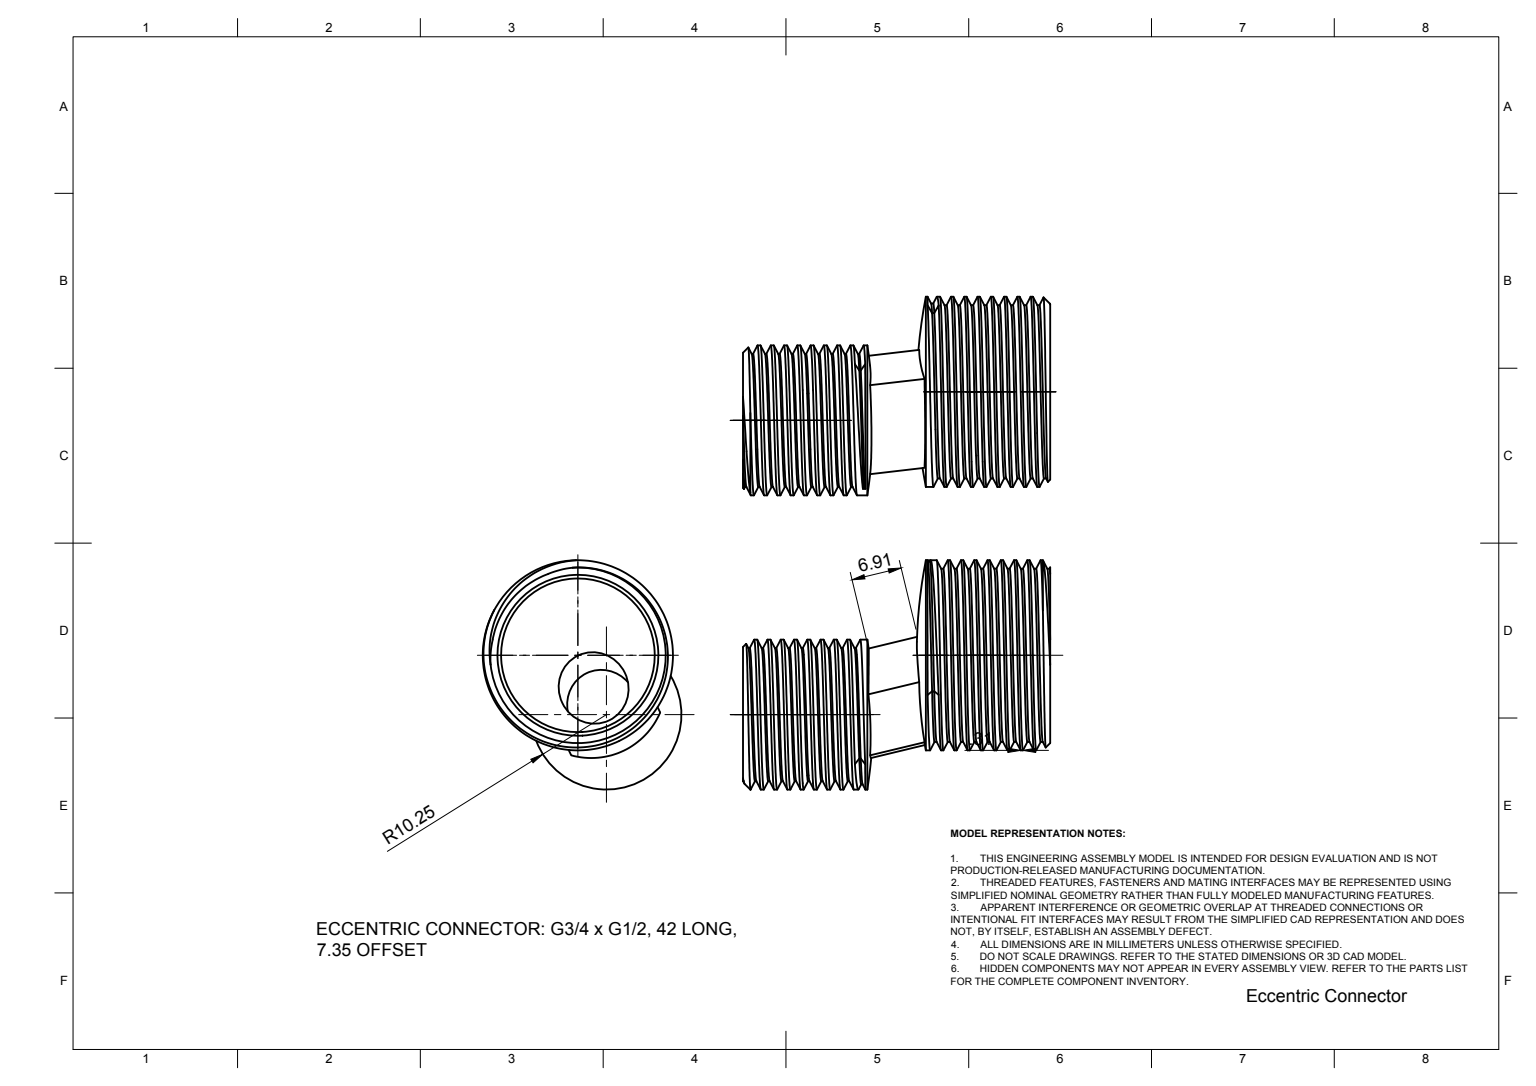
ISO-10303-21;
HEADER;
/* Generated by software containing ST-Developer
 * from STEP Tools, Inc. (www.steptools.com) 
 */

FILE_DESCRIPTION(
/* description */ ('STEP AP214'),
/* implementation_level */ '2;1');

FILE_NAME(
/* name */ 'Eccentric Connector.step',
/* time_stamp */ '2026-10-05T23:18:41-07:00',
/* author */ (''),
/* organization */ (''),
/* preprocessor_version */ 'ST-DEVELOPER v20.2',
/* originating_system */ 'Autodesk Translation Framework v15.15.0.0',
/* authorisation */ '');

FILE_SCHEMA (('AUTOMOTIVE_DESIGN { 1 0 10303 214 3 1 1 }'));
ENDSEC;

DATA;
#10=MECHANICAL_DESIGN_GEOMETRIC_PRESENTATION_REPRESENTATION('',(#112),#221662);
#73=MANIFOLD_SOLID_BREP('Body1',#79335);
#86=SHAPE_REPRESENTATION_RELATIONSHIP('SRR','None',#221721,#99);
#99=ADVANCED_BREP_SHAPE_REPRESENTATION('',(#73),#221661);
#112=STYLED_ITEM('',(#221783),#73);
#226=B_SPLINE_SURFACE_WITH_KNOTS('',3,3,((#217794,#217795,#217796,#217797,
#217798,#217799,#217800),(#217801,#217802,#217803,#217804,#217805,#217806,
#217807),(#217808,#217809,#217810,#217811,#217812,#217813,#217814),(#217815,
#217816,#217817,#217818,#217819,#217820,#217821)),.UNSPECIFIED.,.F.,.F.,
 .F.,(4,4),(4,1,1,1,4),(0.,1.),(0.,0.25,0.5,0.75,1.),.UNSPECIFIED.);
#227=B_SPLINE_SURFACE_WITH_KNOTS('',3,3,((#217858,#217859,#217860,#217861,
#217862,#217863,#217864,#217865,#217866,#217867,#217868,#217869,#217870,
#217871,#217872,#217873,#217874,#217875,#217876,#217877,#217878,#217879,
#217880,#217881,#217882,#217883,#217884,#217885,#217886,#217887,#217888,
#217889,#217890,#217891,#217892,#217893,#217894,#217895,#217896,#217897,
#217898,#217899,#217900,#217901,#217902,#217903,#217904,#217905,#217906,
#217907,#217908,#217909,#217910,#217911,#217912,#217913,#217914,#217915,
#217916,#217917,#217918,#217919,#217920,#217921,#217922,#217923,#217924),
(#217925,#217926,#217927,#217928,#217929,#217930,#217931,#217932,#217933,
#217934,#217935,#217936,#217937,#217938,#217939,#217940,#217941,#217942,
#217943,#217944,#217945,#217946,#217947,#217948,#217949,#217950,#217951,
#217952,#217953,#217954,#217955,#217956,#217957,#217958,#217959,#217960,
#217961,#217962,#217963,#217964,#217965,#217966,#217967,#217968,#217969,
#217970,#217971,#217972,#217973,#217974,#217975,#217976,#217977,#217978,
#217979,#217980,#217981,#217982,#217983,#217984,#217985,#217986,#217987,
#217988,#217989,#217990,#217991),(#217992,#217993,#217994,#217995,#217996,
#217997,#217998,#217999,#218000,#218001,#218002,#218003,#218004,#218005,
#218006,#218007,#218008,#218009,#218010,#218011,#218012,#218013,#218014,
#218015,#218016,#218017,#218018,#218019,#218020,#218021,#218022,#218023,
#218024,#218025,#218026,#218027,#218028,#218029,#218030,#218031,#218032,
#218033,#218034,#218035,#218036,#218037,#218038,#218039,#218040,#218041,
#218042,#218043,#218044,#218045,#218046,#218047,#218048,#218049,#218050,
#218051,#218052,#218053,#218054,#218055,#218056,#218057,#218058),(#218059,
#218060,#218061,#218062,#218063,#218064,#218065,#218066,#218067,#218068,
#218069,#218070,#218071,#218072,#218073,#218074,#218075,#218076,#218077,
#218078,#218079,#218080,#218081,#218082,#218083,#218084,#218085,#218086,
#218087,#218088,#218089,#218090,#218091,#218092,#218093,#218094,#218095,
#218096,#218097,#218098,#218099,#218100,#218101,#218102,#218103,#218104,
#218105,#218106,#218107,#218108,#218109,#218110,#218111,#218112,#218113,
#218114,#218115,#218116,#218117,#218118,#218119,#218120,#218121,#218122,
#218123,#218124,#218125)),.UNSPECIFIED.,.F.,.F.,.F.,(4,4),(4,1,1,1,1,1,
1,1,1,1,1,1,1,1,1,1,1,1,1,1,1,1,1,1,1,1,1,1,1,1,1,1,1,1,1,1,1,1,1,1,1,1,
1,1,1,1,1,1,1,1,1,1,1,1,1,1,1,1,1,1,1,1,1,1,4),(0.,1.),(0.,0.0156250000000022,
0.0312500000000006,0.0468750000000009,0.0625000000000012,0.0781250000000015,
0.0937500000000018,0.109375000000002,0.124999999999983,0.140624999999983,
0.156249999999984,0.171874999999984,0.187499999999984,0.203124999999984,
0.218749999999985,0.234374999999986,0.249999999999986,0.265624999999986,
0.281249999999986,0.296874999999986,0.312499999999987,0.328124999999987,
0.343749999999987,0.359374999999987,0.374999999999988,0.390624999999988,
0.406249999999988,0.421874999999989,0.437499999999989,0.45312499999999,
0.46874999999999,0.48437499999999,0.49999999999999,0.515624999999991,0.531249999999991,
0.546874999999991,0.562499999999992,0.578124999999992,0.593749999999992,
0.609374999999993,0.624999999999993,0.640624999999993,0.65625,0.671875,
0.6875,0.703125,0.71875,0.734375,0.75,0.765625,0.78125,0.796875,0.8125,
0.828125,0.84375,0.859375,0.875,0.890625,0.90625,0.921875,0.9375,0.953125,
0.96875,0.984375,1.),.UNSPECIFIED.);
#228=B_SPLINE_SURFACE_WITH_KNOTS('',3,3,((#218167,#218168,#218169,#218170,
#218171,#218172,#218173,#218174,#218175,#218176,#218177,#218178,#218179,
#218180,#218181,#218182,#218183,#218184,#218185,#218186,#218187,#218188,
#218189,#218190,#218191,#218192,#218193,#218194,#218195,#218196,#218197,
#218198,#218199,#218200,#218201,#218202,#218203,#218204,#218205,#218206,
#218207,#218208,#218209,#218210,#218211,#218212,#218213,#218214,#218215,
#218216,#218217,#218218,#218219,#218220,#218221,#218222,#218223,#218224,
#218225,#218226,#218227,#218228,#218229,#218230,#218231,#218232,#218233),
(#218234,#218235,#218236,#218237,#218238,#218239,#218240,#218241,#218242,
#218243,#218244,#218245,#218246,#218247,#218248,#218249,#218250,#218251,
#218252,#218253,#218254,#218255,#218256,#218257,#218258,#218259,#218260,
#218261,#218262,#218263,#218264,#218265,#218266,#218267,#218268,#218269,
#218270,#218271,#218272,#218273,#218274,#218275,#218276,#218277,#218278,
#218279,#218280,#218281,#218282,#218283,#218284,#218285,#218286,#218287,
#218288,#218289,#218290,#218291,#218292,#218293,#218294,#218295,#218296,
#218297,#218298,#218299,#218300),(#218301,#218302,#218303,#218304,#218305,
#218306,#218307,#218308,#218309,#218310,#218311,#218312,#218313,#218314,
#218315,#218316,#218317,#218318,#218319,#218320,#218321,#218322,#218323,
#218324,#218325,#218326,#218327,#218328,#218329,#218330,#218331,#218332,
#218333,#218334,#218335,#218336,#218337,#218338,#218339,#218340,#218341,
#218342,#218343,#218344,#218345,#218346,#218347,#218348,#218349,#218350,
#218351,#218352,#218353,#218354,#218355,#218356,#218357,#218358,#218359,
#218360,#218361,#218362,#218363,#218364,#218365,#218366,#218367),(#218368,
#218369,#218370,#218371,#218372,#218373,#218374,#218375,#218376,#218377,
#218378,#218379,#218380,#218381,#218382,#218383,#218384,#218385,#218386,
#218387,#218388,#218389,#218390,#218391,#218392,#218393,#218394,#218395,
#218396,#218397,#218398,#218399,#218400,#218401,#218402,#218403,#218404,
#218405,#218406,#218407,#218408,#218409,#218410,#218411,#218412,#218413,
#218414,#218415,#218416,#218417,#218418,#218419,#218420,#218421,#218422,
#218423,#218424,#218425,#218426,#218427,#218428,#218429,#218430,#218431,
#218432,#218433,#218434)),.UNSPECIFIED.,.F.,.F.,.F.,(4,4),(4,1,1,1,1,1,
1,1,1,1,1,1,1,1,1,1,1,1,1,1,1,1,1,1,1,1,1,1,1,1,1,1,1,1,1,1,1,1,1,1,1,1,
1,1,1,1,1,1,1,1,1,1,1,1,1,1,1,1,1,1,1,1,1,1,4),(0.,1.),(0.,0.0156250000000031,
0.03125,0.046875,0.0625,0.078125,0.09375,0.109375,0.124999999999992,0.140624999999992,
0.156249999999992,0.171874999999992,0.187499999999992,0.203124999999992,
0.218749999999993,0.234374999999993,0.249999999999993,0.265624999999993,
0.281249999999993,0.296874999999993,0.312499999999993,0.328124999999993,
0.343749999999994,0.359374999999994,0.374999999999994,0.390624999999994,
0.406249999999994,0.421874999999994,0.437499999999994,0.453125,0.46875,
0.484375,0.5,0.515625,0.53125,0.546875,0.5625,0.578125,0.59375,0.609375,
0.625,0.640625,0.65625,0.671875,0.6875,0.703125,0.71875,0.734375,0.75,0.765625,
0.78125,0.796875,0.8125,0.828125,0.84375,0.859375,0.875,0.890625,0.90625,
0.921875,0.9375,0.953125,0.96875,0.984375,1.),.UNSPECIFIED.);
#229=B_SPLINE_SURFACE_WITH_KNOTS('',3,3,((#218441,#218442,#218443,#218444,
#218445,#218446,#218447),(#218448,#218449,#218450,#218451,#218452,#218453,
#218454),(#218455,#218456,#218457,#218458,#218459,#218460,#218461),(#218462,
#218463,#218464,#218465,#218466,#218467,#218468)),.UNSPECIFIED.,.F.,.F.,
 .F.,(4,4),(4,1,1,1,4),(0.,1.),(0.,0.250000000000029,0.500000000000019,
0.75000000000001,1.),.UNSPECIFIED.);
#230=B_SPLINE_SURFACE_WITH_KNOTS('',3,3,((#218482,#218483,#218484,#218485,
#218486,#218487,#218488),(#218489,#218490,#218491,#218492,#218493,#218494,
#218495),(#218496,#218497,#218498,#218499,#218500,#218501,#218502),(#218503,
#218504,#218505,#218506,#218507,#218508,#218509)),.UNSPECIFIED.,.F.,.F.,
 .F.,(4,4),(4,1,1,1,4),(0.,1.),(0.,0.25,0.5,0.75,1.),.UNSPECIFIED.);
#231=B_SPLINE_SURFACE_WITH_KNOTS('',3,3,((#218516,#218517,#218518,#218519,
#218520,#218521,#218522,#218523,#218524,#218525,#218526,#218527,#218528,
#218529,#218530,#218531,#218532,#218533,#218534,#218535,#218536,#218537,
#218538,#218539,#218540,#218541,#218542,#218543,#218544,#218545,#218546,
#218547,#218548,#218549,#218550,#218551,#218552,#218553,#218554,#218555,
#218556,#218557,#218558,#218559,#218560,#218561,#218562,#218563,#218564,
#218565,#218566,#218567,#218568,#218569,#218570,#218571,#218572,#218573,
#218574,#218575,#218576,#218577,#218578,#218579,#218580,#218581,#218582),
(#218583,#218584,#218585,#218586,#218587,#218588,#218589,#218590,#218591,
#218592,#218593,#218594,#218595,#218596,#218597,#218598,#218599,#218600,
#218601,#218602,#218603,#218604,#218605,#218606,#218607,#218608,#218609,
#218610,#218611,#218612,#218613,#218614,#218615,#218616,#218617,#218618,
#218619,#218620,#218621,#218622,#218623,#218624,#218625,#218626,#218627,
#218628,#218629,#218630,#218631,#218632,#218633,#218634,#218635,#218636,
#218637,#218638,#218639,#218640,#218641,#218642,#218643,#218644,#218645,
#218646,#218647,#218648,#218649),(#218650,#218651,#218652,#218653,#218654,
#218655,#218656,#218657,#218658,#218659,#218660,#218661,#218662,#218663,
#218664,#218665,#218666,#218667,#218668,#218669,#218670,#218671,#218672,
#218673,#218674,#218675,#218676,#218677,#218678,#218679,#218680,#218681,
#218682,#218683,#218684,#218685,#218686,#218687,#218688,#218689,#218690,
#218691,#218692,#218693,#218694,#218695,#218696,#218697,#218698,#218699,
#218700,#218701,#218702,#218703,#218704,#218705,#218706,#218707,#218708,
#218709,#218710,#218711,#218712,#218713,#218714,#218715,#218716),(#218717,
#218718,#218719,#218720,#218721,#218722,#218723,#218724,#218725,#218726,
#218727,#218728,#218729,#218730,#218731,#218732,#218733,#218734,#218735,
#218736,#218737,#218738,#218739,#218740,#218741,#218742,#218743,#218744,
#218745,#218746,#218747,#218748,#218749,#218750,#218751,#218752,#218753,
#218754,#218755,#218756,#218757,#218758,#218759,#218760,#218761,#218762,
#218763,#218764,#218765,#218766,#218767,#218768,#218769,#218770,#218771,
#218772,#218773,#218774,#218775,#218776,#218777,#218778,#218779,#218780,
#218781,#218782,#218783)),.UNSPECIFIED.,.F.,.F.,.F.,(4,4),(4,1,1,1,1,1,
1,1,1,1,1,1,1,1,1,1,1,1,1,1,1,1,1,1,1,1,1,1,1,1,1,1,1,1,1,1,1,1,1,1,1,1,
1,1,1,1,1,1,1,1,1,1,1,1,1,1,1,1,1,1,1,1,1,1,4),(0.,1.),(0.,0.0156250000000031,
0.03125,0.046875,0.0625,0.078125,0.09375,0.109375,0.124999999999992,0.140624999999992,
0.156249999999992,0.171874999999992,0.187499999999992,0.203124999999992,
0.218749999999993,0.234374999999993,0.249999999999993,0.265624999999993,
0.281249999999993,0.296874999999993,0.312499999999993,0.328124999999993,
0.343749999999994,0.359374999999994,0.374999999999994,0.390624999999994,
0.406249999999994,0.421874999999994,0.437499999999994,0.453125,0.46875,
0.484375,0.5,0.515625,0.53125,0.546875,0.5625,0.578125,0.59375,0.609375,
0.625,0.640625,0.65625,0.671875,0.6875,0.703125,0.71875,0.734375,0.75,0.765625,
0.78125,0.796875,0.8125,0.828125,0.84375,0.859375,0.875,0.890625,0.90625,
0.921875,0.9375,0.953125,0.96875,0.984375,1.),.UNSPECIFIED.);
#232=B_SPLINE_SURFACE_WITH_KNOTS('',3,3,((#218785,#218786,#218787,#218788,
#218789,#218790,#218791,#218792,#218793,#218794,#218795,#218796,#218797,
#218798,#218799,#218800,#218801,#218802,#218803,#218804,#218805,#218806,
#218807,#218808,#218809,#218810,#218811,#218812,#218813,#218814,#218815,
#218816,#218817,#218818,#218819,#218820,#218821,#218822,#218823,#218824,
#218825,#218826,#218827,#218828,#218829,#218830,#218831,#218832,#218833,
#218834,#218835,#218836,#218837,#218838,#218839,#218840,#218841,#218842,
#218843,#218844,#218845,#218846,#218847,#218848,#218849,#218850,#218851),
(#218852,#218853,#218854,#218855,#218856,#218857,#218858,#218859,#218860,
#218861,#218862,#218863,#218864,#218865,#218866,#218867,#218868,#218869,
#218870,#218871,#218872,#218873,#218874,#218875,#218876,#218877,#218878,
#218879,#218880,#218881,#218882,#218883,#218884,#218885,#218886,#218887,
#218888,#218889,#218890,#218891,#218892,#218893,#218894,#218895,#218896,
#218897,#218898,#218899,#218900,#218901,#218902,#218903,#218904,#218905,
#218906,#218907,#218908,#218909,#218910,#218911,#218912,#218913,#218914,
#218915,#218916,#218917,#218918),(#218919,#218920,#218921,#218922,#218923,
#218924,#218925,#218926,#218927,#218928,#218929,#218930,#218931,#218932,
#218933,#218934,#218935,#218936,#218937,#218938,#218939,#218940,#218941,
#218942,#218943,#218944,#218945,#218946,#218947,#218948,#218949,#218950,
#218951,#218952,#218953,#218954,#218955,#218956,#218957,#218958,#218959,
#218960,#218961,#218962,#218963,#218964,#218965,#218966,#218967,#218968,
#218969,#218970,#218971,#218972,#218973,#218974,#218975,#218976,#218977,
#218978,#218979,#218980,#218981,#218982,#218983,#218984,#218985),(#218986,
#218987,#218988,#218989,#218990,#218991,#218992,#218993,#218994,#218995,
#218996,#218997,#218998,#218999,#219000,#219001,#219002,#219003,#219004,
#219005,#219006,#219007,#219008,#219009,#219010,#219011,#219012,#219013,
#219014,#219015,#219016,#219017,#219018,#219019,#219020,#219021,#219022,
#219023,#219024,#219025,#219026,#219027,#219028,#219029,#219030,#219031,
#219032,#219033,#219034,#219035,#219036,#219037,#219038,#219039,#219040,
#219041,#219042,#219043,#219044,#219045,#219046,#219047,#219048,#219049,
#219050,#219051,#219052)),.UNSPECIFIED.,.F.,.F.,.F.,(4,4),(4,1,1,1,1,1,
1,1,1,1,1,1,1,1,1,1,1,1,1,1,1,1,1,1,1,1,1,1,1,1,1,1,1,1,1,1,1,1,1,1,1,1,
1,1,1,1,1,1,1,1,1,1,1,1,1,1,1,1,1,1,1,1,1,1,4),(0.,1.),(0.,0.0156250000000022,
0.0312500000000006,0.0468750000000009,0.0625000000000012,0.0781250000000015,
0.0937500000000018,0.109375000000002,0.124999999999983,0.140624999999983,
0.156249999999984,0.171874999999984,0.187499999999984,0.203124999999984,
0.218749999999985,0.234374999999986,0.249999999999986,0.265624999999986,
0.281249999999986,0.296874999999986,0.312499999999987,0.328124999999987,
0.343749999999987,0.359374999999987,0.374999999999988,0.390624999999988,
0.406249999999988,0.421874999999989,0.437499999999989,0.45312499999999,
0.46874999999999,0.48437499999999,0.49999999999999,0.515624999999991,0.531249999999991,
0.546874999999991,0.562499999999992,0.578124999999992,0.593749999999992,
0.609374999999993,0.624999999999993,0.640624999999993,0.65625,0.671875,
0.6875,0.703125,0.71875,0.734375,0.75,0.765625,0.78125,0.796875,0.8125,
0.828125,0.84375,0.859375,0.875,0.890625,0.90625,0.921875,0.9375,0.953125,
0.96875,0.984375,1.),.UNSPECIFIED.);
#233=B_SPLINE_SURFACE_WITH_KNOTS('',3,3,((#219054,#219055,#219056,#219057,
#219058,#219059,#219060,#219061,#219062,#219063,#219064,#219065,#219066,
#219067,#219068,#219069,#219070,#219071,#219072),(#219073,#219074,#219075,
#219076,#219077,#219078,#219079,#219080,#219081,#219082,#219083,#219084,
#219085,#219086,#219087,#219088,#219089,#219090,#219091),(#219092,#219093,
#219094,#219095,#219096,#219097,#219098,#219099,#219100,#219101,#219102,
#219103,#219104,#219105,#219106,#219107,#219108,#219109,#219110),(#219111,
#219112,#219113,#219114,#219115,#219116,#219117,#219118,#219119,#219120,
#219121,#219122,#219123,#219124,#219125,#219126,#219127,#219128,#219129)),
 .UNSPECIFIED.,.F.,.F.,.F.,(4,4),(4,1,1,1,1,1,1,1,1,1,1,1,1,1,1,1,4),(0.,
1.),(0.,0.0624999999999738,0.124999999999948,0.187499999999503,0.249999999999477,
0.312499999999451,0.374999999999424,0.437499999999398,0.499999999999372,
0.562499999999346,0.62499999999932,0.687499999998875,0.749999999998849,
0.812499999998822,0.874999999998796,0.93749999999877,1.),.UNSPECIFIED.);
#234=B_SPLINE_SURFACE_WITH_KNOTS('',3,3,((#219171,#219172,#219173,#219174,
#219175,#219176,#219177),(#219178,#219179,#219180,#219181,#219182,#219183,
#219184),(#219185,#219186,#219187,#219188,#219189,#219190,#219191),(#219192,
#219193,#219194,#219195,#219196,#219197,#219198)),.UNSPECIFIED.,.F.,.F.,
 .F.,(4,4),(4,1,1,1,4),(0.,1.),(0.,0.25,0.5,0.75,1.),.UNSPECIFIED.);
#235=B_SPLINE_SURFACE_WITH_KNOTS('',3,3,((#219235,#219236,#219237,#219238,
#219239,#219240,#219241,#219242,#219243,#219244,#219245,#219246,#219247,
#219248,#219249,#219250,#219251,#219252,#219253,#219254,#219255,#219256,
#219257,#219258,#219259,#219260,#219261,#219262,#219263,#219264,#219265,
#219266,#219267,#219268,#219269),(#219270,#219271,#219272,#219273,#219274,
#219275,#219276,#219277,#219278,#219279,#219280,#219281,#219282,#219283,
#219284,#219285,#219286,#219287,#219288,#219289,#219290,#219291,#219292,
#219293,#219294,#219295,#219296,#219297,#219298,#219299,#219300,#219301,
#219302,#219303,#219304),(#219305,#219306,#219307,#219308,#219309,#219310,
#219311,#219312,#219313,#219314,#219315,#219316,#219317,#219318,#219319,
#219320,#219321,#219322,#219323,#219324,#219325,#219326,#219327,#219328,
#219329,#219330,#219331,#219332,#219333,#219334,#219335,#219336,#219337,
#219338,#219339),(#219340,#219341,#219342,#219343,#219344,#219345,#219346,
#219347,#219348,#219349,#219350,#219351,#219352,#219353,#219354,#219355,
#219356,#219357,#219358,#219359,#219360,#219361,#219362,#219363,#219364,
#219365,#219366,#219367,#219368,#219369,#219370,#219371,#219372,#219373,
#219374)),.UNSPECIFIED.,.F.,.F.,.F.,(4,4),(4,1,1,1,1,1,1,1,1,1,1,1,1,1,
1,1,1,1,1,1,1,1,1,1,1,1,1,1,1,1,1,1,4),(0.,1.),(0.,0.0312500000000088,0.0625000000000175,
0.0937500000000263,0.125000000000035,0.156250000000044,0.187500000000053,
0.218750000000062,0.25000000000007,0.281250000000078,0.312500000000087,
0.343750000000096,0.375000000000105,0.406250000000114,0.437500000000123,
0.468750000000131,0.50000000000014,0.531250000000149,0.562500000000157,
0.593750000000166,0.625000000000175,0.656250000000184,0.687500000000192,
0.718750000000201,0.75000000000021,0.781250000000079,0.812500000000087,
0.843750000000096,0.875000000000105,0.906250000000114,0.937500000000122,
0.968750000000131,1.),.UNSPECIFIED.);
#236=B_SPLINE_SURFACE_WITH_KNOTS('',3,3,((#219849,#219850,#219851,#219852,
#219853,#219854,#219855,#219856,#219857,#219858,#219859,#219860,#219861,
#219862,#219863,#219864,#219865,#219866,#219867,#219868,#219869,#219870,
#219871,#219872,#219873,#219874,#219875,#219876,#219877,#219878,#219879,
#219880,#219881,#219882,#219883,#219884,#219885,#219886,#219887,#219888,
#219889,#219890,#219891,#219892,#219893,#219894,#219895,#219896,#219897,
#219898,#219899,#219900,#219901,#219902,#219903,#219904,#219905,#219906,
#219907,#219908,#219909,#219910,#219911,#219912,#219913,#219914,#219915),
(#219916,#219917,#219918,#219919,#219920,#219921,#219922,#219923,#219924,
#219925,#219926,#219927,#219928,#219929,#219930,#219931,#219932,#219933,
#219934,#219935,#219936,#219937,#219938,#219939,#219940,#219941,#219942,
#219943,#219944,#219945,#219946,#219947,#219948,#219949,#219950,#219951,
#219952,#219953,#219954,#219955,#219956,#219957,#219958,#219959,#219960,
#219961,#219962,#219963,#219964,#219965,#219966,#219967,#219968,#219969,
#219970,#219971,#219972,#219973,#219974,#219975,#219976,#219977,#219978,
#219979,#219980,#219981,#219982),(#219983,#219984,#219985,#219986,#219987,
#219988,#219989,#219990,#219991,#219992,#219993,#219994,#219995,#219996,
#219997,#219998,#219999,#220000,#220001,#220002,#220003,#220004,#220005,
#220006,#220007,#220008,#220009,#220010,#220011,#220012,#220013,#220014,
#220015,#220016,#220017,#220018,#220019,#220020,#220021,#220022,#220023,
#220024,#220025,#220026,#220027,#220028,#220029,#220030,#220031,#220032,
#220033,#220034,#220035,#220036,#220037,#220038,#220039,#220040,#220041,
#220042,#220043,#220044,#220045,#220046,#220047,#220048,#220049),(#220050,
#220051,#220052,#220053,#220054,#220055,#220056,#220057,#220058,#220059,
#220060,#220061,#220062,#220063,#220064,#220065,#220066,#220067,#220068,
#220069,#220070,#220071,#220072,#220073,#220074,#220075,#220076,#220077,
#220078,#220079,#220080,#220081,#220082,#220083,#220084,#220085,#220086,
#220087,#220088,#220089,#220090,#220091,#220092,#220093,#220094,#220095,
#220096,#220097,#220098,#220099,#220100,#220101,#220102,#220103,#220104,
#220105,#220106,#220107,#220108,#220109,#220110,#220111,#220112,#220113,
#220114,#220115,#220116)),.UNSPECIFIED.,.F.,.F.,.F.,(4,4),(4,1,1,1,1,1,
1,1,1,1,1,1,1,1,1,1,1,1,1,1,1,1,1,1,1,1,1,1,1,1,1,1,1,1,1,1,1,1,1,1,1,1,
1,1,1,1,1,1,1,1,1,1,1,1,1,1,1,1,1,1,1,1,1,1,4),(0.,1.),(0.,0.015625,0.03125,
0.046875,0.0625,0.078125,0.09375,0.109375,0.125,0.140625,0.15625,0.171875,
0.1875,0.203125,0.21875,0.234375,0.25,0.265625,0.28125,0.296875,0.3125,
0.328125,0.34375,0.359375,0.375,0.390625,0.40625,0.421875,0.4375,0.453125,
0.46875,0.484375,0.5,0.515625,0.53125,0.546875,0.5625,0.578125,0.59375,
0.609375,0.625,0.640625,0.65625,0.671875,0.6875,0.703125,0.71875,0.734375,
0.75,0.765625,0.78125,0.796875,0.8125,0.828125,0.84375,0.859375,0.875,0.890625,
0.90625,0.921875,0.9375,0.953125,0.96875,0.984375,1.),.UNSPECIFIED.);
#237=B_SPLINE_SURFACE_WITH_KNOTS('',3,3,((#220185,#220186,#220187,#220188,
#220189,#220190,#220191),(#220192,#220193,#220194,#220195,#220196,#220197,
#220198),(#220199,#220200,#220201,#220202,#220203,#220204,#220205),(#220206,
#220207,#220208,#220209,#220210,#220211,#220212)),.UNSPECIFIED.,.F.,.F.,
 .F.,(4,4),(4,1,1,1,4),(0.,1.),(0.,0.250000000000007,0.5,0.75,1.),
 .UNSPECIFIED.);
#238=B_SPLINE_SURFACE_WITH_KNOTS('',3,3,((#220240,#220241,#220242,#220243,
#220244,#220245,#220246),(#220247,#220248,#220249,#220250,#220251,#220252,
#220253),(#220254,#220255,#220256,#220257,#220258,#220259,#220260),(#220261,
#220262,#220263,#220264,#220265,#220266,#220267)),.UNSPECIFIED.,.F.,.F.,
 .F.,(4,4),(4,1,1,1,4),(0.,1.),(0.,0.25,0.5,0.75,1.),.UNSPECIFIED.);
#239=B_SPLINE_SURFACE_WITH_KNOTS('',3,3,((#220274,#220275,#220276,#220277,
#220278,#220279,#220280,#220281,#220282,#220283,#220284,#220285,#220286,
#220287,#220288,#220289,#220290,#220291,#220292,#220293,#220294,#220295,
#220296,#220297,#220298,#220299,#220300,#220301,#220302,#220303,#220304,
#220305,#220306,#220307,#220308,#220309,#220310,#220311,#220312,#220313,
#220314,#220315,#220316,#220317,#220318,#220319,#220320,#220321,#220322,
#220323,#220324,#220325,#220326,#220327,#220328,#220329,#220330,#220331,
#220332,#220333,#220334,#220335,#220336,#220337,#220338,#220339,#220340),
(#220341,#220342,#220343,#220344,#220345,#220346,#220347,#220348,#220349,
#220350,#220351,#220352,#220353,#220354,#220355,#220356,#220357,#220358,
#220359,#220360,#220361,#220362,#220363,#220364,#220365,#220366,#220367,
#220368,#220369,#220370,#220371,#220372,#220373,#220374,#220375,#220376,
#220377,#220378,#220379,#220380,#220381,#220382,#220383,#220384,#220385,
#220386,#220387,#220388,#220389,#220390,#220391,#220392,#220393,#220394,
#220395,#220396,#220397,#220398,#220399,#220400,#220401,#220402,#220403,
#220404,#220405,#220406,#220407),(#220408,#220409,#220410,#220411,#220412,
#220413,#220414,#220415,#220416,#220417,#220418,#220419,#220420,#220421,
#220422,#220423,#220424,#220425,#220426,#220427,#220428,#220429,#220430,
#220431,#220432,#220433,#220434,#220435,#220436,#220437,#220438,#220439,
#220440,#220441,#220442,#220443,#220444,#220445,#220446,#220447,#220448,
#220449,#220450,#220451,#220452,#220453,#220454,#220455,#220456,#220457,
#220458,#220459,#220460,#220461,#220462,#220463,#220464,#220465,#220466,
#220467,#220468,#220469,#220470,#220471,#220472,#220473,#220474),(#220475,
#220476,#220477,#220478,#220479,#220480,#220481,#220482,#220483,#220484,
#220485,#220486,#220487,#220488,#220489,#220490,#220491,#220492,#220493,
#220494,#220495,#220496,#220497,#220498,#220499,#220500,#220501,#220502,
#220503,#220504,#220505,#220506,#220507,#220508,#220509,#220510,#220511,
#220512,#220513,#220514,#220515,#220516,#220517,#220518,#220519,#220520,
#220521,#220522,#220523,#220524,#220525,#220526,#220527,#220528,#220529,
#220530,#220531,#220532,#220533,#220534,#220535,#220536,#220537,#220538,
#220539,#220540,#220541)),.UNSPECIFIED.,.F.,.F.,.F.,(4,4),(4,1,1,1,1,1,
1,1,1,1,1,1,1,1,1,1,1,1,1,1,1,1,1,1,1,1,1,1,1,1,1,1,1,1,1,1,1,1,1,1,1,1,
1,1,1,1,1,1,1,1,1,1,1,1,1,1,1,1,1,1,1,1,1,1,4),(0.,1.),(0.,0.015625,0.03125,
0.046875,0.0625,0.078125,0.09375,0.109375,0.125,0.140625,0.15625,0.171875,
0.1875,0.203125,0.21875,0.234375,0.25,0.265625,0.28125,0.296875,0.3125,
0.328125,0.34375,0.359375,0.375,0.390625,0.40625,0.421875,0.4375,0.453125,
0.46875,0.484375,0.5,0.515625,0.53125,0.546875,0.5625,0.578125,0.59375,
0.609375,0.625,0.640625,0.65625,0.671875,0.6875,0.703125,0.71875,0.734375,
0.75,0.765625,0.78125,0.796875,0.8125,0.828125,0.84375,0.859375,0.875,0.890625,
0.90625,0.921875,0.9375,0.953125,0.96875,0.984375,1.),.UNSPECIFIED.);
#240=B_SPLINE_SURFACE_WITH_KNOTS('',3,3,((#220621,#220622,#220623,#220624,
#220625,#220626,#220627,#220628,#220629,#220630,#220631,#220632,#220633,
#220634,#220635,#220636,#220637,#220638,#220639,#220640,#220641,#220642,
#220643,#220644,#220645,#220646,#220647,#220648,#220649,#220650,#220651,
#220652,#220653,#220654,#220655,#220656,#220657,#220658,#220659,#220660,
#220661,#220662,#220663,#220664,#220665,#220666,#220667,#220668,#220669,
#220670,#220671,#220672,#220673,#220674,#220675,#220676,#220677,#220678,
#220679,#220680,#220681,#220682,#220683,#220684,#220685,#220686,#220687),
(#220688,#220689,#220690,#220691,#220692,#220693,#220694,#220695,#220696,
#220697,#220698,#220699,#220700,#220701,#220702,#220703,#220704,#220705,
#220706,#220707,#220708,#220709,#220710,#220711,#220712,#220713,#220714,
#220715,#220716,#220717,#220718,#220719,#220720,#220721,#220722,#220723,
#220724,#220725,#220726,#220727,#220728,#220729,#220730,#220731,#220732,
#220733,#220734,#220735,#220736,#220737,#220738,#220739,#220740,#220741,
#220742,#220743,#220744,#220745,#220746,#220747,#220748,#220749,#220750,
#220751,#220752,#220753,#220754),(#220755,#220756,#220757,#220758,#220759,
#220760,#220761,#220762,#220763,#220764,#220765,#220766,#220767,#220768,
#220769,#220770,#220771,#220772,#220773,#220774,#220775,#220776,#220777,
#220778,#220779,#220780,#220781,#220782,#220783,#220784,#220785,#220786,
#220787,#220788,#220789,#220790,#220791,#220792,#220793,#220794,#220795,
#220796,#220797,#220798,#220799,#220800,#220801,#220802,#220803,#220804,
#220805,#220806,#220807,#220808,#220809,#220810,#220811,#220812,#220813,
#220814,#220815,#220816,#220817,#220818,#220819,#220820,#220821),(#220822,
#220823,#220824,#220825,#220826,#220827,#220828,#220829,#220830,#220831,
#220832,#220833,#220834,#220835,#220836,#220837,#220838,#220839,#220840,
#220841,#220842,#220843,#220844,#220845,#220846,#220847,#220848,#220849,
#220850,#220851,#220852,#220853,#220854,#220855,#220856,#220857,#220858,
#220859,#220860,#220861,#220862,#220863,#220864,#220865,#220866,#220867,
#220868,#220869,#220870,#220871,#220872,#220873,#220874,#220875,#220876,
#220877,#220878,#220879,#220880,#220881,#220882,#220883,#220884,#220885,
#220886,#220887,#220888)),.UNSPECIFIED.,.F.,.F.,.F.,(4,4),(4,1,1,1,1,1,
1,1,1,1,1,1,1,1,1,1,1,1,1,1,1,1,1,1,1,1,1,1,1,1,1,1,1,1,1,1,1,1,1,1,1,1,
1,1,1,1,1,1,1,1,1,1,1,1,1,1,1,1,1,1,1,1,1,1,4),(0.,1.),(0.,0.015625,0.03125,
0.046875,0.0625,0.078125,0.09375,0.109375,0.125,0.140625,0.15625,0.171875,
0.1875,0.203125,0.21875,0.234375,0.25,0.265625,0.28125,0.296875,0.3125,
0.328125,0.34375,0.359375,0.375,0.390625,0.40625,0.421875,0.4375,0.453125,
0.46875,0.484375,0.5,0.515625,0.53125,0.546875,0.5625,0.578125,0.59375,
0.609375,0.625,0.640625,0.65625,0.671875,0.6875,0.703125,0.71875,0.734375,
0.75,0.765625,0.78125,0.796875,0.8125,0.828125,0.84375,0.859375,0.875,0.890625,
0.90625,0.921875,0.9375,0.953125,0.96875,0.984375,1.),.UNSPECIFIED.);
#241=B_SPLINE_SURFACE_WITH_KNOTS('',3,3,((#220890,#220891,#220892,#220893,
#220894,#220895,#220896,#220897,#220898,#220899,#220900,#220901,#220902,
#220903,#220904,#220905,#220906,#220907,#220908,#220909,#220910,#220911,
#220912,#220913,#220914,#220915,#220916,#220917,#220918,#220919,#220920,
#220921,#220922,#220923,#220924),(#220925,#220926,#220927,#220928,#220929,
#220930,#220931,#220932,#220933,#220934,#220935,#220936,#220937,#220938,
#220939,#220940,#220941,#220942,#220943,#220944,#220945,#220946,#220947,
#220948,#220949,#220950,#220951,#220952,#220953,#220954,#220955,#220956,
#220957,#220958,#220959),(#220960,#220961,#220962,#220963,#220964,#220965,
#220966,#220967,#220968,#220969,#220970,#220971,#220972,#220973,#220974,
#220975,#220976,#220977,#220978,#220979,#220980,#220981,#220982,#220983,
#220984,#220985,#220986,#220987,#220988,#220989,#220990,#220991,#220992,
#220993,#220994),(#220995,#220996,#220997,#220998,#220999,#221000,#221001,
#221002,#221003,#221004,#221005,#221006,#221007,#221008,#221009,#221010,
#221011,#221012,#221013,#221014,#221015,#221016,#221017,#221018,#221019,
#221020,#221021,#221022,#221023,#221024,#221025,#221026,#221027,#221028,
#221029)),.UNSPECIFIED.,.F.,.F.,.F.,(4,4),(4,1,1,1,1,1,1,1,1,1,1,1,1,1,
1,1,1,1,1,1,1,1,1,1,1,1,1,1,1,1,1,1,4),(0.,1.),(0.,0.0312499999999743,0.0624999999999486,
0.0937499999999229,0.125000000000034,0.156250000000008,0.187499999999983,
0.218749999999957,0.249999999999932,0.281250000000043,0.312500000000017,
0.343749999999991,0.374999999999966,0.406250000000077,0.437500000000052,
0.468750000000026,0.5,0.531249999999974,0.562500000000086,0.59375000000006,
0.625000000000034,0.656250000000009,0.687499999999983,0.718750000000095,
0.750000000000069,0.781250000000043,0.812500000000017,0.843750000000129,
0.875000000000103,0.906250000000077,0.937500000000052,0.968750000000026,
1.),.UNSPECIFIED.);
#242=B_SPLINE_SURFACE_WITH_KNOTS('',3,3,((#221042,#221043,#221044,#221045,
#221046,#221047,#221048,#221049,#221050,#221051,#221052,#221053,#221054,
#221055,#221056,#221057,#221058,#221059,#221060,#221061,#221062,#221063,
#221064,#221065,#221066,#221067,#221068,#221069,#221070,#221071,#221072,
#221073,#221074,#221075,#221076,#221077,#221078,#221079,#221080,#221081,
#221082,#221083,#221084,#221085,#221086,#221087,#221088,#221089,#221090,
#221091,#221092,#221093,#221094,#221095,#221096,#221097,#221098,#221099,
#221100,#221101,#221102,#221103,#221104,#221105,#221106,#221107,#221108),
(#221109,#221110,#221111,#221112,#221113,#221114,#221115,#221116,#221117,
#221118,#221119,#221120,#221121,#221122,#221123,#221124,#221125,#221126,
#221127,#221128,#221129,#221130,#221131,#221132,#221133,#221134,#221135,
#221136,#221137,#221138,#221139,#221140,#221141,#221142,#221143,#221144,
#221145,#221146,#221147,#221148,#221149,#221150,#221151,#221152,#221153,
#221154,#221155,#221156,#221157,#221158,#221159,#221160,#221161,#221162,
#221163,#221164,#221165,#221166,#221167,#221168,#221169,#221170,#221171,
#221172,#221173,#221174,#221175),(#221176,#221177,#221178,#221179,#221180,
#221181,#221182,#221183,#221184,#221185,#221186,#221187,#221188,#221189,
#221190,#221191,#221192,#221193,#221194,#221195,#221196,#221197,#221198,
#221199,#221200,#221201,#221202,#221203,#221204,#221205,#221206,#221207,
#221208,#221209,#221210,#221211,#221212,#221213,#221214,#221215,#221216,
#221217,#221218,#221219,#221220,#221221,#221222,#221223,#221224,#221225,
#221226,#221227,#221228,#221229,#221230,#221231,#221232,#221233,#221234,
#221235,#221236,#221237,#221238,#221239,#221240,#221241,#221242),(#221243,
#221244,#221245,#221246,#221247,#221248,#221249,#221250,#221251,#221252,
#221253,#221254,#221255,#221256,#221257,#221258,#221259,#221260,#221261,
#221262,#221263,#221264,#221265,#221266,#221267,#221268,#221269,#221270,
#221271,#221272,#221273,#221274,#221275,#221276,#221277,#221278,#221279,
#221280,#221281,#221282,#221283,#221284,#221285,#221286,#221287,#221288,
#221289,#221290,#221291,#221292,#221293,#221294,#221295,#221296,#221297,
#221298,#221299,#221300,#221301,#221302,#221303,#221304,#221305,#221306,
#221307,#221308,#221309)),.UNSPECIFIED.,.F.,.F.,.F.,(4,4),(4,1,1,1,1,1,
1,1,1,1,1,1,1,1,1,1,1,1,1,1,1,1,1,1,1,1,1,1,1,1,1,1,1,1,1,1,1,1,1,1,1,1,
1,1,1,1,1,1,1,1,1,1,1,1,1,1,1,1,1,1,1,1,1,1,4),(0.,1.),(0.,0.015625,0.03125,
0.046875,0.0625,0.078125,0.09375,0.109375,0.125,0.140625,0.15625,0.171875,
0.1875,0.203125,0.21875,0.234375,0.25,0.265625,0.28125,0.296875,0.3125,
0.328125,0.34375,0.359375,0.375,0.390625,0.40625,0.421875,0.4375,0.453125,
0.46875,0.484375,0.5,0.515625,0.53125,0.546875,0.5625,0.578125,0.59375,
0.609375,0.625,0.640625,0.65625,0.671875,0.6875,0.703125,0.71875,0.734375,
0.75,0.765625,0.78125,0.796875,0.8125,0.828125,0.84375,0.859375,0.875,0.890625,
0.90625,0.921875,0.9375,0.953125,0.96875,0.984375,1.),.UNSPECIFIED.);
#243=B_SPLINE_SURFACE_WITH_KNOTS('',3,3,((#221311,#221312,#221313,#221314,
#221315,#221316,#221317,#221318,#221319,#221320,#221321,#221322,#221323,
#221324,#221325,#221326,#221327,#221328,#221329,#221330,#221331,#221332,
#221333,#221334,#221335,#221336,#221337,#221338,#221339,#221340,#221341,
#221342,#221343,#221344,#221345),(#221346,#221347,#221348,#221349,#221350,
#221351,#221352,#221353,#221354,#221355,#221356,#221357,#221358,#221359,
#221360,#221361,#221362,#221363,#221364,#221365,#221366,#221367,#221368,
#221369,#221370,#221371,#221372,#221373,#221374,#221375,#221376,#221377,
#221378,#221379,#221380),(#221381,#221382,#221383,#221384,#221385,#221386,
#221387,#221388,#221389,#221390,#221391,#221392,#221393,#221394,#221395,
#221396,#221397,#221398,#221399,#221400,#221401,#221402,#221403,#221404,
#221405,#221406,#221407,#221408,#221409,#221410,#221411,#221412,#221413,
#221414,#221415),(#221416,#221417,#221418,#221419,#221420,#221421,#221422,
#221423,#221424,#221425,#221426,#221427,#221428,#221429,#221430,#221431,
#221432,#221433,#221434,#221435,#221436,#221437,#221438,#221439,#221440,
#221441,#221442,#221443,#221444,#221445,#221446,#221447,#221448,#221449,
#221450)),.UNSPECIFIED.,.F.,.F.,.F.,(4,4),(4,1,1,1,1,1,1,1,1,1,1,1,1,1,
1,1,1,1,1,1,1,1,1,1,1,1,1,1,1,1,1,1,4),(0.,1.),(0.,0.031249999999901,0.0624999999999529,
0.0937500000000048,0.125000000000057,0.156250000000109,0.187500000000009,
0.218750000000062,0.250000000000113,0.281250000000165,0.312500000000066,
0.343750000000118,0.37500000000017,0.406250000000221,0.437500000000123,
0.468750000000175,0.500000000000226,0.531250000000278,0.562500000000179,
0.593750000000231,0.625000000000283,0.656250000000335,0.687500000000236,
0.718750000000288,0.75000000000034,0.781250000000392,0.812500000000292,
0.843750000000344,0.875000000000396,0.906250000000448,0.937500000000349,
0.968750000000401,1.),.UNSPECIFIED.);
#244=B_SPLINE_SURFACE_WITH_KNOTS('',3,3,((#221527,#221528,#221529,#221530,
#221531,#221532,#221533,#221534,#221535,#221536,#221537,#221538,#221539,
#221540,#221541,#221542,#221543,#221544,#221545),(#221546,#221547,#221548,
#221549,#221550,#221551,#221552,#221553,#221554,#221555,#221556,#221557,
#221558,#221559,#221560,#221561,#221562,#221563,#221564),(#221565,#221566,
#221567,#221568,#221569,#221570,#221571,#221572,#221573,#221574,#221575,
#221576,#221577,#221578,#221579,#221580,#221581,#221582,#221583),(#221584,
#221585,#221586,#221587,#221588,#221589,#221590,#221591,#221592,#221593,
#221594,#221595,#221596,#221597,#221598,#221599,#221600,#221601,#221602)),
 .UNSPECIFIED.,.F.,.F.,.F.,(4,4),(4,1,1,1,1,1,1,1,1,1,1,1,1,1,1,1,4),(0.,
1.),(0.,0.0625,0.124999999999643,0.187499999999643,0.249999999999643,0.312499999999286,
0.374999999999286,0.437499999999286,0.499999999999286,0.562499999998929,
0.624999999998929,0.687499999998929,0.749999999998572,0.812499999998572,
0.874999999998572,0.937499999998572,1.),.UNSPECIFIED.);
#1725=FACE_BOUND('',#29373,.T.);
#1726=FACE_BOUND('',#29375,.T.);
#1727=FACE_BOUND('',#29377,.T.);
#1728=FACE_BOUND('',#29381,.T.);
#1969=CONICAL_SURFACE('',#86083,12.87032685775,0.785398346845167);
#1970=CONICAL_SURFACE('',#86103,9.75000242976401,0.785398331532869);
#1971=CONICAL_SURFACE('',#86106,9.75000242976401,0.785398331532869);
#1972=CONICAL_SURFACE('',#86127,12.87032685775,0.785398346845167);
#1973=CONICAL_SURFACE('',#86134,10.75000319972,0.785398446953936);
#1974=CONICAL_SURFACE('',#86142,7.999997663262,0.785397845123046);
#2344=CYLINDRICAL_SURFACE('',#86060,10.25);
#2345=CYLINDRICAL_SURFACE('',#86063,10.25);
#2346=CYLINDRICAL_SURFACE('',#86064,10.25);
#2347=CYLINDRICAL_SURFACE('',#86065,10.25);
#2348=CYLINDRICAL_SURFACE('',#86066,10.25);
#2349=CYLINDRICAL_SURFACE('',#86067,10.25);
#2350=CYLINDRICAL_SURFACE('',#86068,10.25);
#2351=CYLINDRICAL_SURFACE('',#86069,10.25);
#2352=CYLINDRICAL_SURFACE('',#86070,13.);
#2353=CYLINDRICAL_SURFACE('',#86072,13.);
#2354=CYLINDRICAL_SURFACE('',#86074,13.);
#2355=CYLINDRICAL_SURFACE('',#86075,13.);
#2356=CYLINDRICAL_SURFACE('',#86076,13.);
#2357=CYLINDRICAL_SURFACE('',#86077,13.);
#2358=CYLINDRICAL_SURFACE('',#86078,13.);
#2359=CYLINDRICAL_SURFACE('',#86079,13.);
#2360=CYLINDRICAL_SURFACE('',#86080,13.);
#2361=CYLINDRICAL_SURFACE('',#86085,9.09006752601109);
#2362=CYLINDRICAL_SURFACE('',#86086,9.09006752601109);
#2363=CYLINDRICAL_SURFACE('',#86087,9.09006752601109);
#2364=CYLINDRICAL_SURFACE('',#86088,9.09006752601109);
#2365=CYLINDRICAL_SURFACE('',#86089,9.0900675260086);
#2366=CYLINDRICAL_SURFACE('',#86090,9.0900675260086);
#2367=CYLINDRICAL_SURFACE('',#86091,9.0900675260086);
#2368=CYLINDRICAL_SURFACE('',#86092,9.0900675260086);
#2369=CYLINDRICAL_SURFACE('',#86093,9.08769033371916);
#2370=CYLINDRICAL_SURFACE('',#86095,11.8397710119949);
#2371=CYLINDRICAL_SURFACE('',#86097,11.8397710119949);
#2372=CYLINDRICAL_SURFACE('',#86098,11.8397710119949);
#2373=CYLINDRICAL_SURFACE('',#86099,11.8397710119877);
#2374=CYLINDRICAL_SURFACE('',#86100,11.8397710119877);
#2375=CYLINDRICAL_SURFACE('',#86101,11.8397710119877);
#2376=CYLINDRICAL_SURFACE('',#86102,11.8397710119877);
#2377=CYLINDRICAL_SURFACE('',#86108,4.75);
#2378=CYLINDRICAL_SURFACE('',#86111,11.8397710119877);
#2379=CYLINDRICAL_SURFACE('',#86112,11.8397710119949);
#2380=CYLINDRICAL_SURFACE('',#86114,10.3625);
#2381=CYLINDRICAL_SURFACE('',#86115,9.08769033371916);
#2382=CYLINDRICAL_SURFACE('',#86117,9.0900675260086);
#2383=CYLINDRICAL_SURFACE('',#86118,9.09006752601109);
#2384=CYLINDRICAL_SURFACE('',#86129,13.);
#2385=CYLINDRICAL_SURFACE('',#86130,10.5);
#2386=CYLINDRICAL_SURFACE('',#86140,7.75);
#2387=CYLINDRICAL_SURFACE('',#86145,10.25);
#2388=CYLINDRICAL_SURFACE('',#86150,10.3625);
#2699=ELLIPSE('',#86109,4.91756185694817,4.75000000000039);
#2700=ELLIPSE('',#86110,4.91756185694847,4.75000000000065);
#9707=LINE('',#212793,#16774);
#9708=LINE('',#212860,#16775);
#9709=LINE('',#212912,#16776);
#9710=LINE('',#212962,#16777);
#9711=LINE('',#213102,#16778);
#9712=LINE('',#213238,#16779);
#9713=LINE('',#213381,#16780);
#9714=LINE('',#213518,#16781);
#9715=LINE('',#213654,#16782);
#9716=LINE('',#213790,#16783);
#9717=LINE('',#213917,#16784);
#9718=LINE('',#213931,#16785);
#9719=LINE('',#214065,#16786);
#9720=LINE('',#214206,#16787);
#9721=LINE('',#214371,#16788);
#9722=LINE('',#214529,#16789);
#9723=LINE('',#214696,#16790);
#9724=LINE('',#214861,#16791);
#9725=LINE('',#215024,#16792);
#9726=LINE('',#215033,#16793);
#9727=LINE('',#215042,#16794);
#9728=LINE('',#215120,#16795);
#9729=LINE('',#215236,#16796);
#9730=LINE('',#215256,#16797);
#9731=LINE('',#215342,#16798);
#9732=LINE('',#215414,#16799);
#9733=LINE('',#215564,#16800);
#9734=LINE('',#215710,#16801);
#9735=LINE('',#215726,#16802);
#9736=LINE('',#215804,#16803);
#9737=LINE('',#215878,#16804);
#9738=LINE('',#216014,#16805);
#9739=LINE('',#216152,#16806);
#9740=LINE('',#216169,#16807);
#9741=LINE('',#216322,#16808);
#9742=LINE('',#216480,#16809);
#9743=LINE('',#216638,#16810);
#9744=LINE('',#216670,#16811);
#9745=LINE('',#216774,#16812);
#9746=LINE('',#216856,#16813);
#9747=LINE('',#217016,#16814);
#9748=LINE('',#217176,#16815);
#9749=LINE('',#217308,#16816);
#9750=LINE('',#217410,#16817);
#9751=LINE('',#217428,#16818);
#9752=LINE('',#217843,#16819);
#9753=LINE('',#218127,#16820);
#9754=LINE('',#218166,#16821);
#9755=LINE('',#218784,#16822);
#9756=LINE('',#219053,#16823);
#9757=LINE('',#219145,#16824);
#9758=LINE('',#219220,#16825);
#9759=LINE('',#220124,#16826);
#9760=LINE('',#220620,#16827);
#9761=LINE('',#220889,#16828);
#9762=LINE('',#221310,#16829);
#9763=LINE('',#221467,#16830);
#9764=LINE('',#221472,#16831);
#9765=LINE('',#221481,#16832);
#9766=LINE('',#221485,#16833);
#9767=LINE('',#221618,#16834);
#16774=VECTOR('',#106328,10.25);
#16775=VECTOR('',#106329,10.25);
#16776=VECTOR('',#106334,1000.);
#16777=VECTOR('',#106337,10.25);
#16778=VECTOR('',#106340,10.25);
#16779=VECTOR('',#106343,10.25);
#16780=VECTOR('',#106346,10.25);
#16781=VECTOR('',#106349,10.25);
#16782=VECTOR('',#106352,10.25);
#16783=VECTOR('',#106355,10.25);
#16784=VECTOR('',#106358,13.);
#16785=VECTOR('',#106363,13.);
#16786=VECTOR('',#106368,13.);
#16787=VECTOR('',#106371,13.);
#16788=VECTOR('',#106374,13.);
#16789=VECTOR('',#106377,13.);
#16790=VECTOR('',#106380,13.);
#16791=VECTOR('',#106383,13.);
#16792=VECTOR('',#106390,13.);
#16793=VECTOR('',#106391,1000.);
#16794=VECTOR('',#106392,13.);
#16795=VECTOR('',#106395,12.87032685775);
#16796=VECTOR('',#106400,9.09006752601109);
#16797=VECTOR('',#106401,10.);
#16798=VECTOR('',#106404,9.09006752601109);
#16799=VECTOR('',#106407,9.09006752601109);
#16800=VECTOR('',#106410,9.09006752601109);
#16801=VECTOR('',#106413,9.0900675260086);
#16802=VECTOR('',#106414,10.);
#16803=VECTOR('',#106417,9.0900675260086);
#16804=VECTOR('',#106420,9.0900675260086);
#16805=VECTOR('',#106423,9.0900675260086);
#16806=VECTOR('',#106426,9.08769033371916);
#16807=VECTOR('',#106431,11.8397710119949);
#16808=VECTOR('',#106436,11.8397710119949);
#16809=VECTOR('',#106439,11.8397710119949);
#16810=VECTOR('',#106442,11.8397710119877);
#16811=VECTOR('',#106443,10.);
#16812=VECTOR('',#106446,11.8397710119877);
#16813=VECTOR('',#106449,11.8397710119877);
#16814=VECTOR('',#106452,11.8397710119877);
#16815=VECTOR('',#106455,9.75000242976401);
#16816=VECTOR('',#106468,4.75);
#16817=VECTOR('',#106479,1000.);
#16818=VECTOR('',#106480,1000.);
#16819=VECTOR('',#106489,1000.);
#16820=VECTOR('',#106490,10.);
#16821=VECTOR('',#106491,10.);
#16822=VECTOR('',#106494,10.);
#16823=VECTOR('',#106495,10.);
#16824=VECTOR('',#106498,1000.);
#16825=VECTOR('',#106513,1000.);
#16826=VECTOR('',#106514,10.);
#16827=VECTOR('',#106517,10.);
#16828=VECTOR('',#106518,10.);
#16829=VECTOR('',#106521,10.);
#16830=VECTOR('',#106526,10.5);
#16831=VECTOR('',#106533,10.75000319972);
#16832=VECTOR('',#106546,7.75);
#16833=VECTOR('',#106551,7.999997663262);
#16834=VECTOR('',#106566,1000.);
#19865=PLANE('',#86119);
#19866=PLANE('',#86120);
#19867=PLANE('',#86128);
#19868=PLANE('',#86136);
#19869=PLANE('',#86137);
#19870=PLANE('',#86138);
#19871=PLANE('',#86144);
#19872=PLANE('',#86149);
#23808=FACE_OUTER_BOUND('',#29303,.T.);
#23809=FACE_OUTER_BOUND('',#29304,.T.);
#23810=FACE_OUTER_BOUND('',#29305,.T.);
#23811=FACE_OUTER_BOUND('',#29306,.T.);
#23812=FACE_OUTER_BOUND('',#29307,.T.);
#23813=FACE_OUTER_BOUND('',#29308,.T.);
#23814=FACE_OUTER_BOUND('',#29309,.T.);
#23815=FACE_OUTER_BOUND('',#29310,.T.);
#23816=FACE_OUTER_BOUND('',#29311,.T.);
#23817=FACE_OUTER_BOUND('',#29312,.T.);
#23818=FACE_OUTER_BOUND('',#29313,.T.);
#23819=FACE_OUTER_BOUND('',#29314,.T.);
#23820=FACE_OUTER_BOUND('',#29315,.T.);
#23821=FACE_OUTER_BOUND('',#29316,.T.);
#23822=FACE_OUTER_BOUND('',#29317,.T.);
#23823=FACE_OUTER_BOUND('',#29318,.T.);
#23824=FACE_OUTER_BOUND('',#29319,.T.);
#23825=FACE_OUTER_BOUND('',#29320,.T.);
#23826=FACE_OUTER_BOUND('',#29321,.T.);
#23827=FACE_OUTER_BOUND('',#29322,.T.);
#23828=FACE_OUTER_BOUND('',#29323,.T.);
#23829=FACE_OUTER_BOUND('',#29324,.T.);
#23830=FACE_OUTER_BOUND('',#29325,.T.);
#23831=FACE_OUTER_BOUND('',#29326,.T.);
#23832=FACE_OUTER_BOUND('',#29327,.T.);
#23833=FACE_OUTER_BOUND('',#29328,.T.);
#23834=FACE_OUTER_BOUND('',#29329,.T.);
#23835=FACE_OUTER_BOUND('',#29330,.T.);
#23836=FACE_OUTER_BOUND('',#29331,.T.);
#23837=FACE_OUTER_BOUND('',#29332,.T.);
#23838=FACE_OUTER_BOUND('',#29333,.T.);
#23839=FACE_OUTER_BOUND('',#29334,.T.);
#23840=FACE_OUTER_BOUND('',#29335,.T.);
#23841=FACE_OUTER_BOUND('',#29336,.T.);
#23842=FACE_OUTER_BOUND('',#29337,.T.);
#23843=FACE_OUTER_BOUND('',#29338,.T.);
#23844=FACE_OUTER_BOUND('',#29339,.T.);
#23845=FACE_OUTER_BOUND('',#29340,.T.);
#23846=FACE_OUTER_BOUND('',#29341,.T.);
#23847=FACE_OUTER_BOUND('',#29342,.T.);
#23848=FACE_OUTER_BOUND('',#29343,.T.);
#23849=FACE_OUTER_BOUND('',#29344,.T.);
#23850=FACE_OUTER_BOUND('',#29345,.T.);
#23851=FACE_OUTER_BOUND('',#29346,.T.);
#23852=FACE_OUTER_BOUND('',#29347,.T.);
#23853=FACE_OUTER_BOUND('',#29348,.T.);
#23854=FACE_OUTER_BOUND('',#29349,.T.);
#23855=FACE_OUTER_BOUND('',#29350,.T.);
#23856=FACE_OUTER_BOUND('',#29351,.T.);
#23857=FACE_OUTER_BOUND('',#29352,.T.);
#23858=FACE_OUTER_BOUND('',#29353,.T.);
#23859=FACE_OUTER_BOUND('',#29354,.T.);
#23860=FACE_OUTER_BOUND('',#29355,.T.);
#23861=FACE_OUTER_BOUND('',#29356,.T.);
#23862=FACE_OUTER_BOUND('',#29357,.T.);
#23863=FACE_OUTER_BOUND('',#29358,.T.);
#23864=FACE_OUTER_BOUND('',#29359,.T.);
#23865=FACE_OUTER_BOUND('',#29360,.T.);
#23866=FACE_OUTER_BOUND('',#29361,.T.);
#23867=FACE_OUTER_BOUND('',#29362,.T.);
#23868=FACE_OUTER_BOUND('',#29363,.T.);
#23869=FACE_OUTER_BOUND('',#29364,.T.);
#23870=FACE_OUTER_BOUND('',#29365,.T.);
#23871=FACE_OUTER_BOUND('',#29366,.T.);
#23872=FACE_OUTER_BOUND('',#29367,.T.);
#23873=FACE_OUTER_BOUND('',#29368,.T.);
#23874=FACE_OUTER_BOUND('',#29369,.T.);
#23875=FACE_OUTER_BOUND('',#29370,.T.);
#23876=FACE_OUTER_BOUND('',#29371,.T.);
#23877=FACE_OUTER_BOUND('',#29372,.T.);
#23878=FACE_OUTER_BOUND('',#29374,.T.);
#23879=FACE_OUTER_BOUND('',#29376,.T.);
#23880=FACE_OUTER_BOUND('',#29378,.T.);
#23881=FACE_OUTER_BOUND('',#29379,.T.);
#23882=FACE_OUTER_BOUND('',#29380,.T.);
#23883=FACE_OUTER_BOUND('',#29382,.T.);
#23884=FACE_OUTER_BOUND('',#29383,.T.);
#23885=FACE_OUTER_BOUND('',#29384,.T.);
#23886=FACE_OUTER_BOUND('',#29385,.T.);
#23887=FACE_OUTER_BOUND('',#29386,.T.);
#29303=EDGE_LOOP('',(#74809,#74810,#74811,#74812,#74813,#74814,#74815,#74816,
#74817,#74818,#74819,#74820,#74821));
#29304=EDGE_LOOP('',(#74822,#74823,#74824,#74825));
#29305=EDGE_LOOP('',(#74826,#74827,#74828,#74829));
#29306=EDGE_LOOP('',(#74830,#74831,#74832,#74833,#74834));
#29307=EDGE_LOOP('',(#74835,#74836,#74837,#74838,#74839));
#29308=EDGE_LOOP('',(#74840,#74841,#74842,#74843));
#29309=EDGE_LOOP('',(#74844,#74845,#74846,#74847));
#29310=EDGE_LOOP('',(#74848,#74849,#74850,#74851,#74852));
#29311=EDGE_LOOP('',(#74853,#74854,#74855));
#29312=EDGE_LOOP('',(#74856,#74857,#74858,#74859,#74860,#74861,#74862));
#29313=EDGE_LOOP('',(#74863,#74864,#74865,#74866,#74867));
#29314=EDGE_LOOP('',(#74868,#74869,#74870,#74871,#74872));
#29315=EDGE_LOOP('',(#74873,#74874,#74875,#74876));
#29316=EDGE_LOOP('',(#74877,#74878,#74879,#74880,#74881));
#29317=EDGE_LOOP('',(#74882,#74883,#74884,#74885,#74886));
#29318=EDGE_LOOP('',(#74887,#74888,#74889,#74890));
#29319=EDGE_LOOP('',(#74891,#74892,#74893,#74894,#74895,#74896,#74897,#74898,
#74899,#74900));
#29320=EDGE_LOOP('',(#74901,#74902,#74903,#74904,#74905,#74906));
#29321=EDGE_LOOP('',(#74907,#74908,#74909,#74910,#74911));
#29322=EDGE_LOOP('',(#74912,#74913,#74914,#74915));
#29323=EDGE_LOOP('',(#74916,#74917,#74918,#74919));
#29324=EDGE_LOOP('',(#74920,#74921,#74922,#74923));
#29325=EDGE_LOOP('',(#74924,#74925,#74926,#74927,#74928));
#29326=EDGE_LOOP('',(#74929,#74930,#74931,#74932));
#29327=EDGE_LOOP('',(#74933,#74934,#74935,#74936));
#29328=EDGE_LOOP('',(#74937,#74938,#74939,#74940));
#29329=EDGE_LOOP('',(#74941,#74942,#74943,#74944));
#29330=EDGE_LOOP('',(#74945,#74946,#74947,#74948));
#29331=EDGE_LOOP('',(#74949,#74950,#74951,#74952));
#29332=EDGE_LOOP('',(#74953,#74954,#74955,#74956));
#29333=EDGE_LOOP('',(#74957,#74958,#74959,#74960,#74961));
#29334=EDGE_LOOP('',(#74962,#74963,#74964,#74965));
#29335=EDGE_LOOP('',(#74966,#74967,#74968,#74969));
#29336=EDGE_LOOP('',(#74970,#74971,#74972,#74973));
#29337=EDGE_LOOP('',(#74974,#74975,#74976,#74977,#74978,#74979,#74980));
#29338=EDGE_LOOP('',(#74981,#74982,#74983));
#29339=EDGE_LOOP('',(#74984,#74985,#74986,#74987));
#29340=EDGE_LOOP('',(#74988,#74989,#74990,#74991));
#29341=EDGE_LOOP('',(#74992,#74993,#74994,#74995));
#29342=EDGE_LOOP('',(#74996,#74997,#74998,#74999,#75000));
#29343=EDGE_LOOP('',(#75001,#75002,#75003,#75004,#75005,#75006,#75007));
#29344=EDGE_LOOP('',(#75008,#75009,#75010,#75011,#75012,#75013));
#29345=EDGE_LOOP('',(#75014,#75015,#75016,#75017,#75018,#75019));
#29346=EDGE_LOOP('',(#75020,#75021,#75022,#75023));
#29347=EDGE_LOOP('',(#75024,#75025,#75026,#75027,#75028,#75029,#75030,#75031,
#75032,#75033,#75034,#75035,#75036));
#29348=EDGE_LOOP('',(#75037,#75038,#75039,#75040,#75041,#75042,#75043,#75044,
#75045,#75046,#75047,#75048,#75049));
#29349=EDGE_LOOP('',(#75050,#75051,#75052,#75053,#75054));
#29350=EDGE_LOOP('',(#75055,#75056,#75057,#75058));
#29351=EDGE_LOOP('',(#75059,#75060,#75061,#75062,#75063));
#29352=EDGE_LOOP('',(#75064,#75065,#75066,#75067,#75068,#75069,#75070,#75071,
#75072,#75073,#75074,#75075,#75076,#75077));
#29353=EDGE_LOOP('',(#75078,#75079,#75080,#75081,#75082,#75083,#75084,#75085,
#75086,#75087,#75088,#75089,#75090,#75091));
#29354=EDGE_LOOP('',(#75092,#75093,#75094,#75095,#75096,#75097,#75098,#75099));
#29355=EDGE_LOOP('',(#75100,#75101,#75102,#75103,#75104));
#29356=EDGE_LOOP('',(#75105,#75106,#75107,#75108,#75109,#75110,#75111,#75112,
#75113));
#29357=EDGE_LOOP('',(#75114,#75115,#75116));
#29358=EDGE_LOOP('',(#75117,#75118,#75119,#75120));
#29359=EDGE_LOOP('',(#75121,#75122,#75123,#75124,#75125));
#29360=EDGE_LOOP('',(#75126,#75127,#75128,#75129,#75130,#75131,#75132,#75133,
#75134,#75135,#75136,#75137));
#29361=EDGE_LOOP('',(#75138,#75139,#75140,#75141,#75142));
#29362=EDGE_LOOP('',(#75143,#75144,#75145,#75146));
#29363=EDGE_LOOP('',(#75147,#75148,#75149,#75150,#75151));
#29364=EDGE_LOOP('',(#75152,#75153,#75154,#75155,#75156,#75157,#75158,#75159,
#75160,#75161,#75162));
#29365=EDGE_LOOP('',(#75163,#75164,#75165,#75166,#75167,#75168,#75169,#75170,
#75171,#75172));
#29366=EDGE_LOOP('',(#75173,#75174,#75175,#75176,#75177,#75178,#75179,#75180,
#75181,#75182,#75183));
#29367=EDGE_LOOP('',(#75184,#75185,#75186,#75187,#75188));
#29368=EDGE_LOOP('',(#75189,#75190,#75191,#75192,#75193,#75194,#75195,#75196,
#75197,#75198));
#29369=EDGE_LOOP('',(#75199,#75200,#75201,#75202,#75203,#75204,#75205,#75206,
#75207));
#29370=EDGE_LOOP('',(#75208,#75209,#75210,#75211,#75212));
#29371=EDGE_LOOP('',(#75213,#75214,#75215,#75216,#75217));
#29372=EDGE_LOOP('',(#75218,#75219,#75220,#75221,#75222,#75223,#75224));
#29373=EDGE_LOOP('',(#75225));
#29374=EDGE_LOOP('',(#75226));
#29375=EDGE_LOOP('',(#75227));
#29376=EDGE_LOOP('',(#75228));
#29377=EDGE_LOOP('',(#75229));
#29378=EDGE_LOOP('',(#75230,#75231,#75232,#75233));
#29379=EDGE_LOOP('',(#75234,#75235,#75236,#75237));
#29380=EDGE_LOOP('',(#75238,#75239,#75240,#75241,#75242));
#29381=EDGE_LOOP('',(#75243));
#29382=EDGE_LOOP('',(#75244,#75245,#75246,#75247,#75248,#75249,#75250,#75251));
#29383=EDGE_LOOP('',(#75252,#75253,#75254,#75255,#75256,#75257,#75258,#75259,
#75260,#75261,#75262,#75263));
#29384=EDGE_LOOP('',(#75264,#75265,#75266,#75267,#75268,#75269,#75270,#75271,
#75272));
#29385=EDGE_LOOP('',(#75273,#75274,#75275,#75276));
#29386=EDGE_LOOP('',(#75277,#75278,#75279,#75280));
#30485=B_SPLINE_CURVE_WITH_KNOTS('',3,(#212795,#212796,#212797,#212798,
#212799,#212800,#212801,#212802,#212803,#212804,#212805,#212806,#212807,
#212808,#212809,#212810,#212811,#212812,#212813,#212814,#212815,#212816,
#212817,#212818,#212819,#212820,#212821,#212822,#212823,#212824,#212825,
#212826,#212827,#212828,#212829,#212830,#212831,#212832,#212833,#212834,
#212835,#212836,#212837,#212838,#212839,#212840,#212841,#212842,#212843,
#212844,#212845,#212846,#212847,#212848,#212849,#212850,#212851,#212852,
#212853,#212854,#212855,#212856,#212857,#212858),.UNSPECIFIED.,.F.,.F.,
(4,2,2,2,2,2,2,2,2,2,2,2,2,2,2,2,2,2,2,2,2,2,2,2,2,2,2,2,2,2,2,4),(-23.4655815117522,
-23.3821633536412,-23.2277363527294,-23.0362474977428,-22.8467003384102,
-22.649719777506,-22.3128056337548,-22.1099831860358,-21.9074402590789,
-21.8087745346896,-21.4994489052755,-21.4005123478419,-21.0840256137525,
-20.9058937064287,-20.7532789815947,-20.562208019526,-20.3727918208678,
-20.1760490515299,-19.7704517016932,-19.3649166721905,-19.0881265530438,
-18.8239123291825,-18.6794135983185,-18.4723542547888,-18.37203416693,-18.1810349703384,
-18.0313863852817,-17.8735599285529,-17.6813646175406,-17.4915681537435,
-17.2941928509983,-17.0142195375219),.UNSPECIFIED.);
#30486=B_SPLINE_CURVE_WITH_KNOTS('',3,(#212865,#212866,#212867,#212868,
#212869,#212870,#212871,#212872,#212873,#212874,#212875,#212876,#212877,
#212878,#212879,#212880,#212881,#212882,#212883,#212884,#212885,#212886),
 .UNSPECIFIED.,.F.,.F.,(4,2,2,2,2,2,2,2,2,2,4),(-25.3579380604563,-25.2126790926101,
-25.0707763793626,-24.7883580752298,-24.6165805135713,-24.4630647928614,
-24.2717305560932,-24.0822302806376,-23.8853298566005,-23.5490789423312,
-23.4655815117522),.UNSPECIFIED.);
#30487=B_SPLINE_CURVE_WITH_KNOTS('',3,(#212888,#212889,#212890,#212891,
#212892,#212893,#212894,#212895,#212896,#212897,#212898,#212899),
 .UNSPECIFIED.,.F.,.F.,(4,2,2,2,2,4),(0.,0.250779295927683,0.498420132327997,
0.665822634254242,0.997622742450503,1.3324035533165),.UNSPECIFIED.);
#30488=B_SPLINE_CURVE_WITH_KNOTS('',3,(#212901,#212902,#212903,#212904,
#212905,#212906,#212907,#212908,#212909,#212910),.UNSPECIFIED.,.F.,.F.,
(4,2,2,2,4),(1.00000001185067E-6,0.17890870313989,0.360010001015589,0.541048047586756,
0.720025159562407),.UNSPECIFIED.);
#30489=B_SPLINE_CURVE_WITH_KNOTS('',3,(#212914,#212915,#212916,#212917,
#212918,#212919,#212920,#212921,#212922,#212923),.UNSPECIFIED.,.F.,.F.,
(4,2,2,2,4),(9.72076722368276E-6,0.179235827648045,0.360521578492218,0.541895207425194,
0.721026938706915),.UNSPECIFIED.);
#30490=B_SPLINE_CURVE_WITH_KNOTS('',3,(#212925,#212926,#212927,#212928,
#212929,#212930,#212931,#212932,#212933,#212934,#212935,#212936),
 .UNSPECIFIED.,.F.,.F.,(4,2,2,2,2,4),(4.89083575544467E-5,0.335287965816992,
0.667578151924596,0.835217190795273,1.08321230565055,1.334348166746),
 .UNSPECIFIED.);
#30491=B_SPLINE_CURVE_WITH_KNOTS('',3,(#212937,#212938,#212939,#212940,
#212941,#212942,#212943,#212944,#212945,#212946,#212947,#212948,#212949,
#212950,#212951,#212952,#212953,#212954,#212955,#212956,#212957,#212958),
 .UNSPECIFIED.,.F.,.F.,(4,2,2,2,2,2,2,2,2,2,4),(-1.89255759737355,-1.80353521663288,
-1.60097725222907,-1.3981474008695,-1.05868693104851,-0.86140418669837,
-0.671667910335707,-0.508679971146122,-0.262571560520725,-0.132568711431051,
-0.000222633785011576),.UNSPECIFIED.);
#30492=B_SPLINE_CURVE_WITH_KNOTS('',3,(#212963,#212964,#212965,#212966,
#212967,#212968,#212969,#212970,#212971,#212972,#212973,#212974,#212975,
#212976,#212977,#212978,#212979,#212980,#212981,#212982,#212983,#212984,
#212985,#212986,#212987,#212988,#212989,#212990,#212991,#212992,#212993,
#212994,#212995,#212996,#212997,#212998,#212999,#213000,#213001,#213002,
#213003,#213004,#213005,#213006,#213007,#213008,#213009,#213010,#213011,
#213012,#213013,#213014,#213015,#213016,#213017,#213018,#213019,#213020,
#213021,#213022,#213023,#213024,#213025,#213026,#213027,#213028,#213029,
#213030,#213031,#213032),.UNSPECIFIED.,.F.,.F.,(4,2,2,2,2,2,2,2,2,2,2,2,
2,2,2,2,2,2,2,2,2,2,2,2,2,2,2,2,2,2,2,2,2,2,4),(-17.0142195375219,-16.9539796203354,
-16.7890489696158,-16.6342677925073,-16.4426964451876,-16.2531188482399,
-16.0560894062044,-15.7188030761123,-15.5159750456067,-15.3134253016677,
-15.1583517074344,-15.0588606872297,-14.6532131620584,-14.2480183614723,
-14.0613034149302,-13.9082183743288,-13.7051158366063,-13.5460702373005,
-13.263110126487,-13.0703537647283,-12.9197353366452,-12.820016273049,-12.6770837035873,
-12.5342903108104,-12.3394687327371,-12.2390554377965,-12.0233345598109,
-11.8716865495169,-11.6868040567647,-11.4843070065672,-11.1768445161315,
-10.9977790660545,-10.7593578972188,-10.5702642746217,-10.5638492065124),
 .UNSPECIFIED.);
#30493=B_SPLINE_CURVE_WITH_KNOTS('',3,(#213033,#213034,#213035,#213036,
#213037,#213038,#213039,#213040,#213041,#213042,#213043,#213044,#213045,
#213046,#213047,#213048,#213049,#213050,#213051,#213052,#213053,#213054,
#213055,#213056,#213057,#213058,#213059,#213060,#213061,#213062,#213063,
#213064,#213065,#213066,#213067,#213068,#213069,#213070,#213071,#213072,
#213073,#213074,#213075,#213076,#213077,#213078,#213079,#213080,#213081,
#213082,#213083,#213084,#213085,#213086,#213087,#213088,#213089,#213090,
#213091,#213092,#213093,#213094,#213095,#213096,#213097,#213098),
 .UNSPECIFIED.,.F.,.F.,(4,2,2,2,2,2,2,2,2,2,2,2,2,2,2,2,2,2,2,2,2,2,2,2,
2,2,2,2,2,2,2,2,4),(-8.34439189346545,-8.24590534832181,-8.14668971659077,
-8.0049280196085,-7.90578734244284,-7.75527402355542,-7.56164635479124,
-7.28035238806601,-7.12534157358082,-6.92238574982098,-6.75614142420925,
-6.4185497256095,-6.22148570635503,-6.03188435919294,-5.84024949079621,
-5.68516707862395,-5.52189531741973,-5.17828352388869,-4.77275280538589,
-4.57628006212064,-4.38699097039336,-4.19638854892432,-4.0456449408773,
-3.85387561061917,-3.56891093370617,-3.36522566092619,-3.20822221584918,
-3.05476221089561,-2.86850590511233,-2.4632747529187,-2.05761577697304,
-1.95813288497916,-1.89255759737355),.UNSPECIFIED.);
#30494=B_SPLINE_CURVE_WITH_KNOTS('',3,(#213103,#213104,#213105,#213106,
#213107,#213108,#213109,#213110,#213111,#213112,#213113,#213114,#213115,
#213116,#213117,#213118,#213119,#213120,#213121,#213122,#213123,#213124,
#213125,#213126,#213127,#213128,#213129,#213130,#213131,#213132,#213133,
#213134,#213135,#213136,#213137,#213138,#213139,#213140,#213141,#213142,
#213143,#213144,#213145,#213146,#213147,#213148,#213149,#213150,#213151,
#213152,#213153,#213154,#213155,#213156,#213157,#213158,#213159,#213160,
#213161,#213162,#213163,#213164,#213165,#213166,#213167,#213168),
 .UNSPECIFIED.,.F.,.F.,(4,2,2,2,2,2,2,2,2,2,2,2,2,2,2,2,2,2,2,2,2,2,2,2,
2,2,2,2,2,2,2,2,4),(-10.5638492065124,-10.3665281400106,-10.2065643589849,
-10.0657701952293,-9.96554246102645,-9.81531484461045,-9.61940377013227,
-9.41681481261266,-9.16094167265437,-8.88884314638493,-8.69155264734285,
-8.50181173061584,-8.30976242994707,-8.15264143083408,-7.99976837552985,
-7.81280965557528,-7.40763311197167,-7.00199007004737,-6.90249478182624,
-6.7471184359148,-6.42909757011231,-6.33010686318968,-6.12761283321231,
-5.81684026459228,-5.63219570194093,-5.48423490732585,-5.28150664967726,
-5.08689708330431,-4.80741352692034,-4.6564265426323,-4.45361226970384,
-4.27215445416353,-4.11333321794941),.UNSPECIFIED.);
#30495=B_SPLINE_CURVE_WITH_KNOTS('',3,(#213169,#213170,#213171,#213172,
#213173,#213174,#213175,#213176,#213177,#213178,#213179,#213180,#213181,
#213182,#213183,#213184,#213185,#213186,#213187,#213188,#213189,#213190,
#213191,#213192,#213193,#213194,#213195,#213196,#213197,#213198,#213199,
#213200,#213201,#213202,#213203,#213204,#213205,#213206,#213207,#213208,
#213209,#213210,#213211,#213212,#213213,#213214,#213215,#213216,#213217,
#213218,#213219,#213220,#213221,#213222,#213223,#213224,#213225,#213226,
#213227,#213228,#213229,#213230,#213231,#213232,#213233,#213234),
 .UNSPECIFIED.,.F.,.F.,(4,2,2,2,2,2,2,2,2,2,2,2,2,2,2,2,2,2,2,2,2,2,2,2,
2,2,2,2,2,2,2,2,4),(-14.7964729471967,-14.7930121131524,-14.6037362465881,
-14.4072806385629,-14.0017540267854,-13.6582611829268,-13.4949397283514,
-13.3398727218517,-13.1209657585198,-13.0205232688638,-12.8243944231431,
-12.6819509109363,-12.5393934714743,-12.4394141585229,-12.2887441952975,
-12.0963925010855,-11.8126276373192,-11.6515132105288,-11.448327176925,
-11.3012939126661,-11.1069033964773,-11.0064990991705,-10.7918073490527,
-10.6411697653991,-10.4485619690297,-10.1653115199523,-10.005523195632,
-9.80239002765117,-9.65153351059004,-9.46206185717822,-9.05703579811716,
-8.65139829862876,-8.34439189346545),.UNSPECIFIED.);
#30496=B_SPLINE_CURVE_WITH_KNOTS('',3,(#213240,#213241,#213242,#213243,
#213244,#213245,#213246,#213247,#213248,#213249,#213250,#213251,#213252,
#213253,#213254,#213255,#213256,#213257,#213258,#213259,#213260,#213261,
#213262,#213263,#213264,#213265,#213266,#213267),.UNSPECIFIED.,.F.,.F.,
(4,2,2,2,2,2,2,2,2,2,2,2,2,4),(-25.3599939626477,-25.2110052268727,-25.0658395881092,
-24.7731830676316,-24.6302233121548,-24.4709374768147,-24.2672182293805,
-24.0781558955,-23.8400128244761,-23.6610071037644,-23.353579459936,-23.1510946673596,
-23.0520783263848,-23.0237218553495),.UNSPECIFIED.);
#30497=B_SPLINE_CURVE_WITH_KNOTS('',3,(#213268,#213269,#213270,#213271,
#213272,#213273,#213274,#213275,#213276,#213277,#213278,#213279,#213280,
#213281,#213282,#213283,#213284,#213285,#213286,#213287,#213288,#213289,
#213290,#213291,#213292,#213293,#213294,#213295,#213296,#213297,#213298,
#213299,#213300,#213301,#213302,#213303,#213304,#213305,#213306,#213307,
#213308,#213309,#213310,#213311),.UNSPECIFIED.,.F.,.F.,(4,2,2,2,2,2,2,2,
2,2,2,2,2,2,2,2,2,2,2,2,2,4),(-4.11333321794941,-3.96076191479785,-3.86202062745145,
-3.54599574300317,-3.44707915710504,-3.13716544626074,-3.03848011624721,
-2.72045780085061,-2.62146595892779,-2.41896937024694,-2.10817748977627,
-1.92349758118348,-1.77537722483771,-1.5726426679254,-1.37872992888174,
-1.09796693044656,-0.944179154417269,-0.741277533053446,-0.570394112429525,
-0.287612371759698,-0.145595795194013,-5.55694362388068E-6),
 .UNSPECIFIED.);
#30498=B_SPLINE_CURVE_WITH_KNOTS('',3,(#213312,#213313,#213314,#213315,
#213316,#213317,#213318,#213319,#213320,#213321,#213322,#213323,#213324,
#213325,#213326,#213327,#213328,#213329,#213330,#213331,#213332,#213333,
#213334,#213335,#213336,#213337,#213338,#213339,#213340,#213341,#213342,
#213343,#213344,#213345,#213346,#213347,#213348,#213349,#213350,#213351,
#213352,#213353,#213354,#213355,#213356,#213357,#213358,#213359,#213360,
#213361,#213362,#213363,#213364,#213365,#213366,#213367,#213368,#213369,
#213370,#213371,#213372,#213373,#213374,#213375,#213376,#213377),
 .UNSPECIFIED.,.F.,.F.,(4,2,2,2,2,2,2,2,2,2,2,2,2,2,2,2,2,2,2,2,2,2,2,2,
2,2,2,2,2,2,2,2,4),(-21.2462595254853,-21.0130526317412,-20.6600149992664,
-20.5011090444902,-20.2980763381775,-20.0685171116799,-19.8659046223187,
-19.6629317394128,-19.4602424779167,-19.2488692412891,-19.1003391764158,
-18.9119956891045,-18.7227658705206,-18.5264138806326,-18.1946275381072,
-18.0253752742207,-17.8713489015093,-17.586778234647,-17.384325934204,-17.2851176679844,
-17.0156489622446,-16.7691855010582,-16.6235747431412,-16.414894933244,
-16.3145588184473,-16.1228121116564,-15.9737542503545,-15.7706040124235,
-15.610203095414,-15.3267169747295,-15.1342348821604,-14.9835871024164,
-14.7964729471967),.UNSPECIFIED.);
#30499=B_SPLINE_CURVE_WITH_KNOTS('',3,(#213382,#213383,#213384,#213385,
#213386,#213387,#213388,#213389,#213390,#213391,#213392,#213393,#213394,
#213395,#213396,#213397,#213398,#213399,#213400,#213401,#213402,#213403,
#213404,#213405,#213406,#213407,#213408,#213409,#213410,#213411,#213412,
#213413,#213414,#213415,#213416,#213417,#213418,#213419,#213420,#213421,
#213422,#213423,#213424,#213425,#213426,#213427,#213428,#213429,#213430,
#213431,#213432,#213433,#213434,#213435,#213436,#213437,#213438,#213439,
#213440,#213441,#213442,#213443),.UNSPECIFIED.,.F.,.F.,(4,2,2,2,2,2,2,2,
2,2,2,2,2,2,2,2,2,2,2,2,2,2,2,2,2,2,2,2,2,2,4),(-23.0237218553495,-22.7829578146256,
-22.53985611019,-22.3372736023383,-22.1979623272724,-22.0150657011536,-21.7052985547119,
-21.5028125493589,-21.4038147651851,-21.085595223343,-20.9085658857745,
-20.7057289281245,-20.5536435482767,-20.3682264157039,-20.1726079358586,
-19.8466166265223,-19.6741889045732,-19.5206951783369,-19.3294245802063,
-19.1399535116033,-18.9431008723126,-18.5375013263223,-18.2636250828212,
-18.004062687006,-17.801480911653,-17.6064861128457,-17.4561549159828,-17.2417879958575,
-17.0663359785854,-16.7612726574011,-16.5735077595754),.UNSPECIFIED.);
#30500=B_SPLINE_CURVE_WITH_KNOTS('',3,(#213445,#213446,#213447,#213448,
#213449,#213450,#213451,#213452,#213453,#213454,#213455,#213456,#213457,
#213458,#213459,#213460,#213461,#213462,#213463,#213464,#213465,#213466,
#213467,#213468,#213469,#213470,#213471,#213472,#213473,#213474,#213475,
#213476,#213477,#213478,#213479,#213480,#213481,#213482,#213483,#213484,
#213485,#213486),.UNSPECIFIED.,.F.,.F.,(4,2,2,2,2,2,2,2,2,2,2,2,2,2,2,2,
2,2,2,2,4),(-25.3598482220487,-25.2134211082989,-25.0706251162533,-24.7853399490412,
-24.6208618383294,-24.4178851639507,-24.2622830408013,-23.9807185207273,
-23.7872130499894,-23.5844639595727,-23.3696718488658,-23.1670170319282,
-22.9595539400521,-22.7568765161118,-22.5470207421421,-22.3983316917044,
-22.2097930130438,-22.0205546305087,-21.8241908375456,-21.418680597865,
-21.2462595254853),.UNSPECIFIED.);
#30501=B_SPLINE_CURVE_WITH_KNOTS('',3,(#213487,#213488,#213489,#213490,
#213491,#213492,#213493,#213494,#213495,#213496,#213497,#213498,#213499,
#213500,#213501,#213502,#213503,#213504,#213505,#213506,#213507,#213508,
#213509,#213510,#213511,#213512,#213513,#213514),.UNSPECIFIED.,.F.,.F.,
(4,2,2,2,2,2,2,2,2,2,2,2,2,4),(-2.33721822141003,-2.31110570753062,-2.21223251201049,
-1.90071971511215,-1.80197161402924,-1.48609808399419,-1.38718479643066,
-1.076992667329,-0.978293896948929,-0.660945421098482,-0.499220557990324,
-0.258250015726861,-0.130322448606808,-5.55694360169744E-6),
 .UNSPECIFIED.);
#30502=B_SPLINE_CURVE_WITH_KNOTS('',3,(#213519,#213520,#213521,#213522,
#213523,#213524,#213525,#213526,#213527,#213528,#213529,#213530,#213531,
#213532,#213533,#213534,#213535,#213536,#213537,#213538,#213539,#213540,
#213541,#213542,#213543,#213544,#213545,#213546,#213547,#213548,#213549,
#213550,#213551,#213552,#213553,#213554,#213555,#213556,#213557,#213558,
#213559,#213560,#213561,#213562,#213563,#213564,#213565,#213566,#213567,
#213568,#213569,#213570,#213571,#213572,#213573,#213574,#213575,#213576,
#213577,#213578,#213579,#213580,#213581,#213582,#213583,#213584),
 .UNSPECIFIED.,.F.,.F.,(4,2,2,2,2,2,2,2,2,2,2,2,2,2,2,2,2,2,2,2,2,2,2,2,
2,2,2,2,2,2,2,2,4),(-16.5735077595754,-16.558788014462,-16.4597521147959,
-16.1906086541584,-16.0245717260025,-15.8367395841997,-15.6409285758089,
-15.313443646354,-15.1418470460958,-14.9882133987819,-14.7969063470367,
-14.6074203021057,-14.410544531441,-14.0049311364927,-13.7310093334175,
-13.4713700195003,-13.2687826464027,-13.0737994753134,-12.923462076633,
-12.8253058156821,-12.68010861894,-12.5351957885283,-12.3477195958187,-11.9425815080008,
-11.5369479410831,-11.437442651998,-11.2814916431801,-10.9654562255593,
-10.8665420645695,-10.5566653339251,-10.4579842233931,-10.1399353299562,
-10.1215558732796),.UNSPECIFIED.);
#30503=B_SPLINE_CURVE_WITH_KNOTS('',3,(#213585,#213586,#213587,#213588,
#213589,#213590,#213591,#213592,#213593,#213594,#213595,#213596,#213597,
#213598,#213599,#213600,#213601,#213602,#213603,#213604,#213605,#213606,
#213607,#213608,#213609,#213610,#213611,#213612,#213613,#213614,#213615,
#213616,#213617,#213618,#213619,#213620,#213621,#213622,#213623,#213624,
#213625,#213626,#213627,#213628,#213629,#213630,#213631,#213632,#213633,
#213634,#213635,#213636,#213637,#213638,#213639,#213640,#213641,#213642,
#213643,#213644,#213645,#213646,#213647,#213648,#213649,#213650),
 .UNSPECIFIED.,.F.,.F.,(4,2,2,2,2,2,2,2,2,2,2,2,2,2,2,2,2,2,2,2,2,2,2,2,
2,2,2,2,2,2,2,2,4),(-8.78646590511648,-8.69447764122115,-8.50512180829162,
-8.31427326472456,-8.16256695330588,-7.97809447067373,-7.77559387977924,
-7.46594770522954,-7.28328997819737,-7.14515274060527,-6.94255908319348,
-6.69117979097634,-6.42066375919234,-6.2243223411716,-6.03509287700676,
-5.84714336525967,-5.69892935521848,-5.48430236760396,-5.28156262317273,
-5.08768687858614,-4.80685766016851,-4.65291432428607,-4.44999718079432,
-4.27993773196351,-3.9496315087519,-3.75346099655457,-3.56430030673111,
-3.38227916274677,-3.23818448040399,-2.96662657818636,-2.82057795462476,
-2.58018133296781,-2.33721822141003),.UNSPECIFIED.);
#30504=B_SPLINE_CURVE_WITH_KNOTS('',3,(#213655,#213656,#213657,#213658,
#213659,#213660,#213661,#213662,#213663,#213664,#213665,#213666,#213667,
#213668,#213669,#213670,#213671,#213672,#213673,#213674,#213675,#213676,
#213677,#213678,#213679,#213680,#213681,#213682,#213683,#213684,#213685,
#213686,#213687,#213688,#213689,#213690,#213691,#213692,#213693,#213694,
#213695,#213696,#213697,#213698,#213699,#213700,#213701,#213702,#213703,
#213704,#213705,#213706,#213707,#213708,#213709,#213710,#213711,#213712,
#213713,#213714,#213715,#213716,#213717,#213718),.UNSPECIFIED.,.F.,.F.,
(4,2,2,2,2,2,2,2,2,2,2,2,2,2,2,2,2,2,2,2,2,2,2,2,2,2,2,2,2,2,2,4),(-10.1215558732796,
-10.0409453002839,-9.83845542996561,-9.52785452984907,-9.34350900069316,
-9.19707221940522,-8.99438494390757,-8.7925223606963,-8.58992278550474,
-8.35652235900569,-8.15340240102332,-8.0019933378063,-7.81322384890866,
-7.40816004464301,-7.00252650556468,-6.90298973191125,-6.74558906250778,
-6.43423701736284,-6.33549805144709,-6.01942533379578,-5.92050772757459,
-5.61066228809942,-5.51198031710246,-5.1938716118372,-5.09487729173345,
-4.89238287118889,-4.58202669110098,-4.39812304091263,-4.2539365260713,
-4.05128954032214,-3.83776873148533,-3.67017174968231),.UNSPECIFIED.);
#30505=B_SPLINE_CURVE_WITH_KNOTS('',3,(#213719,#213720,#213721,#213722,
#213723,#213724,#213725,#213726,#213727,#213728,#213729,#213730,#213731,
#213732,#213733,#213734,#213735,#213736,#213737,#213738,#213739,#213740,
#213741,#213742,#213743,#213744,#213745,#213746,#213747,#213748,#213749,
#213750,#213751,#213752,#213753,#213754,#213755,#213756,#213757,#213758,
#213759,#213760,#213761,#213762,#213763,#213764,#213765,#213766,#213767,
#213768,#213769,#213770,#213771,#213772,#213773,#213774,#213775,#213776,
#213777,#213778,#213779,#213780,#213781,#213782,#213783,#213784,#213785,
#213786),.UNSPECIFIED.,.F.,.F.,(4,2,2,2,2,2,2,2,2,2,2,2,2,2,2,2,2,2,2,2,
2,2,2,2,2,2,2,2,2,2,2,2,2,4),(-15.2367903044136,-14.8893236437563,-14.7291495722032,
-14.5261341402795,-14.3693368356338,-14.1830571286185,-13.9873569675475,
-13.6608086821188,-13.4886697502539,-13.3351159169796,-13.1175658866552,
-13.0171341357064,-12.8215524175462,-12.6789588457294,-12.536241436693,
-12.4363691812245,-12.2857172284162,-12.0931903303355,-11.8097624008203,
-11.6495335418658,-11.4463782081366,-11.2967969002635,-11.1057014414873,
-11.0053745853545,-10.7981093394651,-10.6534740075858,-10.391513092408,
-10.116228035644,-9.71058551650308,-9.51313229873795,-9.32327827108487,
-9.22500334979002,-8.89109260896205,-8.78646590511648),.UNSPECIFIED.);
#30506=B_SPLINE_CURVE_WITH_KNOTS('',3,(#213792,#213793,#213794,#213795,
#213796,#213797,#213798,#213799,#213800,#213801,#213802,#213803,#213804,
#213805,#213806,#213807,#213808,#213809,#213810,#213811,#213812,#213813,
#213814,#213815),.UNSPECIFIED.,.F.,.F.,(4,2,2,2,2,2,2,2,2,2,2,4),(5.07374035434672E-5,
0.19606314902765,0.390967942257509,0.792252129422002,1.19229882428601,1.39196195962845,
1.5908744447054,1.78833640693294,1.98791847080156,2.18776996778386,2.48510060443345,
2.78256740042348),.UNSPECIFIED.);
#30507=B_SPLINE_CURVE_WITH_KNOTS('',3,(#213816,#213817,#213818,#213819,
#213820,#213821,#213822,#213823,#213824,#213825,#213826,#213827,#213828,
#213829,#213830,#213831,#213832,#213833,#213834,#213835,#213836,#213837,
#213838,#213839,#213840,#213841,#213842,#213843,#213844,#213845,#213846,
#213847,#213848,#213849,#213850,#213851),.UNSPECIFIED.,.F.,.F.,(4,2,2,2,
2,2,2,2,2,2,2,2,2,2,2,2,2,4),(-3.67017174968231,-3.635048745841,-3.43815758420685,
-3.23556456026557,-2.98357247568108,-2.7128797384741,-2.51641098932753,
-2.32712518426374,-2.13652722295863,-1.98578976714053,-1.79398833616895,
-1.50909393296523,-1.30541347022808,-1.14838131573872,-0.99497187110547,
-0.808745254833481,-0.403515045478468,-1.91474428097279E-5),
 .UNSPECIFIED.);
#30508=B_SPLINE_CURVE_WITH_KNOTS('',3,(#213852,#213853,#213854,#213855,
#213856,#213857,#213858,#213859,#213860,#213861,#213862,#213863,#213864,
#213865,#213866,#213867,#213868,#213869,#213870,#213871,#213872,#213873,
#213874,#213875,#213876,#213877,#213878,#213879,#213880,#213881,#213882,
#213883,#213884,#213885,#213886,#213887,#213888,#213889,#213890,#213891,
#213892,#213893,#213894,#213895,#213896,#213897,#213898,#213899,#213900,
#213901,#213902,#213903,#213904,#213905,#213906,#213907,#213908,#213909,
#213910,#213911,#213912,#213913),.UNSPECIFIED.,.F.,.F.,(4,2,2,2,2,2,2,2,
2,2,2,2,2,2,2,2,2,2,2,2,2,2,2,2,2,2,2,2,2,2,4),(-21.6906362475869,-21.5013896141299,
-21.4024213539677,-21.0851404732035,-20.9864295651607,-20.6759526794773,
-20.5770475261363,-20.2614416858976,-20.1053469575417,-20.0058352989294,
-19.600192486939,-19.2232859369709,-19.020710368846,-18.8179491194557,-18.6154479835255,
-18.5164835795067,-18.1992767642662,-18.1005651025437,-17.7900401315637,
-17.6323657521275,-17.5328237855654,-17.127198587604,-16.722159016726,-16.5331182952159,
-16.3819210436559,-16.2244362917703,-16.0323087166128,-15.8425383011383,
-15.6452009065229,-15.2395449589195,-15.2367903044136),.UNSPECIFIED.);
#30509=B_SPLINE_CURVE_WITH_KNOTS('',3,(#213919,#213920,#213921,#213922,
#213923,#213924,#213925,#213926),.UNSPECIFIED.,.F.,.F.,(4,2,2,4),(9.21790452008223,
9.4318832005907,9.73296466445621,10.0352832223881),.UNSPECIFIED.);
#30510=B_SPLINE_CURVE_WITH_KNOTS('',3,(#213932,#213933,#213934,#213935,
#213936,#213937,#213938,#213939,#213940,#213941,#213942,#213943,#213944,
#213945,#213946,#213947,#213948,#213949,#213950,#213951,#213952,#213953,
#213954,#213955,#213956,#213957,#213958,#213959,#213960,#213961,#213962,
#213963,#213964,#213965,#213966,#213967,#213968,#213969,#213970,#213971,
#213972,#213973,#213974,#213975,#213976,#213977,#213978,#213979,#213980,
#213981,#213982,#213983,#213984,#213985,#213986,#213987,#213988,#213989,
#213990,#213991,#213992,#213993,#213994,#213995),.UNSPECIFIED.,.F.,.F.,
(4,2,2,2,2,2,2,2,2,2,2,2,2,2,2,2,2,2,2,2,2,2,2,2,2,2,2,2,2,2,2,4),(1.03510113506669,
1.42190076144609,1.65975570624457,1.90918310386495,2.03534477977157,2.54453754089686,
2.78186254655865,3.03265366633092,3.15880260895928,3.66811591821521,3.90937651886798,
4.15314502278736,4.27935426029102,4.78786109188973,5.01857442699673,5.24596204487806,
5.53988512633587,5.76236179365467,6.26691663031345,6.39333733948748,6.62191123077583,
6.74582667444504,6.99053079450849,7.33725916006411,7.58275600967597,7.8287822692156,
8.05831356870385,8.32996067829968,8.55807863230822,9.06599466340575,9.19223469840276,
9.21790452008223),.UNSPECIFIED.);
#30511=B_SPLINE_CURVE_WITH_KNOTS('',3,(#213999,#214000,#214001,#214002),
 .UNSPECIFIED.,.F.,.F.,(4,4),(0.,0.00054580800139321),.UNSPECIFIED.);
#30512=B_SPLINE_CURVE_WITH_KNOTS('',3,(#214004,#214005,#214006,#214007,
#214008,#214009,#214010,#214011,#214012,#214013,#214014,#214015,#214016,
#214017,#214018,#214019,#214020,#214021,#214022,#214023,#214024,#214025,
#214026,#214027,#214028,#214029,#214030,#214031,#214032,#214033),
 .UNSPECIFIED.,.F.,.F.,(4,2,2,2,2,2,2,2,2,2,2,2,2,2,4),(0.,0.16166597888304,
0.323391460359401,0.526063184698531,0.925852633976886,1.05183001043014,
1.56958669063404,1.76531286769044,1.96277562636095,2.47502393525251,2.70447577935253,
3.02961056722522,3.22205209758851,3.37599328488597,3.53032372881347),
 .UNSPECIFIED.);
#30513=B_SPLINE_CURVE_WITH_KNOTS('',3,(#214034,#214035,#214036,#214037,
#214038,#214039,#214040,#214041,#214042,#214043,#214044,#214045,#214046,
#214047,#214048,#214049,#214050,#214051,#214052,#214053,#214054,#214055,
#214056,#214057,#214058,#214059,#214060,#214061),.UNSPECIFIED.,.F.,.F.,
(4,2,2,2,2,2,2,2,2,2,2,2,2,4),(-4.0928672423958,-3.80981796722786,-3.64049485155161,
-3.12585719634299,-2.93571507444881,-2.5721796822949,-2.39990451027257,
-1.88602332766581,-1.68187581621743,-1.33960776333701,-1.16853206863454,
-0.653965815035966,-0.343366468922743,-1.00000000013978E-6),
 .UNSPECIFIED.);
#30514=B_SPLINE_CURVE_WITH_KNOTS('',3,(#214067,#214068,#214069,#214070,
#214071,#214072,#214073,#214074,#214075,#214076,#214077,#214078,#214079,
#214080,#214081,#214082,#214083,#214084,#214085,#214086,#214087,#214088,
#214089,#214090,#214091,#214092,#214093,#214094,#214095,#214096,#214097,
#214098,#214099,#214100,#214101,#214102,#214103,#214104,#214105,#214106,
#214107,#214108,#214109,#214110,#214111,#214112,#214113,#214114,#214115,
#214116,#214117,#214118,#214119,#214120,#214121,#214122,#214123,#214124,
#214125,#214126,#214127,#214128,#214129,#214130,#214131,#214132),
 .UNSPECIFIED.,.F.,.F.,(4,2,2,2,2,2,2,2,2,2,2,2,2,2,2,2,2,2,2,2,2,2,2,2,
2,2,2,2,2,2,2,2,4),(19.9501840521356,20.2039213034323,20.3287580909671,
20.5798677055414,20.8396508055159,21.0978253952488,21.2234763844211,21.4813984877127,
21.7524924853527,21.8774181480447,22.0805108449731,22.3325329071134,22.5904208234137,
22.8486507412779,22.9737051239086,23.2244367307076,23.4701290954001,23.7283594100504,
23.8533638265947,24.1041849116098,24.3531282121589,24.6113545063552,24.736519792903,
24.9870430282304,25.2253775519541,25.4575680251568,25.6291332729475,25.8870963905533,
26.1714349415304,26.2852130171025,26.6471257924219,26.7579086160256,27.092373191068),
 .UNSPECIFIED.);
#30515=B_SPLINE_CURVE_WITH_KNOTS('',3,(#214133,#214134,#214135,#214136,
#214137,#214138,#214139,#214140,#214141,#214142,#214143,#214144),
 .UNSPECIFIED.,.F.,.F.,(4,2,2,2,2,4),(4.25269675018496E-5,0.255194498557652,
0.508955632318599,0.799301344137275,0.912562061722119,1.03510113506669),
 .UNSPECIFIED.);
#30516=B_SPLINE_CURVE_WITH_KNOTS('',3,(#214145,#214146,#214147,#214148,
#214149,#214150,#214151,#214152,#214153,#214154,#214155,#214156,#214157,
#214158,#214159,#214160,#214161,#214162,#214163,#214164,#214165,#214166,
#214167,#214168,#214169,#214170,#214171,#214172,#214173,#214174,#214175,
#214176,#214177,#214178,#214179,#214180,#214181,#214182,#214183,#214184,
#214185,#214186,#214187,#214188,#214189,#214190,#214191,#214192,#214193,
#214194,#214195,#214196,#214197,#214198,#214199,#214200,#214201,#214202),
 .UNSPECIFIED.,.F.,.F.,(4,2,2,2,2,2,2,2,2,2,2,2,2,2,2,2,2,2,2,2,2,2,2,2,
2,2,2,2,4),(-12.2749063736218,-12.1187900791705,-11.879808815597,-11.5535690996991,
-11.3094012187778,-10.8019634959954,-10.6138794600607,-10.2280063491379,
-10.0105010044501,-9.68641783911147,-9.41284064170808,-8.97177822363525,
-8.76888849795534,-8.36889877677119,-8.24292592755194,-7.88568962577202,
-7.63571172501066,-7.27227457662365,-7.02175834140347,-6.65613264295677,
-6.26737152351143,-6.0766033000751,-5.57048100510707,-5.32573258363369,
-4.99778399626186,-4.71802225787336,-4.39296620626389,-4.16592791266086,
-4.0928672423958),.UNSPECIFIED.);
#30517=B_SPLINE_CURVE_WITH_KNOTS('',3,(#214207,#214208,#214209,#214210,
#214211,#214212,#214213,#214214,#214215,#214216,#214217,#214218,#214219,
#214220,#214221,#214222,#214223,#214224,#214225,#214226,#214227,#214228,
#214229,#214230,#214231,#214232,#214233,#214234,#214235,#214236,#214237,
#214238,#214239,#214240,#214241,#214242,#214243,#214244,#214245,#214246,
#214247,#214248,#214249,#214250,#214251,#214252,#214253,#214254,#214255,
#214256,#214257,#214258,#214259,#214260,#214261,#214262,#214263,#214264,
#214265,#214266,#214267,#214268,#214269,#214270,#214271,#214272,#214273,
#214274,#214275,#214276,#214277,#214278,#214279,#214280,#214281,#214282,
#214283,#214284),.UNSPECIFIED.,.F.,.F.,(4,2,2,2,2,2,2,2,2,2,2,2,2,2,2,2,
2,2,2,2,2,2,2,2,2,2,2,2,2,2,2,2,2,2,2,2,2,2,4),(11.7734600023717,11.9982362050268,
12.2288307658104,12.4791354655245,12.6044197106843,12.8626497232774,13.0985045059271,
13.3300569078068,13.5460652655509,13.7620013704151,13.9935561404502,14.2293816155567,
14.4876118366438,14.6128950196291,14.8632050686861,15.093950803072,15.3250057131515,
15.6256039597299,15.7510855597561,15.9762377203391,16.2075321392228,16.3655548549729,
16.6167748241098,16.8807332018033,17.1388659369982,17.2646851086345,17.5226540391788,
17.8073718259425,17.932474738288,18.1903879181091,18.4486148820817,18.5738163564277,
18.8242739157131,19.0602709056961,19.2920160693179,19.4572439568824,19.7150957671442,
19.9456909285047,19.9501840521356),.UNSPECIFIED.);
#30518=B_SPLINE_CURVE_WITH_KNOTS('',3,(#214286,#214287,#214288,#214289,
#214290,#214291,#214292,#214293,#214294,#214295,#214296,#214297),
 .UNSPECIFIED.,.F.,.F.,(4,2,2,2,2,4),(-13.3097623354321,-13.0506230872222,
-12.7981078626377,-12.6277703233625,-12.4570073448961,-12.2749063736218),
 .UNSPECIFIED.);
#30519=B_SPLINE_CURVE_WITH_KNOTS('',3,(#214298,#214299,#214300,#214301,
#214302,#214303,#214304,#214305,#214306,#214307,#214308,#214309,#214310,
#214311,#214312,#214313,#214314,#214315,#214316,#214317,#214318,#214319,
#214320,#214321,#214322,#214323,#214324,#214325,#214326,#214327,#214328,
#214329,#214330,#214331,#214332,#214333,#214334,#214335,#214336,#214337,
#214338,#214339,#214340,#214341,#214342,#214343,#214344,#214345,#214346,
#214347,#214348,#214349,#214350,#214351,#214352,#214353,#214354,#214355,
#214356,#214357,#214358,#214359,#214360,#214361,#214362,#214363,#214364,
#214365,#214366,#214367),.UNSPECIFIED.,.F.,.F.,(4,2,2,2,2,2,2,2,2,2,2,2,
2,2,2,2,2,2,2,2,2,2,2,2,2,2,2,2,2,2,2,2,2,2,4),(-7.14121730581807,-7.10127190196412,
-6.97635927806433,-6.76787273732327,-6.51625363264104,-6.26142709012785,
-6.00321238811012,-5.87812473396963,-5.62748345688499,-5.38451315576289,
-5.12629705305085,-5.00144012143128,-4.75039183957789,-4.49242993202835,
-4.23425457712158,-4.10868711407363,-3.85079913174379,-3.58528178243477,
-3.34048377236277,-3.08998645698157,-2.96416702950007,-2.67402819920963,
-2.548826428631,-2.29286226189582,-2.03468181880128,-1.90920364004217,-1.65134503451085,
-1.41375102191269,-1.15556492024653,-1.03016186674223,-0.772326080524892,
-0.538863998804044,-0.273114657421419,-0.137051040303161,-6.79217266545488E-5),
 .UNSPECIFIED.);
#30520=B_SPLINE_CURVE_WITH_KNOTS('',3,(#214372,#214373,#214374,#214375,
#214376,#214377,#214378,#214379,#214380,#214381,#214382,#214383,#214384,
#214385,#214386,#214387,#214388,#214389,#214390,#214391,#214392,#214393,
#214394,#214395,#214396,#214397,#214398,#214399,#214400,#214401,#214402,
#214403,#214404,#214405,#214406,#214407,#214408,#214409,#214410,#214411,
#214412,#214413,#214414,#214415,#214416,#214417,#214418,#214419,#214420,
#214421,#214422,#214423,#214424,#214425,#214426,#214427,#214428,#214429,
#214430,#214431,#214432,#214433,#214434,#214435,#214436,#214437,#214438,
#214439,#214440,#214441,#214442,#214443,#214444,#214445,#214446,#214447,
#214448,#214449),.UNSPECIFIED.,.F.,.F.,(4,2,2,2,2,2,2,2,2,2,2,2,2,2,2,2,
2,2,2,2,2,2,2,2,2,2,2,2,2,2,2,2,2,2,2,2,2,2,4),(3.59637852778132,3.77812667911342,
4.02304674635722,4.29062104873451,4.54852148405871,4.67411990136732,4.93229550742404,
5.17248737133136,5.43037080611408,5.55589702810278,5.81408617301148,6.07101155670248,
6.32203927006553,6.44691570930367,6.70513880893479,6.95581693593773,7.08095057279958,
7.36746835221977,7.62543238824665,7.79735490426262,7.92350791987667,8.29187981987286,
8.41683743990179,8.69138966599333,8.94932139764217,9.07501539189821,9.33317961110474,
9.59405572704114,9.71924899120621,10.0085573244635,10.2394175420354,10.4671044593678,
10.5924380553917,10.8877072565187,11.1186536449452,11.341727853923,11.4671925064493,
11.7671943111698,11.7734600023717),.UNSPECIFIED.);
#30521=B_SPLINE_CURVE_WITH_KNOTS('',3,(#214450,#214451,#214452,#214453,
#214454,#214455,#214456,#214457,#214458,#214459,#214460,#214461,#214462,
#214463,#214464,#214465,#214466,#214467,#214468,#214469,#214470,#214471,
#214472,#214473,#214474,#214475,#214476,#214477,#214478,#214479,#214480,
#214481,#214482,#214483,#214484,#214485,#214486,#214487,#214488,#214489,
#214490,#214491,#214492,#214493,#214494,#214495,#214496,#214497,#214498,
#214499,#214500,#214501,#214502,#214503,#214504,#214505,#214506,#214507,
#214508,#214509,#214510,#214511,#214512,#214513,#214514,#214515,#214516,
#214517,#214518,#214519,#214520,#214521,#214522,#214523,#214524,#214525),
 .UNSPECIFIED.,.F.,.F.,(4,2,2,2,2,2,2,2,2,2,2,2,2,2,2,2,2,2,2,2,2,2,2,2,
2,2,2,2,2,2,2,2,2,2,2,2,2,4),(-15.3176231869007,-15.1056438788204,-14.8722725390337,
-14.614416732992,-14.489000008823,-14.2307975543113,-13.9931480555956,-13.7617417105088,
-13.5448308438595,-13.3285120238497,-13.097092852516,-12.8596333519296,
-12.6014293942186,-12.47602821334,-12.218176957919,-11.9856359912747,-11.7274146784205,
-11.602410922309,-11.3516073204166,-11.1029728045464,-10.8447546918672,
-10.7196093690404,-10.4690670570721,-10.2297511991479,-9.99732467670149,
-9.82281327047037,-9.56481527159159,-9.26273929783766,-9.1372175261113,
-8.90657656378107,-8.6483608703652,-8.52352688836427,-8.27244061302118,
-8.01300493924838,-7.75484111316192,-7.62921200516085,-7.37130846105036,
-7.14121730581807),.UNSPECIFIED.);
#30522=B_SPLINE_CURVE_WITH_KNOTS('',3,(#214531,#214532,#214533,#214534,
#214535,#214536,#214537,#214538,#214539,#214540,#214541,#214542,#214543,
#214544,#214545,#214546,#214547,#214548,#214549,#214550,#214551,#214552,
#214553,#214554,#214555,#214556,#214557,#214558,#214559,#214560,#214561,
#214562,#214563,#214564,#214565,#214566,#214567,#214568,#214569,#214570,
#214571,#214572,#214573,#214574,#214575,#214576),.UNSPECIFIED.,.F.,.F.,
(4,2,2,2,2,2,2,2,2,2,2,2,2,2,2,2,2,2,2,2,2,2,4),(-27.0906254788674,-26.9501859108409,
-26.8108374409825,-26.5377652063263,-26.314814384877,-26.2047766401236,
-25.8436700170918,-25.7187168828716,-25.4433658352626,-25.1854571453625,
-25.0155712252688,-24.8894553916724,-24.5219127449176,-24.3969666928096,
-24.1223476036517,-23.891498454964,-23.671986020183,-23.4378392902655,-23.2579366145597,
-23.1316996181331,-22.7603654578437,-22.6354219479875,-22.5104081169932),
 .UNSPECIFIED.);
#30523=B_SPLINE_CURVE_WITH_KNOTS('',3,(#214577,#214578,#214579,#214580,
#214581,#214582,#214583,#214584,#214585,#214586,#214587,#214588,#214589,
#214590,#214591,#214592,#214593,#214594,#214595,#214596,#214597,#214598,
#214599,#214600,#214601,#214602,#214603,#214604,#214605,#214606,#214607,
#214608,#214609,#214610,#214611,#214612),.UNSPECIFIED.,.F.,.F.,(4,2,2,2,
2,2,2,2,2,2,2,2,2,2,2,2,2,4),(6.63670101017275E-6,0.255164148591463,0.5026236995069,
0.769207716988034,1.02708819460434,1.19522482133063,1.42721465689468,1.68501797683759,
1.80999390851426,2.08699717987714,2.21271380182159,2.46280904639482,2.70750797272155,
2.97099701514689,3.09660781343983,3.40130864969258,3.52723844382287,3.59637852778132),
 .UNSPECIFIED.);
#30524=B_SPLINE_CURVE_WITH_KNOTS('',3,(#214613,#214614,#214615,#214616,
#214617,#214618,#214619,#214620,#214621,#214622,#214623,#214624,#214625,
#214626,#214627,#214628,#214629,#214630,#214631,#214632,#214633,#214634,
#214635,#214636,#214637,#214638,#214639,#214640,#214641,#214642,#214643,
#214644,#214645,#214646,#214647,#214648,#214649,#214650,#214651,#214652,
#214653,#214654,#214655,#214656,#214657,#214658,#214659,#214660,#214661,
#214662,#214663,#214664,#214665,#214666,#214667,#214668,#214669,#214670,
#214671,#214672,#214673,#214674,#214675,#214676,#214677,#214678,#214679,
#214680,#214681,#214682,#214683,#214684,#214685,#214686,#214687,#214688,
#214689,#214690,#214691,#214692),.UNSPECIFIED.,.F.,.F.,(4,2,2,2,2,2,2,2,
2,2,2,2,2,2,2,2,2,2,2,2,2,2,2,2,2,2,2,2,2,2,2,2,2,2,2,2,2,2,2,4),(-23.4938196648925,
-23.4149340907595,-23.2518796395597,-23.0202919717034,-22.7851614155846,
-22.5347413007983,-22.4095333736385,-22.1513199685413,-21.9013907117378,
-21.6505529411977,-21.5255691067719,-21.2673495098011,-21.0094825445456,
-20.7573720460851,-20.5557484524118,-20.4308259828129,-20.1594536607042,
-19.901541807629,-19.7758924762591,-19.5177299337117,-19.2578655533035,
-19.0067644829067,-18.8819345614844,-18.6237154355237,-18.3813050082189,
-18.1306759018197,-18.0055771756941,-17.7473595214231,-17.5137027493023,
-17.2558477942795,-17.1304271894833,-16.8722273623606,-16.6177156880087,
-16.3667526914773,-16.2418387291235,-15.9836170256549,-15.7396157516227,
-15.4889398935453,-15.3638642493586,-15.3176231869007),.UNSPECIFIED.);
#30525=B_SPLINE_CURVE_WITH_KNOTS('',3,(#214697,#214698,#214699,#214700,
#214701,#214702,#214703,#214704,#214705,#214706,#214707,#214708,#214709,
#214710,#214711,#214712,#214713,#214714,#214715,#214716,#214717,#214718,
#214719,#214720,#214721,#214722,#214723,#214724,#214725,#214726,#214727,
#214728,#214729,#214730,#214731,#214732,#214733,#214734,#214735,#214736,
#214737,#214738,#214739,#214740,#214741,#214742,#214743,#214744,#214745,
#214746,#214747,#214748,#214749,#214750,#214751,#214752,#214753,#214754,
#214755,#214756,#214757,#214758,#214759,#214760,#214761,#214762,#214763,
#214764,#214765,#214766,#214767,#214768,#214769,#214770,#214771,#214772,
#214773,#214774),.UNSPECIFIED.,.F.,.F.,(4,2,2,2,2,2,2,2,2,2,2,2,2,2,2,2,
2,2,2,2,2,2,2,2,2,2,2,2,2,2,2,2,2,2,2,2,2,2,4),(-22.5104081169932,-22.3612307693209,
-22.2355377097177,-21.9285413116893,-21.8025981562684,-21.551656587909,
-21.306722143075,-21.0388457213177,-20.7809474596957,-20.6553456671694,
-20.397175432749,-20.1384391189269,-19.8873687315545,-19.7625221501105,
-19.5043045239689,-19.2615640724446,-19.0109272243863,-18.8858343260698,
-18.6276181991213,-18.3800459105684,-18.1292740488693,-18.0042546680597,
-17.7460368060689,-17.4881657987609,-17.236111325147,-17.0336800623867,
-16.9087594766789,-16.6375496402009,-16.3796396281236,-16.2539930447797,
-15.9958313522177,-15.7360196781561,-15.4849211969179,-15.3600911092144,
-15.1018732790179,-14.8712963732557,-14.6134571162699,-14.4880912198269,
-14.334025337542),.UNSPECIFIED.);
#30526=B_SPLINE_CURVE_WITH_KNOTS('',3,(#214776,#214777,#214778,#214779,
#214780,#214781,#214782,#214783,#214784,#214785,#214786,#214787,#214788,
#214789,#214790,#214791,#214792,#214793,#214794,#214795,#214796,#214797,
#214798,#214799,#214800,#214801,#214802,#214803,#214804,#214805,#214806,
#214807,#214808,#214809,#214810,#214811),.UNSPECIFIED.,.F.,.F.,(4,2,2,2,
2,2,2,2,2,2,2,2,2,2,2,2,2,4),(-27.089958399627,-26.952979419026,-26.8169785957911,
-26.5513613453522,-26.3745643085782,-26.1163666107755,-25.87887336021,-25.647399127963,
-25.431082688021,-25.1956028474001,-25.0178025030768,-24.7851132908777,
-24.5557298449793,-24.2978969360107,-24.1329631967999,-23.9012495356808,
-23.6653755408411,-23.4938196648925),.UNSPECIFIED.);
#30527=B_SPLINE_CURVE_WITH_KNOTS('',3,(#214812,#214813,#214814,#214815,
#214816,#214817,#214818,#214819,#214820,#214821,#214822,#214823,#214824,
#214825,#214826,#214827,#214828,#214829,#214830,#214831,#214832,#214833,
#214834,#214835,#214836,#214837,#214838,#214839,#214840,#214841,#214842,
#214843,#214844,#214845,#214846,#214847,#214848,#214849,#214850,#214851,
#214852,#214853,#214854,#214855,#214856,#214857),.UNSPECIFIED.,.F.,.F.,
(4,2,2,2,2,2,2,2,2,2,2,2,2,2,2,2,2,2,2,2,2,2,4),(-4.5795509234186,-4.50984625011772,
-4.27825488944027,-4.1149876509827,-3.86459297117082,-3.62991131288588,
-3.39840441911819,-3.23643616951018,-2.98583978245699,-2.74413559559504,
-2.48592991455161,-2.36114402600808,-2.10999536200624,-1.84777195661155,
-1.589644744617,-1.46390699951972,-1.20598373740661,-0.927127338164872,
-0.812594909757223,-0.606764161622401,-0.304527926094519,-0.153020088801399,
-3.84812749945382E-6),.UNSPECIFIED.);
#30528=B_SPLINE_CURVE_WITH_KNOTS('',3,(#214862,#214863,#214864,#214865,
#214866,#214867,#214868,#214869,#214870,#214871,#214872,#214873,#214874,
#214875,#214876,#214877,#214878,#214879,#214880,#214881,#214882,#214883,
#214884,#214885,#214886,#214887,#214888,#214889,#214890,#214891,#214892,
#214893,#214894,#214895,#214896,#214897,#214898,#214899,#214900,#214901,
#214902,#214903,#214904,#214905,#214906,#214907,#214908,#214909,#214910,
#214911,#214912,#214913,#214914,#214915,#214916,#214917,#214918,#214919,
#214920,#214921,#214922,#214923,#214924,#214925,#214926,#214927,#214928,
#214929,#214930,#214931,#214932,#214933,#214934,#214935,#214936,#214937,
#214938,#214939),.UNSPECIFIED.,.F.,.F.,(4,2,2,2,2,2,2,2,2,2,2,2,2,2,2,2,
2,2,2,2,2,2,2,2,2,2,2,2,2,2,2,2,2,2,2,2,2,2,4),(-14.334025337542,-14.2298880752575,
-13.9928889355398,-13.7614412675403,-13.5452357011143,-13.3285719908861,
-13.0971354937459,-12.8599793321159,-12.601777163161,-12.4764005548312,
-12.2185590226874,-11.9873142271819,-11.7290963947761,-11.6042075960275,
-11.3532104274166,-11.0972543394135,-10.8390648910172,-10.7135831106281,
-10.4557157588316,-10.2181940081271,-9.95999746144929,-9.83459447204947,
-9.57674878778774,-9.34391585468663,-9.08570178135842,-8.96067581182445,
-8.70992487595289,-8.4629645160084,-8.20475120064606,-8.07969125810166,
-7.82900251582835,-7.58427333026132,-7.32605897513911,-7.201111763903,-6.95022163718091,
-6.69815316779949,-6.43995054050984,-6.31464537487433,-6.15788331278694),
 .UNSPECIFIED.);
#30529=B_SPLINE_CURVE_WITH_KNOTS('',3,(#214940,#214941,#214942,#214943,
#214944,#214945,#214946,#214947,#214948,#214949,#214950,#214951,#214952,
#214953,#214954,#214955,#214956,#214957,#214958,#214959,#214960,#214961,
#214962,#214963,#214964,#214965,#214966,#214967,#214968,#214969,#214970,
#214971,#214972,#214973,#214974,#214975,#214976,#214977,#214978,#214979,
#214980,#214981,#214982,#214983,#214984,#214985,#214986,#214987,#214988,
#214989,#214990,#214991,#214992,#214993,#214994,#214995,#214996,#214997,
#214998,#214999,#215000,#215001,#215002,#215003,#215004,#215005,#215006,
#215007,#215008,#215009,#215010,#215011,#215012,#215013,#215014,#215015,
#215016,#215017),.UNSPECIFIED.,.F.,.F.,(4,2,2,2,2,2,2,2,2,2,2,2,2,2,2,2,
2,2,2,2,2,2,2,2,2,2,2,2,2,2,2,2,2,2,2,2,2,2,4),(-12.7553010434687,-12.6016556768374,
-12.4763182694624,-12.218491551322,-11.9892784696402,-11.7566700395306,
-11.5797800311709,-11.3436395338856,-11.1265836305225,-10.895209493342,
-10.6572556971099,-10.3990679449927,-10.2736349244766,-10.0157862458109,
-9.78103815707203,-9.52283394508956,-9.39765070502228,-9.14720450848217,
-8.91082671304611,-8.67902923702854,-8.51277037102089,-8.25492183080519,
-8.01981155397926,-7.76161037628427,-7.63639857901851,-7.38601142426069,
-7.15160657277073,-6.9201416220309,-6.75884469323388,-6.50814457860648,
-6.26276625595113,-6.00455921046281,-5.87958199057688,-5.62875764298286,
-5.37886593938861,-5.12066465996931,-4.99546505972988,-4.74505487654086,
-4.5795509234186),.UNSPECIFIED.);
#30530=B_SPLINE_CURVE_WITH_KNOTS('',3,(#215026,#215027,#215028,#215029,
#215030,#215031),.UNSPECIFIED.,.F.,.F.,(4,2,4),(1.00000001154634E-6,0.291982877240899,
0.583963182531403),.UNSPECIFIED.);
#30531=B_SPLINE_CURVE_WITH_KNOTS('',3,(#215035,#215036,#215037,#215038,
#215039,#215040),.UNSPECIFIED.,.F.,.F.,(4,2,4),(1.18860081512343E-5,0.292247563585459,
0.584494052040958),.UNSPECIFIED.);
#30532=B_SPLINE_CURVE_WITH_KNOTS('',3,(#215044,#215045,#215046,#215047,
#215048,#215049,#215050,#215051,#215052,#215053,#215054,#215055,#215056,
#215057,#215058,#215059,#215060,#215061,#215062,#215063,#215064,#215065,
#215066,#215067,#215068,#215069,#215070,#215071,#215072,#215073,#215074,
#215075,#215076,#215077,#215078,#215079,#215080,#215081,#215082,#215083,
#215084,#215085,#215086,#215087,#215088,#215089,#215090,#215091,#215092,
#215093,#215094,#215095,#215096,#215097,#215098,#215099,#215100,#215101,
#215102,#215103),.UNSPECIFIED.,.F.,.F.,(4,2,2,2,2,2,2,2,2,2,2,2,2,2,2,2,
2,2,2,2,2,2,2,2,2,2,2,2,2,4),(-27.0887410610092,-26.9511925330194,-26.8146181657615,
-26.5477430484365,-26.3703867926432,-26.1121969470036,-25.8619181368252,
-25.61109070341,-25.486127317508,-25.2279323061975,-24.9957522036846,-24.7379286430516,
-24.6125451134737,-24.3543677958648,-24.1004364568259,-23.9752344396555,
-23.6847558007391,-23.4539116075989,-23.2606464300677,-23.1342701225633,
-22.7584338658159,-22.633498574235,-22.3598177762354,-22.1019137699259,
-21.9762419243061,-21.7181016904069,-21.4575171051022,-21.2064122614871,
-21.0816012437997,-20.9311220871695),.UNSPECIFIED.);
#30533=B_SPLINE_CURVE_WITH_KNOTS('',3,(#215104,#215105,#215106,#215107,
#215108,#215109,#215110,#215111,#215112,#215113,#215114,#215115,#215116,
#215117),.UNSPECIFIED.,.F.,.F.,(4,2,2,2,2,2,4),(0.,0.254132792260232,0.504072118513429,
1.01015766536903,1.26037994975016,1.64270580735333,2.01988313929097),
 .UNSPECIFIED.);
#30534=B_SPLINE_CURVE_WITH_KNOTS('',3,(#215122,#215123,#215124,#215125),
 .UNSPECIFIED.,.F.,.F.,(4,4),(-0.00220042394831986,0.),.UNSPECIFIED.);
#30535=B_SPLINE_CURVE_WITH_KNOTS('',3,(#215127,#215128,#215129,#215130,
#215131,#215132,#215133,#215134,#215135,#215136,#215137,#215138,#215139,
#215140,#215141,#215142,#215143,#215144,#215145,#215146,#215147,#215148,
#215149,#215150,#215151,#215152,#215153,#215154,#215155,#215156,#215157,
#215158,#215159,#215160,#215161,#215162,#215163,#215164,#215165,#215166,
#215167,#215168,#215169,#215170,#215171,#215172),.UNSPECIFIED.,.F.,.F.,
(4,2,2,2,2,2,2,2,2,2,2,2,2,2,2,2,2,2,2,2,2,2,4),(3.77495847628064E-5,0.239786601820375,
0.486605707252922,0.970538667060806,1.45703768164762,1.71085426685665,1.9510783074637,
2.07349206054796,2.55160936918131,2.80110529120643,3.03699522422359,3.28275824999043,
3.52002970929651,3.76617821420921,4.00121882590256,4.49262572156428,4.61272242555652,
4.85423743097051,5.08785380877439,5.57193736666521,6.05829820485534,6.18384427890247,
6.56939833044695),.UNSPECIFIED.);
#30536=B_SPLINE_CURVE_WITH_KNOTS('',3,(#215175,#215176,#215177,#215178,
#215179,#215180,#215181,#215182,#215183,#215184,#215185,#215186,#215187,
#215188,#215189,#215190,#215191,#215192,#215193,#215194,#215195,#215196,
#215197,#215198,#215199,#215200,#215201,#215202,#215203,#215204,#215205,
#215206,#215207,#215208,#215209,#215210,#215211,#215212,#215213,#215214,
#215215,#215216,#215217,#215218,#215219,#215220,#215221,#215222,#215223,
#215224,#215225,#215226,#215227,#215228,#215229,#215230,#215231,#215232),
 .UNSPECIFIED.,.F.,.F.,(4,3,3,3,3,3,3,3,3,3,3,3,3,3,3,3,3,3,3,4),(0.,0.0577023232573194,
0.115555621115559,0.173492165360459,0.231551782116688,0.25,0.307569756346389,
0.36507578732566,0.422538236883637,0.479957516807691,0.537334036195806,
0.594651018367979,0.651929822767017,0.709155453145963,0.75,0.807257177143259,
0.864351407537752,0.921347999937229,0.97820765935611,0.999999816562462),
 .UNSPECIFIED.);
#30537=B_SPLINE_CURVE_WITH_KNOTS('',3,(#215238,#215239,#215240,#215241),
 .UNSPECIFIED.,.F.,.F.,(4,4),(-6.83645233358743E-6,-1.00000001751477E-6),
 .UNSPECIFIED.);
#30538=B_SPLINE_CURVE_WITH_KNOTS('',3,(#215243,#215244,#215245,#215246,
#215247,#215248,#215249,#215250,#215251,#215252,#215253,#215254),
 .UNSPECIFIED.,.F.,.F.,(4,2,2,2,2,4),(0.000339869836819791,0.29675202029107,
0.394471814058443,0.493164400823471,0.639110988050242,0.788070724201746),
 .UNSPECIFIED.);
#30539=B_SPLINE_CURVE_WITH_KNOTS('',3,(#215257,#215258,#215259,#215260,
#215261,#215262,#215263,#215264,#215265,#215266,#215267,#215268),
 .UNSPECIFIED.,.F.,.F.,(4,2,2,2,2,4),(-0.787810247908823,-0.491424601923884,
-0.393707156561869,-0.295035291842161,-0.149115943288589,-9.76537854817782E-5),
 .UNSPECIFIED.);
#30540=B_SPLINE_CURVE_WITH_KNOTS('',3,(#215271,#215272,#215273,#215274,
#215275,#215276,#215277,#215278,#215279,#215280,#215281,#215282,#215283,
#215284,#215285,#215286,#215287,#215288,#215289,#215290,#215291,#215292,
#215293,#215294,#215295,#215296,#215297,#215298,#215299,#215300,#215301,
#215302,#215303,#215304,#215305,#215306,#215307,#215308,#215309,#215310,
#215311,#215312,#215313,#215314,#215315,#215316,#215317,#215318,#215319,
#215320,#215321,#215322,#215323,#215324,#215325,#215326,#215327,#215328,
#215329,#215330,#215331,#215332,#215333,#215334,#215335,#215336,#215337,
#215338,#215339,#215340),.UNSPECIFIED.,.F.,.F.,(4,2,2,2,2,2,2,2,2,2,2,2,
2,2,2,2,2,2,2,2,2,2,2,2,2,2,2,2,2,2,2,2,2,2,4),(-20.0196235340061,-19.8157278920515,
-19.6158545518425,-19.4425763978127,-19.2852028557817,-19.1959685061364,
-19.0203362825393,-18.8728424835519,-18.7345184196789,-18.5651733062971,
-18.3584086465096,-18.1897342242108,-18.1009133571369,-17.9231088860798,
-17.7687386604926,-17.6127844006329,-17.4523655002313,-17.3638013379125,
-17.1842840455061,-17.0221648541842,-16.9027716802059,-16.7343479146783,
-16.5301402266849,-16.3682944213952,-16.1638372797701,-16.0746707278444,
-15.9189413862097,-15.8312910721691,-15.5641446602286,-15.3837526745358,
-15.2039523974867,-15.0498956541389,-14.9618693672449,-14.6038541971235,
-14.2994391167293),.UNSPECIFIED.);
#30541=B_SPLINE_CURVE_WITH_KNOTS('',3,(#215343,#215344,#215345,#215346,
#215347,#215348,#215349,#215350,#215351,#215352,#215353,#215354,#215355,
#215356,#215357,#215358,#215359,#215360,#215361,#215362,#215363,#215364,
#215365,#215366,#215367,#215368,#215369,#215370,#215371,#215372,#215373,
#215374,#215375,#215376,#215377,#215378,#215379,#215380,#215381,#215382,
#215383,#215384,#215385,#215386,#215387,#215388,#215389,#215390,#215391,
#215392,#215393,#215394,#215395,#215396,#215397,#215398,#215399,#215400,
#215401,#215402,#215403,#215404,#215405,#215406,#215407,#215408,#215409,
#215410),.UNSPECIFIED.,.F.,.F.,(4,2,2,2,2,2,2,2,2,2,2,2,2,2,2,2,2,2,2,2,
2,2,2,2,2,2,2,2,2,2,2,2,2,4),(-5.72098192612602,-5.4140289061323,-5.056101730372,
-4.96798087881037,-4.819769206694,-4.54633567752282,-4.37277702978704,-4.20554432130538,
-4.0478229434517,-3.91343223942507,-3.5963260817461,-3.50785527543515,-3.35735778939112,
-3.20580694022997,-3.02615489172175,-2.84949295160721,-2.76019692805457,
-2.56673230648565,-2.40566688978276,-2.2464078740048,-2.09440523942289,
-1.91421338925738,-1.73650461422533,-1.55941996019895,-1.47033771435364,
-1.31006776518604,-1.14767795859055,-0.999884460342694,-0.824207561520106,
-0.734963617853822,-0.578056733648994,-0.420047611278566,-0.211187702725621,
-6.83645233358743E-6),.UNSPECIFIED.);
#30542=B_SPLINE_CURVE_WITH_KNOTS('',3,(#215415,#215416,#215417,#215418,
#215419,#215420,#215421,#215422,#215423,#215424,#215425,#215426,#215427,
#215428,#215429,#215430,#215431,#215432,#215433,#215434,#215435,#215436,
#215437,#215438,#215439,#215440,#215441,#215442,#215443,#215444,#215445,
#215446,#215447,#215448,#215449,#215450,#215451,#215452,#215453,#215454,
#215455,#215456,#215457,#215458,#215459,#215460,#215461,#215462,#215463,
#215464,#215465,#215466,#215467,#215468,#215469,#215470,#215471,#215472,
#215473,#215474,#215475,#215476,#215477,#215478,#215479,#215480,#215481,
#215482,#215483,#215484,#215485,#215486),.UNSPECIFIED.,.F.,.F.,(4,2,2,2,
2,2,2,2,2,2,2,2,2,2,2,2,2,2,2,2,2,2,2,2,2,2,2,2,2,2,2,2,2,2,2,4),(-11.4412093673078,
-11.338051198562,-11.1891609467898,-11.1010562826919,-10.7866246366731,
-10.6066561084781,-10.4268423987289,-10.2467065997548,-10.098678538798,
-10.0105929109292,-9.65463874041737,-9.48052854819771,-9.31002440202757,
-9.13918288304346,-8.98055225874758,-8.82546188245068,-8.67973574012756,
-8.49997454609656,-8.41152390733726,-8.24811344358312,-8.07358642266137,
-7.92464560938184,-7.70469009445336,-7.55442719254641,-7.35785242194359,
-7.20795195047273,-6.90068692991203,-6.81290801551602,-6.64908308538578,
-6.49018627923697,-6.31439124792872,-6.22502211673781,-6.07787970006461,
-5.9211138364368,-5.76964709342306,-5.72098192612602),.UNSPECIFIED.);
#30543=B_SPLINE_CURVE_WITH_KNOTS('',3,(#215487,#215488,#215489,#215490,
#215491,#215492,#215493,#215494,#215495,#215496,#215497,#215498,#215499,
#215500,#215501,#215502,#215503,#215504,#215505,#215506,#215507,#215508,
#215509,#215510,#215511,#215512,#215513,#215514,#215515,#215516,#215517,
#215518,#215519,#215520,#215521,#215522,#215523,#215524,#215525,#215526,
#215527,#215528,#215529,#215530,#215531,#215532,#215533,#215534,#215535,
#215536,#215537,#215538,#215539,#215540,#215541,#215542,#215543,#215544,
#215545,#215546,#215547,#215548,#215549,#215550,#215551,#215552,#215553,
#215554,#215555,#215556,#215557,#215558,#215559,#215560),.UNSPECIFIED.,
 .F.,.F.,(4,2,2,2,2,2,2,2,2,2,2,2,2,2,2,2,2,2,2,2,2,2,2,2,2,2,2,2,2,2,2,
2,2,2,2,2,4),(-14.2994391167293,-14.2477501603601,-14.0678479146357,-13.892033039284,
-13.7449994332337,-13.5933261734264,-13.4364967134449,-13.3472472844073,
-13.1713477116733,-12.9929134291802,-12.8495266728997,-12.6946660563486,
-12.50714685734,-12.3408887659613,-12.2520944775663,-12.0738427041846,-11.9100950504764,
-11.762543263869,-11.6043231736101,-11.5157857281393,-11.3361551841859,
-11.1826312112805,-11.0366836994984,-10.8800924293092,-10.709523970501,
-10.5391611197758,-10.3652159760863,-10.0092725080805,-9.92114808123932,
-9.76123299805315,-9.58102608277333,-9.38455674435135,-9.20446141623579,
-9.04465508227102,-8.77152473193952,-8.59818150590377,-8.58008361725819),
 .UNSPECIFIED.);
#30544=B_SPLINE_CURVE_WITH_KNOTS('',3,(#215565,#215566,#215567,#215568,
#215569,#215570,#215571,#215572,#215573,#215574,#215575,#215576,#215577,
#215578,#215579,#215580,#215581,#215582,#215583,#215584,#215585,#215586,
#215587,#215588,#215589,#215590,#215591,#215592,#215593,#215594,#215595,
#215596,#215597,#215598,#215599,#215600,#215601,#215602,#215603,#215604,
#215605,#215606,#215607,#215608,#215609,#215610,#215611,#215612,#215613,
#215614,#215615,#215616,#215617,#215618,#215619,#215620,#215621,#215622,
#215623,#215624,#215625,#215626,#215627,#215628,#215629,#215630,#215631,
#215632,#215633,#215634),.UNSPECIFIED.,.F.,.F.,(4,2,2,2,2,2,2,2,2,2,2,2,
2,2,2,2,2,2,2,2,2,2,2,2,2,2,2,2,2,2,2,2,2,2,4),(-17.1619514598514,-17.0707998436542,
-16.9045145666629,-16.7309852587693,-16.4586010792192,-16.309900328499,
-16.221783342895,-15.8639724075797,-15.5085207792211,-15.355192371691,-15.2006223540609,
-15.0529932168943,-14.9636273693785,-14.7878315671842,-14.6292399631429,
-14.4801068549128,-14.3234633590855,-14.1304499920554,-13.9645679910772,
-13.8756157382424,-13.6982985297934,-13.5306753108811,-13.3696744824731,
-13.2167356928649,-13.0331390496967,-12.868276309184,-12.6976058536657,
-12.5270153994763,-12.3098536115514,-12.144439553079,-12.0660876907221,
-11.9201930773019,-11.8318736328062,-11.5176804116582,-11.4412093673078),
 .UNSPECIFIED.);
#30545=B_SPLINE_CURVE_WITH_KNOTS('',3,(#215635,#215636,#215637,#215638,
#215639,#215640,#215641,#215642,#215643,#215644,#215645,#215646,#215647,
#215648,#215649,#215650,#215651,#215652,#215653,#215654,#215655,#215656,
#215657,#215658,#215659,#215660,#215661,#215662,#215663,#215664,#215665,
#215666,#215667,#215668,#215669,#215670,#215671,#215672,#215673,#215674,
#215675,#215676,#215677,#215678,#215679,#215680,#215681,#215682,#215683,
#215684,#215685,#215686,#215687,#215688,#215689,#215690,#215691,#215692,
#215693,#215694,#215695,#215696,#215697,#215698,#215699,#215700,#215701,
#215702,#215703,#215704,#215705,#215706),.UNSPECIFIED.,.F.,.F.,(4,2,2,2,
2,2,2,2,2,2,2,2,2,2,2,2,2,2,2,2,2,2,2,2,2,2,2,2,2,2,2,2,2,2,2,4),(-8.58008361725819,
-8.4286097990283,-8.26279364651665,-8.12156683079037,-7.91613144710299,
-7.7770878294328,-7.60612693118763,-7.51786059374663,-7.355334811172,-7.17383932316611,
-7.02447968816001,-6.83757625395707,-6.68626101237962,-6.50602979938285,
-6.32854906868142,-6.15109686754141,-6.06207677134911,-5.90122486412687,
-5.73980986202818,-5.59047106699529,-5.41469586981278,-5.32548902221139,
-5.16583815293916,-4.98252592676009,-4.84153082561947,-4.61168690966548,
-4.47290134245129,-4.25386145852119,-4.12105436091202,-3.80495585716246,
-3.71697908525877,-3.56653413552749,-3.29029346081404,-3.1165390136774,
-2.94720715469032,-2.86068452297866),.UNSPECIFIED.);
#30546=B_SPLINE_CURVE_WITH_KNOTS('',3,(#215712,#215713,#215714,#215715),
 .UNSPECIFIED.,.F.,.F.,(4,4),(-9.10624732692347E-6,-9.99999999714383E-7),
 .UNSPECIFIED.);
#30547=B_SPLINE_CURVE_WITH_KNOTS('',3,(#215717,#215718,#215719,#215720,
#215721,#215722,#215723,#215724),.UNSPECIFIED.,.F.,.F.,(4,2,2,4),(0.000264654385577618,
0.197179255479982,0.294830977384805,0.393932741177781),.UNSPECIFIED.);
#30548=B_SPLINE_CURVE_WITH_KNOTS('',3,(#215727,#215728,#215729,#215730,
#215731,#215732,#215733,#215734),.UNSPECIFIED.,.F.,.F.,(4,2,2,4),(-0.393859367022616,
-0.195155498856749,-0.0984062562737634,-0.000187054781780563),
 .UNSPECIFIED.);
#30549=B_SPLINE_CURVE_WITH_KNOTS('',3,(#215737,#215738,#215739,#215740,
#215741,#215742,#215743,#215744,#215745,#215746,#215747,#215748,#215749,
#215750,#215751,#215752,#215753,#215754,#215755,#215756,#215757,#215758,
#215759,#215760,#215761,#215762,#215763,#215764,#215765,#215766,#215767,
#215768,#215769,#215770,#215771,#215772,#215773,#215774,#215775,#215776,
#215777,#215778,#215779,#215780,#215781,#215782,#215783,#215784,#215785,
#215786,#215787,#215788,#215789,#215790,#215791,#215792,#215793,#215794,
#215795,#215796,#215797,#215798,#215799,#215800,#215801,#215802),
 .UNSPECIFIED.,.F.,.F.,(4,2,2,2,2,2,2,2,2,2,2,2,2,2,2,2,2,2,2,2,2,2,2,2,
2,2,2,2,2,2,2,2,4),(-20.0265413516697,-19.7916844706762,-19.5590662266383,
-19.4024008232342,-19.256032447578,-19.166686445916,-18.9909052667409,-18.8210922306707,
-18.6737831612299,-18.521576051052,-18.3315039514708,-18.1668536215511,
-17.995500173617,-17.8256557704653,-17.609225679366,-17.4395698378931,-17.3509823357291,
-17.1723670573172,-17.0230846436569,-16.8620577093886,-16.7023795041317,
-16.5322074361327,-16.3618316254644,-16.1883018411768,-15.8329332221974,
-15.5336648716409,-15.4458799425158,-15.1745299152678,-14.9941718872728,
-14.8143733476338,-14.6613652206745,-14.5733584986169,-14.3060169149355),
 .UNSPECIFIED.);
#30550=B_SPLINE_CURVE_WITH_KNOTS('',3,(#215805,#215806,#215807,#215808,
#215809,#215810,#215811,#215812,#215813,#215814,#215815,#215816,#215817,
#215818,#215819,#215820,#215821,#215822,#215823,#215824,#215825,#215826,
#215827,#215828,#215829,#215830,#215831,#215832,#215833,#215834,#215835,
#215836,#215837,#215838,#215839,#215840,#215841,#215842,#215843,#215844,
#215845,#215846,#215847,#215848,#215849,#215850,#215851,#215852,#215853,
#215854,#215855,#215856,#215857,#215858,#215859,#215860,#215861,#215862,
#215863,#215864,#215865,#215866,#215867,#215868,#215869,#215870,#215871,
#215872,#215873,#215874),.UNSPECIFIED.,.F.,.F.,(4,2,2,2,2,2,2,2,2,2,2,2,
2,2,2,2,2,2,2,2,2,2,2,2,2,2,2,2,2,2,2,2,2,2,4),(-5.72061718523155,-5.45327902906014,
-5.36526221058928,-5.21232654173221,-4.94148501082312,-4.76805599127904,
-4.60257504126808,-4.45597704073809,-4.27635443196831,-4.11908377830053,
-3.82844746279641,-3.47270207454062,-3.29904824307419,-3.12863076631413,
-2.95830433805699,-2.79525046268999,-2.63930549851454,-2.48756465643266,
-2.30737197039185,-2.12968316227983,-1.95260099959419,-1.86352213387736,
-1.70295441302047,-1.55476562448681,-1.39890926825175,-1.22301319224729,
-1.1336969300927,-0.981472937761808,-0.835350461991401,-0.756826061006568,
-0.597584350396601,-0.38942460359425,-0.19920936171246,-0.100488991555656,
-9.10624732692347E-6),.UNSPECIFIED.);
#30551=B_SPLINE_CURVE_WITH_KNOTS('',3,(#215879,#215880,#215881,#215882,
#215883,#215884,#215885,#215886,#215887,#215888,#215889,#215890,#215891,
#215892,#215893,#215894,#215895,#215896,#215897,#215898,#215899,#215900,
#215901,#215902,#215903,#215904,#215905,#215906,#215907,#215908,#215909,
#215910,#215911,#215912,#215913,#215914,#215915,#215916,#215917,#215918,
#215919,#215920,#215921,#215922,#215923,#215924,#215925,#215926,#215927,
#215928,#215929,#215930,#215931,#215932,#215933,#215934,#215935,#215936,
#215937,#215938,#215939,#215940,#215941,#215942,#215943,#215944,#215945,
#215946,#215947,#215948),.UNSPECIFIED.,.F.,.F.,(4,2,2,2,2,2,2,2,2,2,2,2,
2,2,2,2,2,2,2,2,2,2,2,2,2,2,2,2,2,2,2,2,2,2,4),(-11.4419881045767,-11.2813757427722,
-10.9230195600775,-10.5627315202554,-10.3040525988962,-10.0984733872441,
-10.0109954258154,-9.83436174340115,-9.74575772244497,-9.60239614232087,
-9.52573747390332,-9.35709163921518,-9.23242885839426,-9.0787523283877,
-8.8991056633472,-8.81056299647559,-8.65235325948151,-8.50488912061725,
-8.34098326812671,-8.16271885955965,-8.07392192693336,-7.90764130003375,
-7.72001379955113,-7.56506656821126,-7.42215076339577,-7.24369481826094,
-7.06777708120355,-6.97852418519129,-6.82191574427426,-6.67154336340269,
-6.52324657455666,-6.34744501943803,-6.16753233716479,-5.8113316468472,
-5.72061718523155),.UNSPECIFIED.);
#30552=B_SPLINE_CURVE_WITH_KNOTS('',3,(#215949,#215950,#215951,#215952,
#215953,#215954,#215955,#215956,#215957,#215958,#215959,#215960,#215961,
#215962,#215963,#215964,#215965,#215966,#215967,#215968,#215969,#215970,
#215971,#215972,#215973,#215974,#215975,#215976,#215977,#215978,#215979,
#215980,#215981,#215982,#215983,#215984,#215985,#215986,#215987,#215988,
#215989,#215990,#215991,#215992,#215993,#215994,#215995,#215996,#215997,
#215998,#215999,#216000,#216001,#216002,#216003,#216004,#216005,#216006,
#216007,#216008,#216009,#216010),.UNSPECIFIED.,.F.,.F.,(4,2,2,2,2,2,2,2,
2,2,2,2,2,2,2,2,2,2,2,2,2,2,2,2,2,2,2,2,2,2,4),(-14.3060169149355,-14.2153533605477,
-13.8592013666033,-13.6793010719143,-13.5035148376052,-13.3553481442817,
-13.2008977678138,-13.0461650598207,-12.9568903328304,-12.7809148780731,
-12.6240853619038,-12.4969981438777,-12.3275773000993,-12.1235583172129,
-11.954900463041,-11.7571435569065,-11.5890846229911,-11.4181410921951,
-11.2476093170342,-11.0735226012537,-10.7173257541303,-10.4374746893783,
-10.279085066303,-10.1905159431329,-10.0138961142132,-9.92641324896063,
-9.72320254008456,-9.46435634533218,-9.10415884290171,-8.74601715292997,
-8.58352616457983),.UNSPECIFIED.);
#30553=B_SPLINE_CURVE_WITH_KNOTS('',3,(#216015,#216016,#216017,#216018,
#216019,#216020,#216021,#216022,#216023,#216024,#216025,#216026,#216027,
#216028,#216029,#216030,#216031,#216032,#216033,#216034,#216035,#216036,
#216037,#216038,#216039,#216040,#216041,#216042,#216043,#216044,#216045,
#216046,#216047,#216048,#216049,#216050,#216051,#216052,#216053,#216054,
#216055,#216056,#216057,#216058,#216059,#216060,#216061,#216062,#216063,
#216064,#216065,#216066,#216067,#216068,#216069,#216070,#216071,#216072,
#216073,#216074,#216075,#216076,#216077,#216078,#216079,#216080,#216081,
#216082),.UNSPECIFIED.,.F.,.F.,(4,2,2,2,2,2,2,2,2,2,2,2,2,2,2,2,2,2,2,2,
2,2,2,2,2,2,2,2,2,2,2,2,2,4),(-17.1637028159425,-17.060980079838,-16.9731277708488,
-16.7039506772942,-16.6158780571909,-16.2579619756541,-15.902163184888,
-15.7222693652696,-15.5464068666462,-15.4013221879371,-15.2469926384159,
-15.0895045273709,-15.0002592668443,-14.8243372318778,-14.6499630540693,
-14.4989074383824,-14.4109524992573,-14.0991443530046,-13.9481908664376,
-13.7545715781592,-13.6668395980893,-13.3716646622225,-13.2255092730848,
-13.0815190750491,-12.9115779913326,-12.6477158018356,-12.5071502928206,
-12.2921387977884,-12.1128676892355,-11.9372023629355,-11.7950742363449,
-11.6250873609284,-11.455560653579,-11.4419881045767),.UNSPECIFIED.);
#30554=B_SPLINE_CURVE_WITH_KNOTS('',3,(#216083,#216084,#216085,#216086,
#216087,#216088,#216089,#216090,#216091,#216092,#216093,#216094,#216095,
#216096,#216097,#216098,#216099,#216100,#216101,#216102,#216103,#216104,
#216105,#216106,#216107,#216108,#216109,#216110,#216111,#216112,#216113,
#216114,#216115,#216116,#216117,#216118,#216119,#216120,#216121,#216122,
#216123,#216124,#216125,#216126,#216127,#216128,#216129,#216130,#216131,
#216132,#216133,#216134,#216135,#216136,#216137,#216138,#216139,#216140,
#216141,#216142,#216143,#216144,#216145,#216146,#216147,#216148),
 .UNSPECIFIED.,.F.,.F.,(4,2,2,2,2,2,2,2,2,2,2,2,2,2,2,2,2,2,2,2,2,2,2,2,
2,2,2,2,2,2,2,2,4),(-8.58352616457983,-8.57213493872926,-8.4043656780315,
-8.23701159034506,-8.09922963062936,-7.8790859158866,-7.74110042947993,
-7.56032808455996,-7.26345493070519,-6.90746919946779,-6.73291365888483,
-6.56197986053401,-6.39019403814515,-6.2205243571735,-5.9923600289844,-5.90464672861176,
-5.71406901099162,-5.56250424947646,-5.38258318234043,-5.20398838814573,
-5.02796851980871,-4.93869431385693,-4.78385613976576,-4.62994880217048,
-4.48093247543028,-4.30514646512333,-4.12522809790341,-3.76913166638306,
-3.41116858385401,-3.32315902178704,-3.17015858971904,-2.99032705055544,
-2.86193028654911),.UNSPECIFIED.);
#30555=B_SPLINE_CURVE_WITH_KNOTS('',3,(#216154,#216155,#216156,#216157),
 .UNSPECIFIED.,.F.,.F.,(4,4),(0.000166910408644729,0.000172246164355015),
 .UNSPECIFIED.);
#30556=B_SPLINE_CURVE_WITH_KNOTS('',3,(#216159,#216160,#216161,#216162,
#216163,#216164),.UNSPECIFIED.,.F.,.F.,(4,2,4),(0.00015886842573906,0.234718197189778,
0.469154050605007),.UNSPECIFIED.);
#30557=B_SPLINE_CURVE_WITH_KNOTS('',3,(#216171,#216172,#216173,#216174,
#216175,#216176,#216177,#216178,#216179,#216180,#216181,#216182,#216183,
#216184,#216185,#216186,#216187,#216188,#216189,#216190,#216191,#216192,
#216193,#216194,#216195,#216196,#216197,#216198,#216199,#216200,#216201,
#216202,#216203,#216204,#216205,#216206,#216207,#216208,#216209,#216210,
#216211,#216212,#216213,#216214,#216215,#216216,#216217,#216218,#216219,
#216220,#216221,#216222,#216223,#216224,#216225,#216226,#216227,#216228,
#216229,#216230,#216231,#216232,#216233,#216234,#216235,#216236,#216237,
#216238,#216239,#216240,#216241,#216242,#216243,#216244),.UNSPECIFIED.,
 .F.,.F.,(4,2,2,2,2,2,2,2,2,2,2,2,2,2,2,2,2,2,2,2,2,2,2,2,2,2,2,2,2,2,2,
2,2,2,2,2,4),(-6.99964291132138,-6.96394858937547,-6.73463545641311,-6.49990723450948,
-6.27551710468842,-6.16173884786356,-5.93194349327878,-5.69738288218128,
-5.47300205903081,-5.35908307540296,-5.12907111679914,-4.89457892018263,
-4.67026667804598,-4.55619766722167,-4.32637859683717,-4.09175009325455,
-3.86759000101173,-3.75343478832399,-3.52419127870063,-3.25368513389825,
-3.13973680388134,-2.95254528949578,-2.72385358337876,-2.4451494752902,
-2.33112321801767,-2.0093121095651,-1.89438301602845,-1.73461634653569,
-1.50777243640498,-1.2869037055871,-1.06277033526056,-0.948922951171791,
-0.720534931469837,-0.485452231856019,-0.245885103670598,-0.123137748004486,
-0.00053524047117373),.UNSPECIFIED.);
#30558=B_SPLINE_CURVE_WITH_KNOTS('',3,(#216247,#216248,#216249,#216250,
#216251,#216252,#216253,#216254,#216255,#216256,#216257,#216258,#216259,
#216260,#216261,#216262,#216263,#216264,#216265,#216266,#216267,#216268,
#216269,#216270,#216271,#216272,#216273,#216274,#216275,#216276,#216277,
#216278,#216279,#216280,#216281,#216282,#216283,#216284,#216285,#216286,
#216287,#216288,#216289,#216290,#216291,#216292,#216293,#216294,#216295,
#216296,#216297,#216298,#216299,#216300,#216301,#216302,#216303,#216304,
#216305,#216306,#216307,#216308,#216309,#216310,#216311,#216312,#216313,
#216314,#216315,#216316,#216317,#216318),.UNSPECIFIED.,.F.,.F.,(4,2,2,2,
2,2,2,2,2,2,2,2,2,2,2,2,2,2,2,2,2,2,2,2,2,2,2,2,2,2,2,2,2,2,2,4),(-24.6757663477501,
-24.5533436654801,-24.4307711038346,-24.1915697619018,-23.9564679661864,
-23.7281366468575,-23.6142452247218,-23.3901168444522,-23.1548585281943,
-23.040619601695,-22.7722458466604,-22.6576238849321,-22.4301674660062,
-22.206076808646,-21.9625811024712,-21.7349429828328,-21.5767302857709,
-21.4620624951134,-21.2330970713377,-21.0089981637414,-20.7547023533752,
-20.5255173717378,-20.3722665776375,-20.2577140022871,-19.937803146283,
-19.7067859523919,-19.4772611387739,-19.1295462031688,-19.015361295707,
-18.7919457097124,-18.5670290601582,-18.332361974679,-18.2181203927842,
-17.9941659427034,-17.76958038057,-17.675937012053),.UNSPECIFIED.);
#30559=B_SPLINE_CURVE_WITH_KNOTS('',3,(#216323,#216324,#216325,#216326,
#216327,#216328,#216329,#216330,#216331,#216332,#216333,#216334,#216335,
#216336,#216337,#216338,#216339,#216340,#216341,#216342,#216343,#216344,
#216345,#216346,#216347,#216348,#216349,#216350,#216351,#216352,#216353,
#216354,#216355,#216356,#216357,#216358,#216359,#216360,#216361,#216362,
#216363,#216364,#216365,#216366,#216367,#216368,#216369,#216370,#216371,
#216372,#216373,#216374,#216375,#216376,#216377,#216378,#216379,#216380,
#216381,#216382,#216383,#216384,#216385,#216386,#216387,#216388,#216389,
#216390,#216391,#216392,#216393,#216394,#216395,#216396,#216397,#216398),
 .UNSPECIFIED.,.F.,.F.,(4,2,2,2,2,2,2,2,2,2,2,2,2,2,2,2,2,2,2,2,2,2,2,2,
2,2,2,2,2,2,2,2,2,2,2,2,2,4),(-14.4469920765838,-14.3339145542341,-14.1050748344662,
-13.9912231520843,-13.7669491019276,-13.5318755495119,-13.3035366786338,
-13.1121862203767,-12.9981460748547,-12.7756563829289,-12.5512394960465,
-12.3377263279076,-12.1170350634801,-11.8925161013489,-11.7787201437416,
-11.5485381666371,-11.2577338092456,-11.1435996416612,-10.8691626700202,
-10.7551801220181,-10.4083716979756,-10.1772692913796,-9.94810338992655,
-9.63183711218707,-9.51709302956755,-9.36871627394153,-9.14044456903546,
-8.9051890107586,-8.68108149544486,-8.56723085598633,-8.33887699025705,
-8.10375453299894,-7.87949303584005,-7.76573182405683,-7.53696692993187,
-7.30202815163844,-7.07767053099068,-6.99964291132138),.UNSPECIFIED.);
#30560=B_SPLINE_CURVE_WITH_KNOTS('',3,(#216399,#216400,#216401,#216402,
#216403,#216404,#216405,#216406,#216407,#216408,#216409,#216410,#216411,
#216412,#216413,#216414,#216415,#216416,#216417,#216418,#216419,#216420,
#216421,#216422,#216423,#216424,#216425,#216426,#216427,#216428,#216429,
#216430,#216431,#216432,#216433,#216434,#216435,#216436,#216437,#216438,
#216439,#216440,#216441,#216442,#216443,#216444,#216445,#216446,#216447,
#216448,#216449,#216450,#216451,#216452,#216453,#216454,#216455,#216456,
#216457,#216458,#216459,#216460,#216461,#216462,#216463,#216464,#216465,
#216466,#216467,#216468,#216469,#216470,#216471,#216472,#216473,#216474,
#216475,#216476),.UNSPECIFIED.,.F.,.F.,(4,2,2,2,2,2,2,2,2,2,2,2,2,2,2,2,
2,2,2,2,2,2,2,2,2,2,2,2,2,2,2,2,2,2,2,2,2,2,4),(-17.675937012053,-17.541667988348,
-17.3127948338258,-17.1989373991103,-16.9746455461691,-16.7395623888719,
-16.5111942932525,-16.3972697177496,-16.173096276875,-15.937840867139,-15.7097470667384,
-15.5957282273868,-15.3717063968006,-15.1363769908546,-14.9081664213362,
-14.7575876744846,-14.6428942325424,-14.4145872524929,-14.1904560789865,
-13.9434569157579,-13.8291588794412,-13.5264564835631,-13.4123746202815,
-13.1286563608922,-12.8985952015119,-12.784689567824,-12.5602259551404,
-12.3386056468598,-12.1227904334969,-11.8984111410574,-11.6756230896314,
-11.5615489911593,-11.3771973098817,-11.1484317978468,-10.9134094215749,
-10.68899971096,-10.4649257225573,-10.35065873192,-10.22845558376),
 .UNSPECIFIED.);
#30561=B_SPLINE_CURVE_WITH_KNOTS('',3,(#216481,#216482,#216483,#216484,
#216485,#216486,#216487,#216488,#216489,#216490,#216491,#216492,#216493,
#216494,#216495,#216496,#216497,#216498,#216499,#216500,#216501,#216502,
#216503,#216504,#216505,#216506,#216507,#216508,#216509,#216510,#216511,
#216512,#216513,#216514,#216515,#216516,#216517,#216518,#216519,#216520,
#216521,#216522,#216523,#216524,#216525,#216526,#216527,#216528,#216529,
#216530,#216531,#216532,#216533,#216534,#216535,#216536,#216537,#216538,
#216539,#216540,#216541,#216542,#216543,#216544,#216545,#216546,#216547,
#216548,#216549,#216550,#216551,#216552,#216553,#216554,#216555,#216556),
 .UNSPECIFIED.,.F.,.F.,(4,2,2,2,2,2,2,2,2,2,2,2,2,2,2,2,2,2,2,2,2,2,2,2,
2,2,2,2,2,2,2,2,2,2,2,2,2,4),(-21.8943047423385,-21.7758651347812,-21.5410515033964,
-21.4268285997185,-21.2030184270806,-20.9786575429375,-20.7625105893418,
-20.6478936288047,-20.3698911794026,-20.2550588086357,-19.9389522360808,
-19.8248572046001,-19.5625496742136,-19.3359762790518,-19.1730889945457,
-19.0582271151876,-18.829574401143,-18.6052712102383,-18.3485145033467,
-18.1199766319641,-18.0056172240497,-17.7816376834012,-17.5794451870502,
-17.3443875772851,-17.1711327726157,-17.0564223246057,-16.7285022822342,
-16.4973841529025,-16.2679629029584,-15.9218777080356,-15.8076985043827,
-15.5842721602659,-15.3593844814189,-15.1247284981361,-15.0104927267103,
-14.7865329091102,-14.5619722283021,-14.4469920765838),.UNSPECIFIED.);
#30562=B_SPLINE_CURVE_WITH_KNOTS('',3,(#216557,#216558,#216559,#216560,
#216561,#216562,#216563,#216564,#216565,#216566,#216567,#216568,#216569,
#216570,#216571,#216572,#216573,#216574,#216575,#216576,#216577,#216578,
#216579,#216580,#216581,#216582,#216583,#216584,#216585,#216586,#216587,
#216588,#216589,#216590,#216591,#216592,#216593,#216594,#216595,#216596,
#216597,#216598,#216599,#216600,#216601,#216602,#216603,#216604,#216605,
#216606,#216607,#216608,#216609,#216610,#216611,#216612,#216613,#216614,
#216615,#216616,#216617,#216618,#216619,#216620,#216621,#216622,#216623,
#216624,#216625,#216626,#216627,#216628,#216629,#216630,#216631,#216632,
#216633,#216634),.UNSPECIFIED.,.F.,.F.,(4,2,2,2,2,2,2,2,2,2,2,2,2,2,2,2,
2,2,2,2,2,2,2,2,2,2,2,2,2,2,2,2,2,2,2,2,2,2,4),(-10.22845558376,-10.1158401265768,
-9.89115177753051,-9.66761368388471,-9.55338621355086,-9.23692071620921,
-9.122370932652,-8.88771372650107,-8.66369006558576,-8.54886806983543,-8.3206913669332,
-8.05897886871758,-7.94483082538692,-7.62945980835995,-7.51499320151402,
-7.23290372901667,-7.11853656580412,-6.855130090617,-6.74109476064902,-6.41878779605464,
-6.30405435983148,-6.13915860379677,-5.90440188687171,-5.74427454092565,
-5.51714392881869,-5.26655270450146,-5.04193707803073,-4.81349746352477,
-4.6984382894124,-4.53524967574988,-4.30883411100736,-4.0454369895731,-3.93119365547195,
-3.69615849635357,-3.47178830981662,-3.24790775411328,-3.13367035284959,
-2.89883668306189,-2.78075214770189),.UNSPECIFIED.);
#30563=B_SPLINE_CURVE_WITH_KNOTS('',3,(#216640,#216641,#216642,#216643),
 .UNSPECIFIED.,.F.,.F.,(4,4),(-2.98098074791244E-6,-9.99999995798516E-7),
 .UNSPECIFIED.);
#30564=B_SPLINE_CURVE_WITH_KNOTS('',3,(#216645,#216646,#216647,#216648,
#216649,#216650,#216651,#216652,#216653,#216654,#216655,#216656,#216657,
#216658,#216659,#216660,#216661,#216662,#216663,#216664,#216665,#216666,
#216667,#216668),.UNSPECIFIED.,.F.,.F.,(4,2,2,2,2,2,2,2,2,2,2,4),(-1.88511749361157,
-1.67932546304624,-1.47452695338293,-1.33807794175079,-1.10356670932426,
-0.989276198914495,-0.873916728340471,-0.661501516222309,-0.498025259869575,
-0.252000037418745,-0.126229715199769,-0.000254800321387329),
 .UNSPECIFIED.);
#30565=B_SPLINE_CURVE_WITH_KNOTS('',3,(#216671,#216672,#216673,#216674,
#216675,#216676,#216677,#216678,#216679,#216680,#216681,#216682,#216683,
#216684,#216685,#216686,#216687,#216688,#216689,#216690,#216691,#216692),
 .UNSPECIFIED.,.F.,.F.,(4,2,2,2,2,2,2,2,2,2,4),(5.98718350673662E-5,0.203932709927782,
0.406516261468655,0.541488095383629,0.718522052217718,0.942619519328621,
1.17051888563091,1.39440958810066,1.63674335451055,1.76079483716829,1.88502497314799),
 .UNSPECIFIED.);
#30566=B_SPLINE_CURVE_WITH_KNOTS('',3,(#216695,#216696,#216697,#216698,
#216699,#216700,#216701,#216702,#216703,#216704,#216705,#216706,#216707,
#216708,#216709,#216710,#216711,#216712,#216713,#216714,#216715,#216716,
#216717,#216718,#216719,#216720,#216721,#216722,#216723,#216724,#216725,
#216726,#216727,#216728,#216729,#216730,#216731,#216732,#216733,#216734,
#216735,#216736,#216737,#216738,#216739,#216740,#216741,#216742,#216743,
#216744,#216745,#216746,#216747,#216748,#216749,#216750,#216751,#216752,
#216753,#216754,#216755,#216756,#216757,#216758,#216759,#216760,#216761,
#216762,#216763,#216764,#216765,#216766,#216767,#216768,#216769,#216770,
#216771,#216772),.UNSPECIFIED.,.F.,.F.,(4,2,2,2,2,2,2,2,2,2,2,2,2,2,2,2,
2,2,2,2,2,2,2,2,2,2,2,2,2,2,2,2,2,2,2,2,2,2,4),(-22.7887754871925,-22.5737853607563,
-22.3645912829662,-22.2250703698579,-21.9520105528446,-21.7234422036205,
-21.5344458228471,-21.4205033205513,-21.1505966646988,-20.9213671507031,
-20.8072028928257,-20.5830474551358,-20.3484175287191,-20.1186112362477,
-20.0045315383634,-19.7802237481903,-19.5457292550042,-19.315729471641,
-19.2017990774839,-18.9774229981112,-18.7428603593495,-18.5130776936426,
-18.3992883308069,-18.1749036431537,-17.9401751152226,-17.7108762627284,
-17.5971442416489,-17.3727928848634,-17.1391574499357,-16.9105229740035,
-16.79667802978,-16.5724458853296,-16.3394723212058,-16.111442940754,-15.9973964286305,
-15.7733306583291,-15.5380042916193,-15.4237362863445,-15.342147766727),
 .UNSPECIFIED.);
#30567=B_SPLINE_CURVE_WITH_KNOTS('',3,(#216775,#216776,#216777,#216778,
#216779,#216780,#216781,#216782,#216783,#216784,#216785,#216786,#216787,
#216788,#216789,#216790,#216791,#216792,#216793,#216794,#216795,#216796,
#216797,#216798,#216799,#216800,#216801,#216802,#216803,#216804,#216805,
#216806,#216807,#216808,#216809,#216810,#216811,#216812,#216813,#216814,
#216815,#216816,#216817,#216818,#216819,#216820,#216821,#216822,#216823,
#216824,#216825,#216826,#216827,#216828,#216829,#216830,#216831,#216832,
#216833,#216834,#216835,#216836,#216837,#216838,#216839,#216840,#216841,
#216842,#216843,#216844,#216845,#216846,#216847,#216848,#216849,#216850,
#216851,#216852),.UNSPECIFIED.,.F.,.F.,(4,2,2,2,2,2,2,2,2,2,2,2,2,2,2,2,
2,2,2,2,2,2,2,2,2,2,2,2,2,2,2,2,2,2,2,2,2,2,4),(-7.44718343892512,-7.36240446244989,
-7.24805819005065,-7.02308065474895,-6.79889962536361,-6.68521835702744,
-6.456593568243,-6.22151211684303,-5.9971659350046,-5.7732432646884,-5.65900294954311,
-5.42412826474149,-5.19948668701251,-4.97616348979199,-4.86194591875158,
-4.62722551562504,-4.40217320669064,-4.16739074652333,-4.0531419222947,
-3.81856601393786,-3.59383807002767,-3.36961197351575,-3.25544477485063,
-2.92967683372141,-2.81502248789315,-2.65144118011975,-2.423646930303,-2.14811559177375,
-2.03388722384771,-1.78699119824193,-1.56303399023159,-1.33478382184713,
-1.22030231366281,-0.942135255595247,-0.827820820338569,-0.584107166585578,
-0.439444762624892,-0.221298301331629,-2.98098074791244E-6),
 .UNSPECIFIED.);
#30568=B_SPLINE_CURVE_WITH_KNOTS('',3,(#216857,#216858,#216859,#216860,
#216861,#216862,#216863,#216864,#216865,#216866,#216867,#216868,#216869,
#216870,#216871,#216872,#216873,#216874,#216875,#216876,#216877,#216878,
#216879,#216880,#216881,#216882,#216883,#216884,#216885,#216886,#216887,
#216888,#216889,#216890,#216891,#216892,#216893,#216894,#216895,#216896,
#216897,#216898,#216899,#216900,#216901,#216902,#216903,#216904,#216905,
#216906,#216907,#216908,#216909,#216910,#216911,#216912,#216913,#216914,
#216915,#216916,#216917,#216918,#216919,#216920,#216921,#216922,#216923,
#216924,#216925,#216926,#216927,#216928,#216929,#216930,#216931,#216932,
#216933,#216934),.UNSPECIFIED.,.F.,.F.,(4,2,2,2,2,2,2,2,2,2,2,2,2,2,2,2,
2,2,2,2,2,2,2,2,2,2,2,2,2,2,2,2,2,2,2,2,2,2,4),(-14.8947554416205,-14.8555328238902,
-14.6255932266936,-14.5115483148371,-14.2871917339874,-14.0526532288194,
-13.8227502409632,-13.7088584582275,-13.4844700238339,-13.2568809816448,
-13.0280884043627,-12.9138754281338,-12.689658624793,-12.4904413403656,
-12.2654119085154,-12.0529319801525,-11.8248485904798,-11.6246180764855,
-11.3947343862561,-11.280540944454,-11.1009100249439,-10.8701321621013,
-10.6356115829466,-10.4108478312659,-10.186578073999,-10.0724663873352,
-9.73649474395671,-9.62156564200684,-9.41972195006705,-9.19568899880307,
-9.08133069845105,-8.85261827817306,-8.59523573549692,-8.37092206998091,
-8.14210122680411,-8.02723354700109,-7.86215740024421,-7.63576125229907,
-7.44718343892512),.UNSPECIFIED.);
#30569=B_SPLINE_CURVE_WITH_KNOTS('',3,(#216935,#216936,#216937,#216938,
#216939,#216940,#216941,#216942,#216943,#216944,#216945,#216946,#216947,
#216948,#216949,#216950,#216951,#216952,#216953,#216954,#216955,#216956,
#216957,#216958,#216959,#216960,#216961,#216962,#216963,#216964,#216965,
#216966,#216967,#216968,#216969,#216970,#216971,#216972,#216973,#216974,
#216975,#216976,#216977,#216978,#216979,#216980,#216981,#216982,#216983,
#216984,#216985,#216986,#216987,#216988,#216989,#216990,#216991,#216992,
#216993,#216994,#216995,#216996,#216997,#216998,#216999,#217000,#217001,
#217002,#217003,#217004,#217005,#217006,#217007,#217008,#217009,#217010,
#217011,#217012),.UNSPECIFIED.,.F.,.F.,(4,2,2,2,2,2,2,2,2,2,2,2,2,2,2,2,
2,2,2,2,2,2,2,2,2,2,2,2,2,2,2,2,2,2,2,2,2,2,4),(-15.342147766727,-15.1529720065065,
-15.0383703444976,-14.810809948066,-14.586751207086,-14.3429750891665,-14.1152058277465,
-13.9570672325687,-13.8424259697976,-13.6133621923892,-13.3892883641721,
-13.1714179393148,-13.0564020234404,-12.716404767469,-12.6023018240209,
-12.3781455868867,-12.1533575609804,-11.9188469906034,-11.6880294779991,
-11.509248903507,-11.3950609040316,-11.165177855366,-10.963986090416,-10.7359806575178,
-10.5257207831069,-10.3006120053153,-10.0657543218304,-9.9515117616543,
-9.71678726270671,-9.49192700742318,-9.26870398584334,-9.15450428638233,
-8.80897988487314,-8.69389321850089,-8.4777887626932,-8.25370904546708,
-8.02408547888485,-7.90947386498692,-7.89471088538268),.UNSPECIFIED.);
#30570=B_SPLINE_CURVE_WITH_KNOTS('',3,(#217017,#217018,#217019,#217020,
#217021,#217022,#217023,#217024,#217025,#217026,#217027,#217028,#217029,
#217030,#217031,#217032,#217033,#217034,#217035,#217036,#217037,#217038,
#217039,#217040,#217041,#217042,#217043,#217044,#217045,#217046,#217047,
#217048,#217049,#217050,#217051,#217052,#217053,#217054,#217055,#217056,
#217057,#217058,#217059,#217060,#217061,#217062,#217063,#217064,#217065,
#217066,#217067,#217068,#217069,#217070,#217071,#217072,#217073,#217074,
#217075,#217076,#217077,#217078,#217079,#217080,#217081,#217082,#217083,
#217084,#217085,#217086,#217087,#217088,#217089,#217090,#217091,#217092,
#217093,#217094),.UNSPECIFIED.,.F.,.F.,(4,2,2,2,2,2,2,2,2,2,2,2,2,2,2,2,
2,2,2,2,2,2,2,2,2,2,2,2,2,2,2,2,2,2,2,2,2,2,4),(-22.3420595105916,-22.3087706117589,
-22.1501209153067,-21.9431458113864,-21.7193635049408,-21.4944800880326,
-21.2599207185237,-21.1456978247876,-20.9213787890152,-20.6967842790541,
-20.4620796048301,-20.3477868290561,-20.1129279053258,-19.8881009482717,
-19.6532740453404,-19.5390667997237,-19.315609140037,-19.0911533599053,
-18.8561460335345,-18.741939321533,-18.5067222121917,-18.2821685233984,
-18.0715067743307,-17.9570526515047,-17.6559632223792,-17.5418483339653,
-17.2763985394528,-17.1618752207304,-16.9343481155266,-16.7103507009649,
-16.4662542480478,-16.2380547179748,-16.0388216827039,-15.924846808128,
-15.6580555001392,-15.4285045183689,-15.314337636522,-15.090086051584,-14.8947554416205),
 .UNSPECIFIED.);
#30571=B_SPLINE_CURVE_WITH_KNOTS('',3,(#217095,#217096,#217097,#217098,
#217099,#217100,#217101,#217102,#217103,#217104,#217105,#217106,#217107,
#217108,#217109,#217110,#217111,#217112,#217113,#217114,#217115,#217116,
#217117,#217118,#217119,#217120,#217121,#217122,#217123,#217124,#217125,
#217126,#217127,#217128,#217129,#217130,#217131,#217132,#217133,#217134,
#217135,#217136,#217137,#217138,#217139,#217140,#217141,#217142,#217143,
#217144,#217145,#217146,#217147,#217148,#217149,#217150,#217151,#217152,
#217153,#217154,#217155,#217156,#217157,#217158,#217159,#217160,#217161,
#217162,#217163,#217164,#217165,#217166,#217167,#217168,#217169,#217170,
#217171,#217172),.UNSPECIFIED.,.F.,.F.,(4,2,2,2,2,2,2,2,2,2,2,2,2,2,2,2,
2,2,2,2,2,2,2,2,2,2,2,2,2,2,2,2,2,2,2,2,2,2,4),(-7.89471088538268,-7.7513446470039,
-7.52274813975883,-7.27356060895527,-7.04945125083501,-6.82000660796923,
-6.70532977234191,-6.54058473742381,-6.3057493848618,-6.14534762068587,
-5.91799925641447,-5.66491089523042,-5.55102496010023,-5.3375198753743,
-5.11108617476756,-4.84273060467716,-4.72849634427378,-4.49323939229272,
-4.2691188750551,-4.15523017770918,-3.92691048583833,-3.69180245193583,
-3.46753946147414,-3.35373345582603,-3.12496264585747,-2.89005372862249,
-2.66571673663732,-2.55193417606568,-2.32261364211153,-2.08792618496844,
-1.8635724908039,-1.74971746957993,-1.51994827839982,-1.28540978867085,
-1.06107669190666,-0.947078264469952,-0.717152631942884,-0.482651609103955,
-0.448047571937242),.UNSPECIFIED.);
#30572=B_SPLINE_CURVE_WITH_KNOTS('',3,(#217180,#217181,#217182,#217183),
 .UNSPECIFIED.,.F.,.F.,(4,4),(0.,0.000776497203231734),.UNSPECIFIED.);
#30573=B_SPLINE_CURVE_WITH_KNOTS('',3,(#217185,#217186,#217187,#217188,
#217189,#217190,#217191,#217192,#217193,#217194,#217195,#217196,#217197,
#217198,#217199,#217200,#217201,#217202,#217203,#217204,#217205,#217206,
#217207,#217208,#217209,#217210,#217211,#217212,#217213,#217214),
 .UNSPECIFIED.,.F.,.F.,(4,2,2,2,2,2,2,2,2,2,2,2,2,2,4),(-2.58819132413352,
-2.3627357246396,-2.13741551586203,-1.98563553180878,-1.79408322231036,
-1.60046605723288,-1.40804760753431,-1.31130466449952,-1.11849752052538,
-0.921488213499259,-0.727078362402504,-0.545763875761456,-0.273849840655846,
-0.136429802224194,-1.19577251124937E-5),.UNSPECIFIED.);
#30574=B_SPLINE_CURVE_WITH_KNOTS('',3,(#217216,#217217,#217218,#217219,
#217220,#217221,#217222,#217223,#217224,#217225,#217226,#217227,#217228,
#217229,#217230,#217231,#217232,#217233,#217234,#217235,#217236,#217237,
#217238,#217239,#217240,#217241,#217242,#217243,#217244,#217245,#217246,
#217247,#217248,#217249),.UNSPECIFIED.,.F.,.F.,(4,2,2,2,2,2,2,2,2,2,2,2,
2,2,2,2,4),(-2.54573725986498,-2.37476608201507,-2.20211346081785,-2.08770172421587,
-1.93349297075605,-1.75019087472256,-1.56693226938244,-1.47443768915228,
-1.29039242591535,-1.19762811175894,-1.01304591077278,-0.825229741583214,
-0.638712708813142,-0.47916634693947,-0.24037936089956,-0.119773973838393,
-2.99430650417543E-6),.UNSPECIFIED.);
#30575=B_SPLINE_CURVE_WITH_KNOTS('',3,(#217252,#217253,#217254,#217255,
#217256,#217257,#217258,#217259,#217260,#217261,#217262,#217263,#217264,
#217265,#217266,#217267,#217268,#217269,#217270,#217271,#217272,#217273,
#217274,#217275,#217276,#217277,#217278,#217279,#217280,#217281,#217282,
#217283,#217284,#217285,#217286,#217287,#217288),.UNSPECIFIED.,.F.,.F.,
(4,3,3,3,3,3,3,3,3,3,3,3,4),(0.,0.0940528831804161,0.188071722346358,0.282046558286538,
0.375986938964542,0.469884151166454,0.5,0.593548460116691,0.686978341973026,
0.780242306988025,0.873402721160576,0.966421835499172,0.999999946312436),
 .UNSPECIFIED.);
#30576=B_SPLINE_CURVE_WITH_KNOTS('',3,(#217291,#217292,#217293,#217294,
#217295,#217296,#217297,#217298,#217299,#217300,#217301,#217302),
 .UNSPECIFIED.,.F.,.F.,(4,2,2,2,2,4),(1.41602269427444E-5,0.103268302452876,
0.209393167485349,0.424646829433195,0.5311273537776,0.948508841723998),
 .UNSPECIFIED.);
#30577=B_SPLINE_CURVE_WITH_KNOTS('',3,(#217311,#217312,#217313,#217314,
#217315,#217316,#217317,#217318),.UNSPECIFIED.,.F.,.F.,(4,2,2,4),(-0.448047571937242,
-0.24397532728341,-0.122603630859418,-0.000536776025982476),
 .UNSPECIFIED.);
#30578=B_SPLINE_CURVE_WITH_KNOTS('',3,(#217319,#217320,#217321,#217322,
#217323,#217324,#217325,#217326),.UNSPECIFIED.,.F.,.F.,(4,2,2,4),(-22.7895799823983,
-22.6678389417462,-22.5467817476268,-22.3420595105916),.UNSPECIFIED.);
#30579=B_SPLINE_CURVE_WITH_KNOTS('',3,(#217329,#217330,#217331,#217332,
#217333,#217334,#217335,#217336,#217337,#217338,#217339,#217340,#217341,
#217342,#217343,#217344,#217345,#217346,#217347,#217348,#217349,#217350,
#217351,#217352,#217353,#217354,#217355,#217356,#217357,#217358,#217359,
#217360),.UNSPECIFIED.,.F.,.F.,(4,2,2,2,2,2,2,2,2,2,2,2,2,2,2,4),(-2.78075214770189,
-2.67416520655263,-2.45088006356431,-2.33666972312661,-2.10198688626357,
-1.87689522479149,-1.64214565828053,-1.52791483266349,-1.29337178707801,
-1.06862921741881,-0.844459861678536,-0.739641881971006,-0.55627135957414,
-0.278570352687516,-0.140184550502981,-0.000333910314163745),
 .UNSPECIFIED.);
#30580=B_SPLINE_CURVE_WITH_KNOTS('',3,(#217363,#217364,#217365,#217366,
#217367,#217368,#217369,#217370,#217371,#217372,#217373,#217374,#217375,
#217376,#217377,#217378,#217379,#217380,#217381,#217382,#217383,#217384,
#217385,#217386,#217387,#217388,#217389,#217390,#217391,#217392,#217393,
#217394),.UNSPECIFIED.,.F.,.F.,(4,2,2,2,2,2,2,2,2,2,2,2,2,2,2,4),(-24.6745311376285,
-24.5346323571423,-24.3961991428265,-24.1183826232944,-23.9348941546191,
-23.8300338079026,-23.6059502628919,-23.3811973449391,-23.146667341407,
-23.0324471264885,-22.7977120868547,-22.5726065945869,-22.3379394752642,
-22.22374090337,-22.0005377731445,-21.8943047423385),.UNSPECIFIED.);
#30581=B_SPLINE_CURVE_WITH_KNOTS('',3,(#217398,#217399,#217400,#217401,
#217402,#217403,#217404,#217405,#217406,#217407,#217408),.UNSPECIFIED.,
 .F.,.F.,(4,2,3,2,4),(-0.707920522022895,-0.389439958817396,0.,0.389439958817396,
0.707920522023277),.UNSPECIFIED.);
#30582=B_SPLINE_CURVE_WITH_KNOTS('',3,(#217412,#217413,#217414,#217415,
#217416,#217417,#217418,#217419,#217420,#217421,#217422),.UNSPECIFIED.,
 .F.,.F.,(4,2,3,2,4),(-0.704072833963995,-0.391088299603276,0.,0.390169294707907,
0.573011129927049),.UNSPECIFIED.);
#30583=B_SPLINE_CURVE_WITH_KNOTS('',3,(#217424,#217425,#217426,#217427),
 .UNSPECIFIED.,.F.,.F.,(4,4),(0.573011129927049,0.704038599815),
 .UNSPECIFIED.);
#30584=B_SPLINE_CURVE_WITH_KNOTS('',3,(#217433,#217434,#217435,#217436,
#217437,#217438,#217439,#217440,#217441,#217442,#217443,#217444,#217445,
#217446,#217447,#217448,#217449,#217450,#217451,#217452,#217453,#217454,
#217455,#217456,#217457,#217458,#217459,#217460,#217461,#217462,#217463,
#217464,#217465,#217466,#217467,#217468),.UNSPECIFIED.,.F.,.F.,(4,2,2,2,
2,2,2,2,2,2,2,2,2,2,2,2,2,4),(-2.69278601163302,-2.48949828256942,-2.2822953333751,
-2.14458879630419,-1.96754811547026,-1.79103983134041,-1.61387421528028,
-1.4368871200193,-1.34835665174934,-1.25978242304794,-1.08286142569904,
-0.905901114537669,-0.728942624524571,-0.640388431951228,-0.480377748963507,
-0.24014543853639,-0.120091889663099,-0.000154281167704561),
 .UNSPECIFIED.);
#30585=B_SPLINE_CURVE_WITH_KNOTS('',3,(#217469,#217470,#217471,#217472,
#217473,#217474,#217475,#217476,#217477,#217478,#217479,#217480,#217481,
#217482,#217483,#217484,#217485,#217486,#217487,#217488,#217489,#217490,
#217491,#217492,#217493,#217494,#217495,#217496,#217497,#217498,#217499,
#217500),.UNSPECIFIED.,.F.,.F.,(4,2,2,2,2,2,2,2,2,2,2,2,2,2,2,4),(-2.46530051632309,
-2.26819680103626,-2.07119546180983,-1.93999090652251,-1.76308472874,-1.58642929791097,
-1.40948483540438,-1.23270430940226,-1.05614800855202,-0.879169642199461,
-0.702326874356245,-0.525413854334426,-0.394197725784808,-0.197144745652885,
-0.0986007555144971,-0.000263540357241407),.UNSPECIFIED.);
#30586=B_SPLINE_CURVE_WITH_KNOTS('',3,(#217502,#217503,#217504,#217505,
#217506,#217507,#217508,#217509,#217510,#217511,#217512,#217513,#217514,
#217515,#217516,#217517,#217518,#217519,#217520,#217521,#217522,#217523,
#217524,#217525),.UNSPECIFIED.,.F.,.F.,(4,2,2,2,2,2,2,2,2,2,2,4),(0.000318649964459465,
0.216450635165624,0.43221115121817,0.575746846605652,0.931054759121386,
1.28597766699898,1.46245055330704,1.63929983860731,1.81580252156612,1.97755622729653,
2.22237862591288,2.46755233424745),.UNSPECIFIED.);
#30587=B_SPLINE_CURVE_WITH_KNOTS('',3,(#217526,#217527,#217528,#217529,
#217530,#217531,#217532,#217533,#217534,#217535,#217536,#217537,#217538,
#217539,#217540,#217541,#217542,#217543,#217544,#217545,#217546,#217547,
#217548,#217549,#217550,#217551,#217552,#217553,#217554,#217555,#217556,
#217557,#217558,#217559),.UNSPECIFIED.,.F.,.F.,(4,2,2,2,2,2,2,2,2,2,2,2,
2,2,2,2,4),(0.000172246164355015,0.137421045642985,0.274393819056073,0.548014470689402,
0.723404022606042,0.900115325731667,1.07657549560485,1.25300012233027,1.43023293239451,
1.78627993866689,1.87475807665471,2.05193119898048,2.14050616753244,2.31698447474687,
2.58688835542286,2.72343276379947,2.8600131789018),.UNSPECIFIED.);
#30588=B_SPLINE_CURVE_WITH_KNOTS('',3,(#217562,#217563,#217564,#217565,
#217566,#217567,#217568,#217569,#217570,#217571,#217572,#217573,#217574,
#217575,#217576,#217577,#217578,#217579,#217580,#217581,#217582,#217583,
#217584,#217585,#217586,#217587,#217588,#217589,#217590,#217591),
 .UNSPECIFIED.,.F.,.F.,(4,2,2,2,2,2,2,2,2,2,2,2,2,2,4),(-2.86193028654911,
-2.80997689806081,-2.53859155289255,-2.45079675084397,-2.1519918870356,
-1.79660795427829,-1.62313020729879,-1.45278636887481,-1.28271379788856,
-1.12400310249263,-0.967139554823996,-0.815414409998087,-0.636542489421722,
-0.323024007865446,-9.999999992516E-7),.UNSPECIFIED.);
#30589=B_SPLINE_CURVE_WITH_KNOTS('',3,(#217592,#217593,#217594,#217595,
#217596,#217597,#217598,#217599,#217600,#217601,#217602,#217603,#217604,
#217605,#217606,#217607,#217608,#217609,#217610,#217611,#217612,#217613,
#217614,#217615),.UNSPECIFIED.,.F.,.F.,(4,2,2,2,2,2,2,2,2,2,2,4),(-2.07371028242565,
-1.89670800614931,-1.71936907413992,-1.6040015767827,-1.44968076011158,
-1.09401343727901,-0.738422468249123,-0.650645318605829,-0.498854971265117,
-0.251161099398345,-0.127294929695514,-0.000361776623968905),
 .UNSPECIFIED.);
#30590=B_SPLINE_CURVE_WITH_KNOTS('',3,(#217617,#217618,#217619,#217620,
#217621,#217622,#217623,#217624,#217625,#217626,#217627,#217628,#217629,
#217630,#217631,#217632,#217633,#217634,#217635,#217636,#217637,#217638,
#217639,#217640,#217641,#217642),.UNSPECIFIED.,.F.,.F.,(4,2,2,2,2,2,2,2,
2,2,2,2,4),(0.000219774119996971,0.128265976878325,0.255769893159544,0.493856419136537,
0.651486942309664,0.821726852996873,1.03589976718783,1.25551703969422,1.3939988560134,
1.57317372451587,1.82118610863373,1.94515901785584,2.07223113354457),
 .UNSPECIFIED.);
#30591=B_SPLINE_CURVE_WITH_KNOTS('',3,(#217643,#217644,#217645,#217646,
#217647,#217648,#217649,#217650,#217651,#217652,#217653,#217654,#217655,
#217656,#217657,#217658,#217659,#217660,#217661,#217662,#217663,#217664,
#217665,#217666,#217667,#217668,#217669,#217670,#217671,#217672),
 .UNSPECIFIED.,.F.,.F.,(4,2,2,2,2,2,2,2,2,2,2,2,2,2,4),(-20.0257156012565,
-19.7027546279237,-19.3893986009445,-19.210538838357,-19.0591308279729,
-18.9074787091117,-18.7457793362987,-18.5752767544231,-18.404751196263,
-18.2310130985394,-17.8756055227173,-17.573445592098,-17.4857146330988,
-17.2174499967721,-17.1637028159425),.UNSPECIFIED.);
#30592=B_SPLINE_CURVE_WITH_KNOTS('',3,(#217675,#217676,#217677,#217678,
#217679,#217680,#217681,#217682,#217683,#217684,#217685,#217686,#217687,
#217688,#217689,#217690,#217691,#217692,#217693,#217694,#217695,#217696,
#217697,#217698,#217699,#217700,#217701,#217702,#217703,#217704,#217705,
#217706,#217707,#217708),.UNSPECIFIED.,.F.,.F.,(4,2,2,2,2,2,2,2,2,2,2,2,
2,2,2,2,4),(-2.86068452297866,-2.77773294211803,-2.63630062493424,-2.44865158052864,
-2.18043666205413,-1.82474834886011,-1.65128159569772,-1.4809693172972,
-1.31094241874573,-1.14993202613478,-0.990511201393968,-0.838687969453853,
-0.65849182006884,-0.576298702112474,-0.435211787338084,-0.287957514444663,
-9.99999996587064E-7),.UNSPECIFIED.);
#30593=B_SPLINE_CURVE_WITH_KNOTS('',3,(#217710,#217711,#217712,#217713,
#217714,#217715,#217716,#217717,#217718,#217719,#217720,#217721,#217722,
#217723,#217724,#217725,#217726,#217727,#217728,#217729,#217730,#217731),
 .UNSPECIFIED.,.F.,.F.,(4,2,2,2,2,2,2,2,2,2,4),(-1.678391897345,-1.54864602532634,
-1.419721708183,-1.17041427886277,-1.02310064103662,-0.854629816400835,
-0.705938572535618,-0.530158421676784,-0.264651666630037,-0.134283710524161,
-0.000635529299139109),.UNSPECIFIED.);
#30594=B_SPLINE_CURVE_WITH_KNOTS('',3,(#217733,#217734,#217735,#217736),
 .UNSPECIFIED.,.F.,.F.,(4,4),(0.,1.),.UNSPECIFIED.);
#30595=B_SPLINE_CURVE_WITH_KNOTS('',3,(#217738,#217739,#217740,#217741,
#217742,#217743,#217744,#217745,#217746,#217747,#217748,#217749,#217750,
#217751,#217752,#217753,#217754,#217755,#217756,#217757,#217758,#217759),
 .UNSPECIFIED.,.F.,.F.,(4,2,2,2,2,2,2,2,2,2,4),(0.000147978863462259,0.132665880132235,
0.264039836401641,0.521001553758146,0.701578774182686,0.838995874465286,
1.11207159352395,1.25225787136096,1.4596258412934,1.56800447107715,1.67810387044742),
 .UNSPECIFIED.);
#30596=B_SPLINE_CURVE_WITH_KNOTS('',3,(#217760,#217761,#217762,#217763,
#217764,#217765,#217766,#217767,#217768,#217769,#217770,#217771,#217772,
#217773,#217774,#217775,#217776,#217777,#217778,#217779,#217780,#217781,
#217782,#217783,#217784,#217785,#217786,#217787,#217788,#217789,#217790,
#217791,#217792,#217793),.UNSPECIFIED.,.F.,.F.,(4,2,2,2,2,2,2,2,2,2,2,2,
2,2,2,2,4),(-20.0226821886523,-19.730263650116,-19.5909631962108,-19.4511634053081,
-19.3697072643866,-19.2822426050699,-19.1116277510905,-18.8907000615668,
-18.7210061060888,-18.5495596781661,-18.3786443708691,-18.2043541297755,
-17.8487913077471,-17.5467363732741,-17.3992244973413,-17.252074015242,
-17.1619514598514),.UNSPECIFIED.);
#30597=B_SPLINE_CURVE_WITH_KNOTS('',3,(#217823,#217824,#217825,#217826,
#217827,#217828,#217829,#217830,#217831,#217832,#217833,#217834,#217835,
#217836,#217837,#217838,#217839,#217840,#217841),.UNSPECIFIED.,.F.,.F.,
(4,3,3,3,3,3,4),(3.59311864544389E-15,0.188384660190751,0.240000922766575,
0.50000123041085,0.760001538055125,0.945884007472818,0.999999610267735),
 .UNSPECIFIED.);
#30598=B_SPLINE_CURVE_WITH_KNOTS('',3,(#217844,#217845,#217846,#217847,
#217848,#217849,#217850,#217851,#217852,#217853,#217854,#217855,#217856,
#217857),.UNSPECIFIED.,.F.,.F.,(4,2,2,2,2,2,4),(0.000337787465768249,0.284976578385984,
0.575874331198088,0.935643861114886,1.30221214423596,1.60875324692279,1.91914645332376),
 .UNSPECIFIED.);
#30599=B_SPLINE_CURVE_WITH_KNOTS('',3,(#218128,#218129,#218130,#218131,
#218132,#218133,#218134,#218135,#218136,#218137,#218138,#218139,#218140,
#218141,#218142,#218143,#218144,#218145,#218146,#218147,#218148,#218149,
#218150,#218151,#218152,#218153,#218154,#218155,#218156,#218157,#218158,
#218159,#218160,#218161,#218162,#218163,#218164,#218165),.UNSPECIFIED.,
 .F.,.F.,(4,2,2,2,2,2,2,2,2,2,2,2,2,2,2,2,2,2,4),(-25.3607679059522,-25.2146555775584,
-25.0721549022585,-24.7878117742293,-24.6209012665101,-24.4665570964828,
-24.2750293060982,-24.0854606330825,-23.8884468545564,-23.5513161309177,
-23.3484860585261,-23.1459344345172,-22.9908242973992,-22.8913313630438,
-22.4856788944898,-22.1092331654096,-21.9066557467446,-21.7038929328105,
-21.6906362475869),.UNSPECIFIED.);
#30600=B_SPLINE_CURVE_WITH_KNOTS('',3,(#218435,#218436,#218437,#218438,
#218439,#218440),.UNSPECIFIED.,.F.,.F.,(4,2,4),(1.30310740493471E-6,0.0653973299358593,
0.130262396001019),.UNSPECIFIED.);
#30601=B_SPLINE_CURVE_WITH_KNOTS('',3,(#218469,#218470,#218471,#218472,
#218473,#218474),.UNSPECIFIED.,.F.,.F.,(4,2,4),(-0.0180566566914932,-0.00903372775810624,
-8.36277994474979E-7),.UNSPECIFIED.);
#30602=B_SPLINE_CURVE_WITH_KNOTS('',3,(#218476,#218477,#218478,#218479,
#218480,#218481),.UNSPECIFIED.,.F.,.F.,(4,2,4),(-0.0180610510695405,-0.0090326996689314,
-5.26550411017056E-6),.UNSPECIFIED.);
#30603=B_SPLINE_CURVE_WITH_KNOTS('',3,(#218510,#218511,#218512,#218513,
#218514,#218515),.UNSPECIFIED.,.F.,.F.,(4,2,4),(0.000679919885625248,0.0656077246252304,
0.130948216318226),.UNSPECIFIED.);
#30604=B_SPLINE_CURVE_WITH_KNOTS('',3,(#219130,#219131,#219132,#219133,
#219134,#219135),.UNSPECIFIED.,.F.,.F.,(4,2,4),(1.37679441807117E-6,0.132788624167673,
0.261946710422657),.UNSPECIFIED.);
#30605=B_SPLINE_CURVE_WITH_KNOTS('',3,(#219136,#219137,#219138,#219139,
#219140,#219141),.UNSPECIFIED.,.F.,.F.,(4,2,4),(9.69834487247414E-6,0.0602748062236532,
0.119740503039193),.UNSPECIFIED.);
#30606=B_SPLINE_CURVE_WITH_KNOTS('',3,(#219154,#219155,#219156,#219157,
#219158,#219159,#219160,#219161,#219162,#219163),.UNSPECIFIED.,.F.,.F.,
(4,2,2,2,4),(2.4605588906763,2.77696986044635,3.16672845187631,3.55648704330627,
3.87289801307633),.UNSPECIFIED.);
#30607=B_SPLINE_CURVE_WITH_KNOTS('',3,(#219165,#219166,#219167,#219168,
#219169,#219170),.UNSPECIFIED.,.F.,.F.,(4,2,4),(3.76834231800082E-5,0.277014521395569,
0.555926380959157),.UNSPECIFIED.);
#30608=B_SPLINE_CURVE_WITH_KNOTS('',3,(#219200,#219201,#219202,#219203,
#219204,#219205,#219206,#219207,#219208,#219209,#219210,#219211,#219212,
#219213,#219214,#219215,#219216,#219217,#219218),.UNSPECIFIED.,.F.,.F.,
(4,3,3,3,3,3,4),(0.,0.176916349798396,0.240000637218418,0.500000956530085,
0.760001275841753,0.935051760841337,0.999999692665191),.UNSPECIFIED.);
#30609=B_SPLINE_CURVE_WITH_KNOTS('',3,(#219221,#219222,#219223,#219224,
#219225,#219226,#219227,#219228,#219229,#219230,#219231,#219232,#219233,
#219234),.UNSPECIFIED.,.F.,.F.,(4,2,2,2,2,2,4),(0.000167093672000697,0.369844031545414,
0.745935182508726,1.21004916822793,1.6809812805178,2.07272751301291,2.46807904564772),
 .UNSPECIFIED.);
#30610=B_SPLINE_CURVE_WITH_KNOTS('',3,(#219376,#219377,#219378,#219379,
#219380,#219381,#219382,#219383,#219384,#219385,#219386,#219387,#219388,
#219389,#219390,#219391,#219392,#219393,#219394,#219395,#219396,#219397,
#219398,#219399,#219400,#219401,#219402,#219403,#219404,#219405,#219406,
#219407,#219408,#219409,#219410,#219411,#219412,#219413,#219414,#219415,
#219416,#219417,#219418,#219419,#219420,#219421,#219422,#219423,#219424,
#219425,#219426,#219427,#219428,#219429,#219430,#219431,#219432,#219433,
#219434,#219435,#219436,#219437,#219438,#219439,#219440,#219441,#219442,
#219443,#219444,#219445,#219446,#219447,#219448,#219449,#219450,#219451,
#219452,#219453,#219454,#219455,#219456,#219457,#219458,#219459,#219460,
#219461,#219462,#219463,#219464,#219465,#219466,#219467,#219468,#219469,
#219470,#219471,#219472,#219473,#219474,#219475,#219476,#219477,#219478,
#219479,#219480,#219481,#219482,#219483,#219484,#219485,#219486,#219487,
#219488,#219489,#219490,#219491,#219492,#219493,#219494,#219495,#219496,
#219497,#219498,#219499,#219500,#219501,#219502,#219503,#219504,#219505,
#219506,#219507,#219508,#219509,#219510,#219511,#219512,#219513,#219514,
#219515,#219516,#219517,#219518,#219519,#219520,#219521,#219522,#219523,
#219524,#219525,#219526,#219527,#219528,#219529,#219530,#219531,#219532,
#219533,#219534,#219535,#219536,#219537,#219538,#219539,#219540,#219541,
#219542,#219543,#219544,#219545,#219546,#219547,#219548,#219549,#219550,
#219551,#219552,#219553,#219554,#219555,#219556,#219557,#219558,#219559,
#219560,#219561,#219562,#219563,#219564,#219565,#219566,#219567,#219568,
#219569,#219570,#219571,#219572,#219573,#219574,#219575,#219576,#219577,
#219578,#219579),.UNSPECIFIED.,.F.,.F.,(4,2,2,2,2,2,2,2,2,2,2,2,2,2,2,2,
2,2,2,2,2,2,2,2,2,2,2,2,2,2,2,2,2,2,2,2,2,2,2,2,2,2,2,2,2,2,2,2,2,2,2,2,
2,2,2,2,2,2,2,2,2,2,2,2,2,2,2,2,2,2,2,2,2,2,2,2,2,2,2,2,2,2,2,2,2,2,2,2,
2,2,2,2,2,2,2,2,2,2,2,2,2,4),(0.00107990836000404,0.0329071535296479,0.195893327983235,
0.355153899134427,0.434988215969284,0.642816515067203,0.737569286405069,
0.908716883287997,0.993153014806632,1.18963661554878,1.28754502541362,1.47339633011078,
1.55811137762964,1.76173951289927,1.85370473309428,2.02895304676804,2.11938121712701,
2.33665348572374,2.42297287419884,2.59661267513458,2.68840363105108,2.90216045958087,
2.987118381251,3.17342429417755,3.26349749411226,3.45824610590557,3.54619696540934,
3.73710767122859,3.83188019089672,4.03301640796955,4.11747646294057,4.30305199952714,
4.40238831720826,4.60868154567945,4.68987410554116,4.87477538213013,4.97656143376426,
5.17614663866258,5.25912879790943,5.44612356943043,5.55060337155454,5.74202887918956,
5.82728553459735,6.01648422346557,6.12403067700903,6.30698556123304,6.3948612127417,
6.59463365103844,6.70174065635423,6.86827502115102,6.95722664984312,7.16281963653449,
7.27369262138387,7.43009961028706,7.52201238463309,7.70970084887526,7.83380812634278,
7.98940531561225,8.08401417045588,8.26759687618598,8.40024551773955,8.54235988021463,
8.63766384385343,8.81511758111811,9.02203998489799,9.12411504919588,9.27578319513838,
9.43003056692406,9.6064767882247,9.70887427561559,9.85136721119973,10.0286666142249,
10.1832040085792,10.2906557513719,10.4409835696911,10.7071639943014,10.8497640573907,
11.0174209505587,11.3437940692132,11.4716454362162,11.6108663252812,11.9469480845909,
12.0272146927954,12.2685798563405,12.5116906256741,12.6535479256158,12.8550753169041,
13.2724871383448,13.4494739492565,13.619028692563,13.8159480124215,14.1806924721594,
14.3608390254965,14.4645640031877,14.7164986862713,14.8965371123671,15.2222169253479,
15.3963408756932,15.575785343045,15.9915006951352,16.2407971147128,16.4907160008511),
 .UNSPECIFIED.);
#30611=B_SPLINE_CURVE_WITH_KNOTS('',3,(#219581,#219582,#219583,#219584,
#219585,#219586,#219587,#219588,#219589,#219590,#219591,#219592,#219593,
#219594,#219595,#219596,#219597,#219598,#219599,#219600,#219601,#219602,
#219603,#219604,#219605,#219606,#219607,#219608,#219609,#219610,#219611,
#219612,#219613,#219614,#219615,#219616,#219617,#219618,#219619,#219620,
#219621,#219622,#219623,#219624,#219625,#219626,#219627,#219628,#219629,
#219630,#219631,#219632,#219633,#219634,#219635,#219636,#219637,#219638,
#219639,#219640,#219641,#219642,#219643,#219644,#219645,#219646,#219647,
#219648,#219649,#219650,#219651,#219652,#219653,#219654,#219655,#219656,
#219657,#219658,#219659,#219660,#219661,#219662,#219663,#219664,#219665),
 .UNSPECIFIED.,.F.,.F.,(4,3,3,3,3,3,3,3,3,3,3,3,3,3,3,3,3,3,3,3,3,3,3,3,
3,3,3,3,4),(0.,0.0475523396469734,0.0945933459100679,0.141741666700758,
0.188796087897991,0.23670174521744,0.246392852642554,0.25047433411042,0.297627468238015,
0.344829936037007,0.380418717175787,0.427580266675554,0.474808467309134,
0.496867832745316,0.502907306312494,0.549192807169434,0.595728951526263,
0.642323912157344,0.688682512690019,0.723451463089525,0.738537131197933,
0.747378842105526,0.752846656127323,0.801913022967692,0.827758314288042,
0.876702333074787,0.92583430503612,0.974954869279015,0.999217082393009),
 .UNSPECIFIED.);
#30612=B_SPLINE_CURVE_WITH_KNOTS('',3,(#219667,#219668,#219669,#219670),
 .UNSPECIFIED.,.F.,.F.,(4,4),(-0.000244606540982073,0.),.UNSPECIFIED.);
#30613=B_SPLINE_CURVE_WITH_KNOTS('',3,(#219671,#219672,#219673,#219674,
#219675,#219676,#219677,#219678,#219679,#219680,#219681,#219682,#219683,
#219684,#219685,#219686,#219687,#219688,#219689,#219690,#219691,#219692,
#219693,#219694,#219695,#219696,#219697,#219698,#219699,#219700,#219701,
#219702,#219703,#219704,#219705,#219706,#219707,#219708,#219709,#219710,
#219711,#219712,#219713,#219714,#219715,#219716,#219717,#219718,#219719,
#219720,#219721,#219722,#219723,#219724,#219725,#219726,#219727,#219728,
#219729,#219730,#219731,#219732,#219733,#219734,#219735,#219736,#219737,
#219738,#219739,#219740,#219741,#219742,#219743,#219744,#219745,#219746,
#219747,#219748,#219749,#219750,#219751,#219752,#219753,#219754,#219755,
#219756,#219757,#219758,#219759,#219760,#219761,#219762,#219763,#219764,
#219765,#219766,#219767,#219768,#219769,#219770,#219771,#219772,#219773,
#219774,#219775,#219776,#219777,#219778,#219779,#219780,#219781,#219782,
#219783,#219784,#219785,#219786,#219787,#219788,#219789,#219790,#219791,
#219792,#219793,#219794,#219795,#219796,#219797,#219798,#219799,#219800,
#219801,#219802,#219803,#219804,#219805,#219806,#219807,#219808,#219809,
#219810,#219811,#219812,#219813,#219814,#219815,#219816,#219817,#219818,
#219819,#219820,#219821,#219822,#219823,#219824,#219825,#219826,#219827,
#219828,#219829,#219830,#219831,#219832,#219833,#219834,#219835,#219836,
#219837,#219838,#219839,#219840,#219841,#219842,#219843,#219844,#219845,
#219846,#219847,#219848),.UNSPECIFIED.,.F.,.F.,(4,2,2,2,2,2,2,2,2,2,2,2,
2,2,2,2,2,2,2,2,2,2,2,2,2,2,2,2,2,2,2,2,2,2,2,2,2,2,2,2,2,2,2,2,2,2,2,2,
2,2,2,2,2,2,2,2,2,2,2,2,2,2,2,2,2,2,2,2,2,2,2,2,2,2,2,2,2,2,2,2,2,2,2,2,
2,2,2,2,4),(-17.8874346102476,-17.5294919404532,-17.186048243388,-16.9295394700842,
-16.809249288478,-16.1896824712227,-15.8340272537738,-15.2083864406208,
-14.9204681110229,-14.3899595900006,-14.1556344483798,-13.9783598065547,
-13.7492496006877,-13.5994074639487,-13.4666029322114,-13.366607942251,
-13.1542141543599,-12.9906873702076,-12.8875365109189,-12.735910683424,
-12.5879560880447,-12.4262389066032,-12.3252101181408,-12.1497599740358,
-12.0316602778982,-11.8443326767789,-11.7509492083987,-11.5889580966796,
-11.4836693199074,-11.2966545630751,-11.1924870275934,-11.0521608685493,
-10.9450814860021,-10.7612433258151,-10.6366324077902,-10.486559685584,
-10.3465040629413,-10.1283588143423,-10.018252455382,-9.89616481200024,
-9.58905421181,-9.07549190175552,-8.68076130992365,-8.46605691770783,-8.01018323269793,
-7.62107621005051,-7.24137219646125,-6.65939456134288,-6.42566825697358,
-6.19571944233163,-5.93321022343852,-5.81507259106976,-5.63942976266636,
-5.45310433687737,-5.26007640926833,-5.15380952307374,-5.03637349809843,
-4.82334403415963,-4.68443024677056,-4.54527121635446,-4.41726995679759,
-4.2451953431367,-4.13877004673389,-4.00127907200663,-3.88561719143933,
-3.73605126423849,-3.64032051174758,-3.46696552173283,-3.36568283466282,
-3.21304464574176,-3.10894067512282,-2.9301644852829,-2.83463383875695,
-2.67405588965988,-2.53885135281524,-2.39350009266555,-2.2994834121668,
-2.13842813199059,-1.95939869233589,-1.8284100896886,-1.69294839797854,
-1.55186298560815,-1.33346072701374,-1.18729433138974,-0.99438201782296,
-0.767650200561418,-0.680987224727819,-0.341206102852197,-0.000193437912458331),
 .UNSPECIFIED.);
#30614=B_SPLINE_CURVE_WITH_KNOTS('',3,(#220118,#220119,#220120,#220121,
#220122,#220123),.UNSPECIFIED.,.F.,.F.,(4,2,4),(-0.1310037054835,-0.0656099052540244,
-3.86587579881701E-6),.UNSPECIFIED.);
#30615=B_SPLINE_CURVE_WITH_KNOTS('',3,(#220125,#220126,#220127,#220128,
#220129,#220130,#220131,#220132,#220133,#220134,#220135,#220136,#220137,
#220138,#220139,#220140,#220141,#220142,#220143,#220144,#220145,#220146,
#220147,#220148,#220149,#220150,#220151,#220152,#220153,#220154,#220155,
#220156,#220157,#220158,#220159,#220160,#220161,#220162,#220163,#220164,
#220165,#220166,#220167,#220168,#220169,#220170,#220171,#220172,#220173,
#220174,#220175,#220176,#220177,#220178,#220179,#220180,#220181,#220182,
#220183,#220184),.UNSPECIFIED.,.F.,.F.,(4,2,2,2,2,2,2,2,2,2,2,2,2,2,2,2,
2,2,2,2,2,2,2,2,2,2,2,2,2,4),(-6.15788331278694,-6.06443252815276,-5.83610230741255,
-5.60523089161273,-5.31363699842867,-5.18840170216816,-4.94062642991686,
-4.68241759985902,-4.557318904294,-4.30670853548563,-4.0646490808404,-3.80643899426189,
-3.68163245799914,-3.43051020036923,-3.16947422123254,-2.91133046902137,
-2.78563835863885,-2.52772346543546,-2.25261630655297,-2.12766163183034,
-1.76426794976545,-1.63827805735133,-1.47827926244735,-1.22738320571347,
-0.974993743424404,-0.716796513895058,-0.539736803061585,-0.273532248004654,
-0.137263400187583,-3.49173976057398E-5),.UNSPECIFIED.);
#30616=B_SPLINE_CURVE_WITH_KNOTS('',3,(#220213,#220214,#220215,#220216,
#220217,#220218),.UNSPECIFIED.,.F.,.F.,(4,2,4),(-0.0180614175475569,-0.00903747414230207,
-8.0491419894641E-7),.UNSPECIFIED.);
#30617=B_SPLINE_CURVE_WITH_KNOTS('',3,(#220219,#220220,#220221,#220222,
#220223,#220224,#220225,#220226,#220227,#220228,#220229,#220230,#220231,
#220232),.UNSPECIFIED.,.F.,.F.,(4,2,2,2,2,2,4),(1.00000038962293E-6,0.377507126467076,
0.760172295625583,1.01061719312921,1.51716116734717,1.76732387692728,2.02167921549914),
 .UNSPECIFIED.);
#30618=B_SPLINE_CURVE_WITH_KNOTS('',3,(#220234,#220235,#220236,#220237,
#220238,#220239),.UNSPECIFIED.,.F.,.F.,(4,2,4),(-0.0180670199973735,-0.00903616121666685,
-6.43699295097665E-6),.UNSPECIFIED.);
#30619=B_SPLINE_CURVE_WITH_KNOTS('',3,(#220268,#220269,#220270,#220271,
#220272,#220273),.UNSPECIFIED.,.F.,.F.,(4,2,4),(-0.131007313205517,-0.0654519306470199,
-7.32542529301984E-6),.UNSPECIFIED.);
#30620=B_SPLINE_CURVE_WITH_KNOTS('',3,(#220542,#220543,#220544,#220545,
#220546,#220547,#220548,#220549,#220550,#220551,#220552,#220553,#220554,
#220555,#220556,#220557,#220558,#220559,#220560,#220561,#220562,#220563,
#220564,#220565,#220566,#220567,#220568,#220569,#220570,#220571,#220572,
#220573,#220574,#220575,#220576,#220577,#220578,#220579,#220580,#220581,
#220582,#220583,#220584,#220585,#220586,#220587,#220588,#220589,#220590,
#220591,#220592,#220593,#220594,#220595,#220596,#220597,#220598,#220599,
#220600,#220601,#220602,#220603,#220604,#220605,#220606,#220607,#220608,
#220609,#220610,#220611,#220612,#220613,#220614,#220615,#220616,#220617,
#220618,#220619),.UNSPECIFIED.,.F.,.F.,(4,2,2,2,2,2,2,2,2,2,2,2,2,2,2,2,
2,2,2,2,2,2,2,2,2,2,2,2,2,2,2,2,2,2,2,2,2,2,4),(-20.9311220871695,-20.8233977585101,
-20.5929681913972,-20.3351437643928,-20.1699664773702,-19.9382476421245,
-19.7022880772898,-19.4518568542575,-19.326668163532,-19.0684679733444,
-18.833648144018,-18.5758020857754,-18.450368441215,-18.1921847851807,-17.9372411480242,
-17.6862799548196,-17.5613796926949,-17.3031720422929,-17.0593174409058,
-16.808658958332,-16.6470842308963,-16.4156015810085,-16.1896008615369,
-16.0641249825309,-15.7633137741317,-15.505326382634,-15.3310206693453,
-15.0986175424629,-14.8698936276518,-14.6120684599034,-14.486738873575,
-14.2285383694322,-13.9919828079423,-13.7605082217295,-13.5444128021083,
-13.3279945079624,-13.096528614438,-12.859855499747,-12.7553010434687),
 .UNSPECIFIED.);
#30621=B_SPLINE_CURVE_WITH_KNOTS('',3,(#221031,#221032,#221033,#221034,
#221035,#221036),.UNSPECIFIED.,.F.,.F.,(4,2,4),(-0.344875729523311,-0.172579825678003,
-3.94566552332552E-5),.UNSPECIFIED.);
#30622=B_SPLINE_CURVE_WITH_KNOTS('',3,(#221037,#221038,#221039,#221040),
 .UNSPECIFIED.,.F.,.F.,(4,4),(-0.00025708205727752,0.),.UNSPECIFIED.);
#30623=B_SPLINE_CURVE_WITH_KNOTS('',3,(#221452,#221453,#221454,#221455,
#221456,#221457),.UNSPECIFIED.,.F.,.F.,(4,2,4),(-0.344703474824423,-0.172091835354088,
-0.00130738802393666),.UNSPECIFIED.);
#30624=B_SPLINE_CURVE_WITH_KNOTS('',3,(#221458,#221459,#221460,#221461),
 .UNSPECIFIED.,.F.,.F.,(4,4),(-0.00138054251313501,0.),.UNSPECIFIED.);
#30625=B_SPLINE_CURVE_WITH_KNOTS('',3,(#221488,#221489,#221490,#221491,
#221492,#221493),.UNSPECIFIED.,.F.,.F.,(4,2,4),(0.000411407934197906,0.132395690524123,
0.265296797891781),.UNSPECIFIED.);
#30626=B_SPLINE_CURVE_WITH_KNOTS('',3,(#221496,#221497,#221498,#221499),
 .UNSPECIFIED.,.F.,.F.,(4,4),(0.,0.000434666445788224),.UNSPECIFIED.);
#30627=B_SPLINE_CURVE_WITH_KNOTS('',3,(#221501,#221502,#221503,#221504,
#221505,#221506,#221507,#221508,#221509,#221510,#221511,#221512,#221513,
#221514,#221515,#221516,#221517,#221518,#221519,#221520,#221521,#221522),
 .UNSPECIFIED.,.F.,.F.,(4,2,2,2,2,2,2,2,2,2,4),(0.,0.144173778921629,0.288103676995556,
0.573727861047887,0.772563733388475,1.17379786176671,1.5750673712583,1.77392881725809,
1.91671525972691,2.13148394855007,2.34639580468754),.UNSPECIFIED.);
#30628=B_SPLINE_CURVE_WITH_KNOTS('',3,(#221523,#221524,#221525,#221526),
 .UNSPECIFIED.,.F.,.F.,(4,4),(4.93459806213273E-5,5.07374035434672E-5),
 .UNSPECIFIED.);
#30629=B_SPLINE_CURVE_WITH_KNOTS('',3,(#221605,#221606,#221607,#221608,
#221609,#221610,#221611,#221612,#221613,#221614),.UNSPECIFIED.,.F.,.F.,
(4,2,2,2,4),(2.44487072892702,2.76003095423418,3.15004164386436,3.5418883593805,
3.8553044918496),.UNSPECIFIED.);
#33552=CIRCLE('',#86061,10.25);
#33553=CIRCLE('',#86062,10.25);
#33554=CIRCLE('',#86071,13.);
#33555=CIRCLE('',#86073,13.);
#33556=CIRCLE('',#86081,13.);
#33557=CIRCLE('',#86082,13.);
#33558=CIRCLE('',#86084,12.00000442428);
#33559=CIRCLE('',#86094,9.08769033371916);
#33560=CIRCLE('',#86096,4.90285210866692);
#33561=CIRCLE('',#86104,10.25);
#33562=CIRCLE('',#86105,9.250003127107);
#33563=CIRCLE('',#86107,10.25);
#33564=CIRCLE('',#86113,11.4812930573653);
#33565=CIRCLE('',#86116,9.08769033371916);
#33566=CIRCLE('',#86121,66.65911415553);
#33567=CIRCLE('',#86122,66.65911415553);
#33568=CIRCLE('',#86123,67.66415225213);
#33569=CIRCLE('',#86125,68.);
#33570=CIRCLE('',#86126,67.66415225213);
#33571=CIRCLE('',#86131,10.5);
#33572=CIRCLE('',#86132,10.5);
#33573=CIRCLE('',#86133,10.5);
#33574=CIRCLE('',#86135,11.0000062575399);
#33575=CIRCLE('',#86139,7.75);
#33576=CIRCLE('',#86141,7.75);
#33577=CIRCLE('',#86143,8.249994983965);
#33578=CIRCLE('',#86147,66.65911415553);
#33579=CIRCLE('',#86148,67.);
#40909=VERTEX_POINT('',#212791);
#40910=VERTEX_POINT('',#212792);
#40911=VERTEX_POINT('',#212794);
#40912=VERTEX_POINT('',#212859);
#40913=VERTEX_POINT('',#212861);
#40914=VERTEX_POINT('',#212864);
#40915=VERTEX_POINT('',#212887);
#40916=VERTEX_POINT('',#212900);
#40917=VERTEX_POINT('',#212911);
#40918=VERTEX_POINT('',#212913);
#40919=VERTEX_POINT('',#212924);
#40920=VERTEX_POINT('',#212960);
#40921=VERTEX_POINT('',#212961);
#40922=VERTEX_POINT('',#213100);
#40923=VERTEX_POINT('',#213101);
#40924=VERTEX_POINT('',#213236);
#40925=VERTEX_POINT('',#213237);
#40926=VERTEX_POINT('',#213239);
#40927=VERTEX_POINT('',#213379);
#40928=VERTEX_POINT('',#213380);
#40929=VERTEX_POINT('',#213444);
#40930=VERTEX_POINT('',#213516);
#40931=VERTEX_POINT('',#213517);
#40932=VERTEX_POINT('',#213652);
#40933=VERTEX_POINT('',#213653);
#40934=VERTEX_POINT('',#213788);
#40935=VERTEX_POINT('',#213789);
#40936=VERTEX_POINT('',#213791);
#40937=VERTEX_POINT('',#213915);
#40938=VERTEX_POINT('',#213916);
#40939=VERTEX_POINT('',#213918);
#40940=VERTEX_POINT('',#213929);
#40941=VERTEX_POINT('',#213930);
#40942=VERTEX_POINT('',#213996);
#40943=VERTEX_POINT('',#213998);
#40944=VERTEX_POINT('',#214003);
#40945=VERTEX_POINT('',#214063);
#40946=VERTEX_POINT('',#214064);
#40947=VERTEX_POINT('',#214066);
#40948=VERTEX_POINT('',#214204);
#40949=VERTEX_POINT('',#214205);
#40950=VERTEX_POINT('',#214285);
#40951=VERTEX_POINT('',#214369);
#40952=VERTEX_POINT('',#214370);
#40953=VERTEX_POINT('',#214527);
#40954=VERTEX_POINT('',#214528);
#40955=VERTEX_POINT('',#214530);
#40956=VERTEX_POINT('',#214694);
#40957=VERTEX_POINT('',#214695);
#40958=VERTEX_POINT('',#214775);
#40959=VERTEX_POINT('',#214859);
#40960=VERTEX_POINT('',#214860);
#40961=VERTEX_POINT('',#215019);
#40962=VERTEX_POINT('',#215020);
#40963=VERTEX_POINT('',#215023);
#40964=VERTEX_POINT('',#215025);
#40965=VERTEX_POINT('',#215032);
#40966=VERTEX_POINT('',#215034);
#40967=VERTEX_POINT('',#215041);
#40968=VERTEX_POINT('',#215043);
#40969=VERTEX_POINT('',#215119);
#40970=VERTEX_POINT('',#215121);
#40971=VERTEX_POINT('',#215126);
#40972=VERTEX_POINT('',#215173);
#40973=VERTEX_POINT('',#215234);
#40974=VERTEX_POINT('',#215235);
#40975=VERTEX_POINT('',#215237);
#40976=VERTEX_POINT('',#215242);
#40977=VERTEX_POINT('',#215255);
#40978=VERTEX_POINT('',#215270);
#40979=VERTEX_POINT('',#215341);
#40980=VERTEX_POINT('',#215412);
#40981=VERTEX_POINT('',#215413);
#40982=VERTEX_POINT('',#215562);
#40983=VERTEX_POINT('',#215563);
#40984=VERTEX_POINT('',#215708);
#40985=VERTEX_POINT('',#215709);
#40986=VERTEX_POINT('',#215711);
#40987=VERTEX_POINT('',#215716);
#40988=VERTEX_POINT('',#215725);
#40989=VERTEX_POINT('',#215736);
#40990=VERTEX_POINT('',#215803);
#40991=VERTEX_POINT('',#215876);
#40992=VERTEX_POINT('',#215877);
#40993=VERTEX_POINT('',#216012);
#40994=VERTEX_POINT('',#216013);
#40995=VERTEX_POINT('',#216150);
#40996=VERTEX_POINT('',#216151);
#40997=VERTEX_POINT('',#216153);
#40998=VERTEX_POINT('',#216158);
#40999=VERTEX_POINT('',#216167);
#41000=VERTEX_POINT('',#216168);
#41001=VERTEX_POINT('',#216170);
#41002=VERTEX_POINT('',#216245);
#41003=VERTEX_POINT('',#216320);
#41004=VERTEX_POINT('',#216321);
#41005=VERTEX_POINT('',#216478);
#41006=VERTEX_POINT('',#216479);
#41007=VERTEX_POINT('',#216636);
#41008=VERTEX_POINT('',#216637);
#41009=VERTEX_POINT('',#216639);
#41010=VERTEX_POINT('',#216644);
#41011=VERTEX_POINT('',#216669);
#41012=VERTEX_POINT('',#216694);
#41013=VERTEX_POINT('',#216773);
#41014=VERTEX_POINT('',#216854);
#41015=VERTEX_POINT('',#216855);
#41016=VERTEX_POINT('',#217014);
#41017=VERTEX_POINT('',#217015);
#41018=VERTEX_POINT('',#217174);
#41019=VERTEX_POINT('',#217175);
#41020=VERTEX_POINT('',#217177);
#41021=VERTEX_POINT('',#217179);
#41022=VERTEX_POINT('',#217184);
#41023=VERTEX_POINT('',#217215);
#41024=VERTEX_POINT('',#217250);
#41025=VERTEX_POINT('',#217290);
#41026=VERTEX_POINT('',#217305);
#41027=VERTEX_POINT('',#217307);
#41028=VERTEX_POINT('',#217328);
#41029=VERTEX_POINT('',#217361);
#41030=VERTEX_POINT('',#217396);
#41031=VERTEX_POINT('',#217397);
#41032=VERTEX_POINT('',#217409);
#41033=VERTEX_POINT('',#217411);
#41034=VERTEX_POINT('',#217423);
#41035=VERTEX_POINT('',#217430);
#41036=VERTEX_POINT('',#217432);
#41037=VERTEX_POINT('',#217501);
#41038=VERTEX_POINT('',#217561);
#41039=VERTEX_POINT('',#217616);
#41040=VERTEX_POINT('',#217674);
#41041=VERTEX_POINT('',#217709);
#41042=VERTEX_POINT('',#217732);
#41043=VERTEX_POINT('',#217737);
#41044=VERTEX_POINT('',#217822);
#41045=VERTEX_POINT('',#217842);
#41046=VERTEX_POINT('',#218126);
#41047=VERTEX_POINT('',#219143);
#41048=VERTEX_POINT('',#219144);
#41049=VERTEX_POINT('',#219146);
#41050=VERTEX_POINT('',#219152);
#41051=VERTEX_POINT('',#219199);
#41052=VERTEX_POINT('',#219219);
#41053=VERTEX_POINT('',#219375);
#41054=VERTEX_POINT('',#219580);
#41055=VERTEX_POINT('',#219666);
#41056=VERTEX_POINT('',#220117);
#41057=VERTEX_POINT('',#221030);
#41058=VERTEX_POINT('',#221451);
#41059=VERTEX_POINT('',#221463);
#41060=VERTEX_POINT('',#221464);
#41061=VERTEX_POINT('',#221466);
#41062=VERTEX_POINT('',#221471);
#41063=VERTEX_POINT('',#221477);
#41064=VERTEX_POINT('',#221480);
#41065=VERTEX_POINT('',#221484);
#41066=VERTEX_POINT('',#221495);
#41067=VERTEX_POINT('',#221500);
#41068=VERTEX_POINT('',#221604);
#52237=EDGE_CURVE('',#40909,#40910,#9707,.T.);
#52238=EDGE_CURVE('',#40909,#40911,#30485,.F.);
#52239=EDGE_CURVE('',#40911,#40912,#9708,.T.);
#52240=EDGE_CURVE('',#40912,#40913,#33552,.T.);
#52241=EDGE_CURVE('',#40913,#40912,#33553,.T.);
#52242=EDGE_CURVE('',#40911,#40914,#30486,.F.);
#52243=EDGE_CURVE('',#40914,#40915,#30487,.T.);
#52244=EDGE_CURVE('',#40915,#40916,#30488,.T.);
#52245=EDGE_CURVE('',#40916,#40917,#9709,.T.);
#52246=EDGE_CURVE('',#40917,#40918,#30489,.T.);
#52247=EDGE_CURVE('',#40918,#40919,#30490,.T.);
#52248=EDGE_CURVE('',#40919,#40910,#30491,.F.);
#52249=EDGE_CURVE('',#40920,#40921,#9710,.T.);
#52250=EDGE_CURVE('',#40920,#40909,#30492,.F.);
#52251=EDGE_CURVE('',#40910,#40921,#30493,.F.);
#52252=EDGE_CURVE('',#40922,#40923,#9711,.T.);
#52253=EDGE_CURVE('',#40922,#40920,#30494,.F.);
#52254=EDGE_CURVE('',#40921,#40923,#30495,.F.);
#52255=EDGE_CURVE('',#40924,#40925,#9712,.T.);
#52256=EDGE_CURVE('',#40924,#40926,#30496,.F.);
#52257=EDGE_CURVE('',#40926,#40922,#30497,.F.);
#52258=EDGE_CURVE('',#40923,#40925,#30498,.F.);
#52259=EDGE_CURVE('',#40927,#40928,#9713,.T.);
#52260=EDGE_CURVE('',#40927,#40924,#30499,.F.);
#52261=EDGE_CURVE('',#40925,#40929,#30500,.F.);
#52262=EDGE_CURVE('',#40929,#40928,#30501,.F.);
#52263=EDGE_CURVE('',#40930,#40931,#9714,.T.);
#52264=EDGE_CURVE('',#40930,#40927,#30502,.F.);
#52265=EDGE_CURVE('',#40928,#40931,#30503,.F.);
#52266=EDGE_CURVE('',#40932,#40933,#9715,.T.);
#52267=EDGE_CURVE('',#40932,#40930,#30504,.F.);
#52268=EDGE_CURVE('',#40931,#40933,#30505,.F.);
#52269=EDGE_CURVE('',#40934,#40935,#9716,.T.);
#52270=EDGE_CURVE('',#40934,#40936,#30506,.T.);
#52271=EDGE_CURVE('',#40936,#40932,#30507,.F.);
#52272=EDGE_CURVE('',#40933,#40935,#30508,.F.);
#52273=EDGE_CURVE('',#40937,#40938,#9717,.T.);
#52274=EDGE_CURVE('',#40937,#40939,#30509,.T.);
#52275=EDGE_CURVE('',#40938,#40939,#33554,.T.);
#52276=EDGE_CURVE('',#40940,#40941,#9718,.T.);
#52277=EDGE_CURVE('',#40940,#40937,#30510,.T.);
#52278=EDGE_CURVE('',#40942,#40938,#33555,.T.);
#52279=EDGE_CURVE('',#40942,#40943,#30511,.T.);
#52280=EDGE_CURVE('',#40943,#40944,#30512,.T.);
#52281=EDGE_CURVE('',#40944,#40941,#30513,.F.);
#52282=EDGE_CURVE('',#40945,#40946,#9719,.T.);
#52283=EDGE_CURVE('',#40945,#40947,#30514,.T.);
#52284=EDGE_CURVE('',#40947,#40940,#30515,.T.);
#52285=EDGE_CURVE('',#40941,#40946,#30516,.F.);
#52286=EDGE_CURVE('',#40948,#40949,#9720,.T.);
#52287=EDGE_CURVE('',#40948,#40945,#30517,.T.);
#52288=EDGE_CURVE('',#40946,#40950,#30518,.F.);
#52289=EDGE_CURVE('',#40950,#40949,#30519,.F.);
#52290=EDGE_CURVE('',#40951,#40952,#9721,.T.);
#52291=EDGE_CURVE('',#40951,#40948,#30520,.T.);
#52292=EDGE_CURVE('',#40949,#40952,#30521,.F.);
#52293=EDGE_CURVE('',#40953,#40954,#9722,.T.);
#52294=EDGE_CURVE('',#40953,#40955,#30522,.F.);
#52295=EDGE_CURVE('',#40955,#40951,#30523,.T.);
#52296=EDGE_CURVE('',#40952,#40954,#30524,.F.);
#52297=EDGE_CURVE('',#40956,#40957,#9723,.T.);
#52298=EDGE_CURVE('',#40956,#40953,#30525,.F.);
#52299=EDGE_CURVE('',#40954,#40958,#30526,.F.);
#52300=EDGE_CURVE('',#40958,#40957,#30527,.F.);
#52301=EDGE_CURVE('',#40959,#40960,#9724,.T.);
#52302=EDGE_CURVE('',#40959,#40956,#30528,.F.);
#52303=EDGE_CURVE('',#40957,#40960,#30529,.F.);
#52304=EDGE_CURVE('',#40961,#40962,#33556,.T.);
#52305=EDGE_CURVE('',#40962,#40961,#33557,.T.);
#52306=EDGE_CURVE('',#40961,#40963,#9725,.T.);
#52307=EDGE_CURVE('',#40963,#40964,#30530,.T.);
#52308=EDGE_CURVE('',#40965,#40964,#9726,.T.);
#52309=EDGE_CURVE('',#40965,#40966,#30531,.T.);
#52310=EDGE_CURVE('',#40966,#40967,#9727,.T.);
#52311=EDGE_CURVE('',#40967,#40968,#30532,.F.);
#52312=EDGE_CURVE('',#40968,#40963,#30533,.T.);
#52313=EDGE_CURVE('',#40938,#40969,#9728,.T.);
#52314=EDGE_CURVE('',#40970,#40939,#30534,.T.);
#52315=EDGE_CURVE('',#40971,#40970,#30535,.F.);
#52316=EDGE_CURVE('',#40972,#40971,#33558,.T.);
#52317=EDGE_CURVE('',#40972,#40969,#30536,.T.);
#52318=EDGE_CURVE('',#40973,#40974,#9729,.T.);
#52319=EDGE_CURVE('',#40975,#40973,#30537,.F.);
#52320=EDGE_CURVE('',#40976,#40975,#30538,.T.);
#52321=EDGE_CURVE('',#40977,#40976,#9730,.T.);
#52322=EDGE_CURVE('',#40977,#40974,#30539,.T.);
#52323=EDGE_CURVE('',#40974,#40978,#30540,.T.);
#52324=EDGE_CURVE('',#40979,#40978,#9731,.T.);
#52325=EDGE_CURVE('',#40973,#40979,#30541,.F.);
#52326=EDGE_CURVE('',#40980,#40981,#9732,.T.);
#52327=EDGE_CURVE('',#40979,#40980,#30542,.F.);
#52328=EDGE_CURVE('',#40978,#40981,#30543,.T.);
#52329=EDGE_CURVE('',#40982,#40983,#9733,.T.);
#52330=EDGE_CURVE('',#40980,#40982,#30544,.F.);
#52331=EDGE_CURVE('',#40981,#40983,#30545,.T.);
#52332=EDGE_CURVE('',#40984,#40985,#9734,.T.);
#52333=EDGE_CURVE('',#40986,#40984,#30546,.F.);
#52334=EDGE_CURVE('',#40987,#40986,#30547,.T.);
#52335=EDGE_CURVE('',#40988,#40987,#9735,.T.);
#52336=EDGE_CURVE('',#40988,#40985,#30548,.T.);
#52337=EDGE_CURVE('',#40985,#40989,#30549,.T.);
#52338=EDGE_CURVE('',#40990,#40989,#9736,.T.);
#52339=EDGE_CURVE('',#40984,#40990,#30550,.F.);
#52340=EDGE_CURVE('',#40991,#40992,#9737,.T.);
#52341=EDGE_CURVE('',#40990,#40991,#30551,.F.);
#52342=EDGE_CURVE('',#40989,#40992,#30552,.T.);
#52343=EDGE_CURVE('',#40993,#40994,#9738,.T.);
#52344=EDGE_CURVE('',#40991,#40993,#30553,.F.);
#52345=EDGE_CURVE('',#40992,#40994,#30554,.T.);
#52346=EDGE_CURVE('',#40995,#40996,#9739,.T.);
#52347=EDGE_CURVE('',#40997,#40995,#30555,.T.);
#52348=EDGE_CURVE('',#40998,#40997,#30556,.T.);
#52349=EDGE_CURVE('',#40996,#40998,#33559,.T.);
#52350=EDGE_CURVE('',#40999,#41000,#9740,.T.);
#52351=EDGE_CURVE('',#40999,#41001,#30557,.T.);
#52352=EDGE_CURVE('',#41001,#41002,#33560,.T.);
#52353=EDGE_CURVE('',#41000,#41002,#30558,.F.);
#52354=EDGE_CURVE('',#41003,#41004,#9741,.T.);
#52355=EDGE_CURVE('',#41003,#40999,#30559,.T.);
#52356=EDGE_CURVE('',#41004,#41000,#30560,.F.);
#52357=EDGE_CURVE('',#41005,#41006,#9742,.T.);
#52358=EDGE_CURVE('',#41005,#41003,#30561,.T.);
#52359=EDGE_CURVE('',#41006,#41004,#30562,.F.);
#52360=EDGE_CURVE('',#41007,#41008,#9743,.T.);
#52361=EDGE_CURVE('',#41007,#41009,#30563,.T.);
#52362=EDGE_CURVE('',#41009,#41010,#30564,.T.);
#52363=EDGE_CURVE('',#41010,#41011,#9744,.T.);
#52364=EDGE_CURVE('',#41008,#41011,#30565,.T.);
#52365=EDGE_CURVE('',#41012,#41008,#30566,.F.);
#52366=EDGE_CURVE('',#41013,#41012,#9745,.T.);
#52367=EDGE_CURVE('',#41013,#41007,#30567,.T.);
#52368=EDGE_CURVE('',#41014,#41015,#9746,.T.);
#52369=EDGE_CURVE('',#41014,#41013,#30568,.T.);
#52370=EDGE_CURVE('',#41015,#41012,#30569,.F.);
#52371=EDGE_CURVE('',#41016,#41017,#9747,.T.);
#52372=EDGE_CURVE('',#41016,#41014,#30570,.T.);
#52373=EDGE_CURVE('',#41017,#41015,#30571,.F.);
#52374=EDGE_CURVE('',#41018,#41019,#9748,.T.);
#52375=EDGE_CURVE('',#41018,#41020,#33561,.T.);
#52376=EDGE_CURVE('',#41020,#41021,#30572,.T.);
#52377=EDGE_CURVE('',#41022,#41021,#30573,.T.);
#52378=EDGE_CURVE('',#41023,#41022,#30574,.T.);
#52379=EDGE_CURVE('',#41024,#41023,#33562,.T.);
#52380=EDGE_CURVE('',#41024,#41019,#30575,.T.);
#52381=EDGE_CURVE('',#41019,#41025,#30576,.T.);
#52382=EDGE_CURVE('',#41025,#41018,#33563,.T.);
#52383=EDGE_CURVE('',#41026,#41026,#2699,.T.);
#52384=EDGE_CURVE('',#41026,#41027,#9749,.T.);
#52385=EDGE_CURVE('',#41027,#41027,#2700,.T.);
#52386=EDGE_CURVE('',#41002,#41017,#30577,.F.);
#52387=EDGE_CURVE('',#41001,#41016,#30578,.T.);
#52388=EDGE_CURVE('',#41028,#41006,#30579,.F.);
#52389=EDGE_CURVE('',#41029,#41028,#33564,.T.);
#52390=EDGE_CURVE('',#41029,#41005,#30580,.T.);
#52391=EDGE_CURVE('',#41030,#41031,#30581,.T.);
#52392=EDGE_CURVE('',#41031,#41032,#9750,.T.);
#52393=EDGE_CURVE('',#41032,#41033,#30582,.T.);
#52394=EDGE_CURVE('',#41033,#41034,#30583,.T.);
#52395=EDGE_CURVE('',#41030,#41034,#9751,.T.);
#52396=EDGE_CURVE('',#41035,#40996,#33565,.T.);
#52397=EDGE_CURVE('',#41035,#41036,#30584,.T.);
#52398=EDGE_CURVE('',#41036,#40988,#30585,.T.);
#52399=EDGE_CURVE('',#41037,#40987,#30586,.T.);
#52400=EDGE_CURVE('',#40995,#41037,#30587,.T.);
#52401=EDGE_CURVE('',#40994,#41038,#30588,.T.);
#52402=EDGE_CURVE('',#41038,#40977,#30589,.T.);
#52403=EDGE_CURVE('',#41039,#40976,#30590,.T.);
#52404=EDGE_CURVE('',#40993,#41039,#30591,.F.);
#52405=EDGE_CURVE('',#40983,#41040,#30592,.T.);
#52406=EDGE_CURVE('',#41040,#41041,#30593,.T.);
#52407=EDGE_CURVE('',#41041,#41042,#30594,.T.);
#52408=EDGE_CURVE('',#41043,#41042,#30595,.T.);
#52409=EDGE_CURVE('',#40982,#41043,#30596,.F.);
#52410=EDGE_CURVE('',#41041,#41044,#30597,.T.);
#52411=EDGE_CURVE('',#41044,#41045,#9752,.T.);
#52412=EDGE_CURVE('',#41042,#41045,#30598,.T.);
#52413=EDGE_CURVE('',#41046,#40988,#9753,.T.);
#52414=EDGE_CURVE('',#40935,#41046,#30599,.F.);
#52415=EDGE_CURVE('',#40929,#40977,#9754,.T.);
#52416=EDGE_CURVE('',#40919,#41041,#30600,.T.);
#52417=EDGE_CURVE('',#40917,#41044,#30601,.T.);
#52418=EDGE_CURVE('',#41045,#40916,#30602,.T.);
#52419=EDGE_CURVE('',#41042,#40914,#30603,.T.);
#52420=EDGE_CURVE('',#40976,#40926,#9755,.T.);
#52421=EDGE_CURVE('',#40987,#40936,#9756,.T.);
#52422=EDGE_CURVE('',#41023,#41035,#30604,.T.);
#52423=EDGE_CURVE('',#41046,#41020,#30605,.T.);
#52424=EDGE_CURVE('',#41047,#41048,#9757,.T.);
#52425=EDGE_CURVE('',#41049,#41047,#33566,.T.);
#52426=EDGE_CURVE('',#41030,#41049,#33567,.T.);
#52427=EDGE_CURVE('',#41048,#41034,#33568,.T.);
#52428=EDGE_CURVE('',#40962,#41033,#33569,.T.);
#52429=EDGE_CURVE('',#41032,#41050,#33570,.T.);
#52430=EDGE_CURVE('',#41048,#41050,#30606,.T.);
#52431=EDGE_CURVE('',#40969,#40942,#30607,.T.);
#52432=EDGE_CURVE('',#41010,#41051,#30608,.T.);
#52433=EDGE_CURVE('',#41051,#41052,#9758,.T.);
#52434=EDGE_CURVE('',#41011,#41052,#30609,.T.);
#52435=EDGE_CURVE('',#41053,#41028,#30610,.T.);
#52436=EDGE_CURVE('',#41054,#41053,#30611,.T.);
#52437=EDGE_CURVE('',#41054,#41055,#30612,.T.);
#52438=EDGE_CURVE('',#41055,#41029,#30613,.T.);
#52439=EDGE_CURVE('',#41056,#41010,#30614,.T.);
#52440=EDGE_CURVE('',#40955,#41001,#9759,.T.);
#52441=EDGE_CURVE('',#41056,#40959,#30615,.F.);
#52442=EDGE_CURVE('',#40965,#41051,#30616,.T.);
#52443=EDGE_CURVE('',#40966,#41056,#30617,.T.);
#52444=EDGE_CURVE('',#41052,#40964,#30618,.T.);
#52445=EDGE_CURVE('',#41011,#40968,#30619,.T.);
#52446=EDGE_CURVE('',#40960,#40967,#30620,.F.);
#52447=EDGE_CURVE('',#41002,#40958,#9760,.T.);
#52448=EDGE_CURVE('',#41028,#40950,#9761,.T.);
#52449=EDGE_CURVE('',#41057,#40972,#30621,.T.);
#52450=EDGE_CURVE('',#41057,#41053,#30622,.T.);
#52451=EDGE_CURVE('',#40947,#41029,#9762,.T.);
#52452=EDGE_CURVE('',#41058,#41055,#30623,.T.);
#52453=EDGE_CURVE('',#41058,#40971,#30624,.T.);
#52454=EDGE_CURVE('',#41059,#41060,#33571,.T.);
#52455=EDGE_CURVE('',#41059,#41061,#9763,.T.);
#52456=EDGE_CURVE('',#41061,#41061,#33572,.T.);
#52457=EDGE_CURVE('',#41060,#41059,#33573,.T.);
#52458=EDGE_CURVE('',#41060,#41062,#9764,.T.);
#52459=EDGE_CURVE('',#41062,#41062,#33574,.T.);
#52460=EDGE_CURVE('',#41063,#41063,#33575,.T.);
#52461=EDGE_CURVE('',#41063,#41064,#9765,.T.);
#52462=EDGE_CURVE('',#41064,#41064,#33576,.T.);
#52463=EDGE_CURVE('',#41064,#41065,#9766,.T.);
#52464=EDGE_CURVE('',#41065,#41065,#33577,.T.);
#52465=EDGE_CURVE('',#40998,#41024,#30625,.T.);
#52466=EDGE_CURVE('',#41025,#41066,#30626,.T.);
#52467=EDGE_CURVE('',#41066,#41067,#30627,.T.);
#52468=EDGE_CURVE('',#41067,#40934,#30628,.T.);
#52469=EDGE_CURVE('',#41068,#41047,#30629,.T.);
#52470=EDGE_CURVE('',#41068,#41031,#33578,.T.);
#52471=EDGE_CURVE('',#41049,#40913,#33579,.T.);
#52472=EDGE_CURVE('',#41068,#41050,#9767,.T.);
#74809=ORIENTED_EDGE('',*,*,#52237,.F.);
#74810=ORIENTED_EDGE('',*,*,#52238,.T.);
#74811=ORIENTED_EDGE('',*,*,#52239,.T.);
#74812=ORIENTED_EDGE('',*,*,#52240,.T.);
#74813=ORIENTED_EDGE('',*,*,#52241,.T.);
#74814=ORIENTED_EDGE('',*,*,#52239,.F.);
#74815=ORIENTED_EDGE('',*,*,#52242,.T.);
#74816=ORIENTED_EDGE('',*,*,#52243,.T.);
#74817=ORIENTED_EDGE('',*,*,#52244,.T.);
#74818=ORIENTED_EDGE('',*,*,#52245,.T.);
#74819=ORIENTED_EDGE('',*,*,#52246,.T.);
#74820=ORIENTED_EDGE('',*,*,#52247,.T.);
#74821=ORIENTED_EDGE('',*,*,#52248,.T.);
#74822=ORIENTED_EDGE('',*,*,#52249,.F.);
#74823=ORIENTED_EDGE('',*,*,#52250,.T.);
#74824=ORIENTED_EDGE('',*,*,#52237,.T.);
#74825=ORIENTED_EDGE('',*,*,#52251,.T.);
#74826=ORIENTED_EDGE('',*,*,#52252,.F.);
#74827=ORIENTED_EDGE('',*,*,#52253,.T.);
#74828=ORIENTED_EDGE('',*,*,#52249,.T.);
#74829=ORIENTED_EDGE('',*,*,#52254,.T.);
#74830=ORIENTED_EDGE('',*,*,#52255,.F.);
#74831=ORIENTED_EDGE('',*,*,#52256,.T.);
#74832=ORIENTED_EDGE('',*,*,#52257,.T.);
#74833=ORIENTED_EDGE('',*,*,#52252,.T.);
#74834=ORIENTED_EDGE('',*,*,#52258,.T.);
#74835=ORIENTED_EDGE('',*,*,#52259,.F.);
#74836=ORIENTED_EDGE('',*,*,#52260,.T.);
#74837=ORIENTED_EDGE('',*,*,#52255,.T.);
#74838=ORIENTED_EDGE('',*,*,#52261,.T.);
#74839=ORIENTED_EDGE('',*,*,#52262,.T.);
#74840=ORIENTED_EDGE('',*,*,#52263,.F.);
#74841=ORIENTED_EDGE('',*,*,#52264,.T.);
#74842=ORIENTED_EDGE('',*,*,#52259,.T.);
#74843=ORIENTED_EDGE('',*,*,#52265,.T.);
#74844=ORIENTED_EDGE('',*,*,#52266,.F.);
#74845=ORIENTED_EDGE('',*,*,#52267,.T.);
#74846=ORIENTED_EDGE('',*,*,#52263,.T.);
#74847=ORIENTED_EDGE('',*,*,#52268,.T.);
#74848=ORIENTED_EDGE('',*,*,#52269,.F.);
#74849=ORIENTED_EDGE('',*,*,#52270,.T.);
#74850=ORIENTED_EDGE('',*,*,#52271,.T.);
#74851=ORIENTED_EDGE('',*,*,#52266,.T.);
#74852=ORIENTED_EDGE('',*,*,#52272,.T.);
#74853=ORIENTED_EDGE('',*,*,#52273,.F.);
#74854=ORIENTED_EDGE('',*,*,#52274,.T.);
#74855=ORIENTED_EDGE('',*,*,#52275,.F.);
#74856=ORIENTED_EDGE('',*,*,#52276,.F.);
#74857=ORIENTED_EDGE('',*,*,#52277,.T.);
#74858=ORIENTED_EDGE('',*,*,#52273,.T.);
#74859=ORIENTED_EDGE('',*,*,#52278,.F.);
#74860=ORIENTED_EDGE('',*,*,#52279,.T.);
#74861=ORIENTED_EDGE('',*,*,#52280,.T.);
#74862=ORIENTED_EDGE('',*,*,#52281,.T.);
#74863=ORIENTED_EDGE('',*,*,#52282,.F.);
#74864=ORIENTED_EDGE('',*,*,#52283,.T.);
#74865=ORIENTED_EDGE('',*,*,#52284,.T.);
#74866=ORIENTED_EDGE('',*,*,#52276,.T.);
#74867=ORIENTED_EDGE('',*,*,#52285,.T.);
#74868=ORIENTED_EDGE('',*,*,#52286,.F.);
#74869=ORIENTED_EDGE('',*,*,#52287,.T.);
#74870=ORIENTED_EDGE('',*,*,#52282,.T.);
#74871=ORIENTED_EDGE('',*,*,#52288,.T.);
#74872=ORIENTED_EDGE('',*,*,#52289,.T.);
#74873=ORIENTED_EDGE('',*,*,#52290,.F.);
#74874=ORIENTED_EDGE('',*,*,#52291,.T.);
#74875=ORIENTED_EDGE('',*,*,#52286,.T.);
#74876=ORIENTED_EDGE('',*,*,#52292,.T.);
#74877=ORIENTED_EDGE('',*,*,#52293,.F.);
#74878=ORIENTED_EDGE('',*,*,#52294,.T.);
#74879=ORIENTED_EDGE('',*,*,#52295,.T.);
#74880=ORIENTED_EDGE('',*,*,#52290,.T.);
#74881=ORIENTED_EDGE('',*,*,#52296,.T.);
#74882=ORIENTED_EDGE('',*,*,#52297,.F.);
#74883=ORIENTED_EDGE('',*,*,#52298,.T.);
#74884=ORIENTED_EDGE('',*,*,#52293,.T.);
#74885=ORIENTED_EDGE('',*,*,#52299,.T.);
#74886=ORIENTED_EDGE('',*,*,#52300,.T.);
#74887=ORIENTED_EDGE('',*,*,#52301,.F.);
#74888=ORIENTED_EDGE('',*,*,#52302,.T.);
#74889=ORIENTED_EDGE('',*,*,#52297,.T.);
#74890=ORIENTED_EDGE('',*,*,#52303,.T.);
#74891=ORIENTED_EDGE('',*,*,#52304,.T.);
#74892=ORIENTED_EDGE('',*,*,#52305,.T.);
#74893=ORIENTED_EDGE('',*,*,#52306,.T.);
#74894=ORIENTED_EDGE('',*,*,#52307,.T.);
#74895=ORIENTED_EDGE('',*,*,#52308,.F.);
#74896=ORIENTED_EDGE('',*,*,#52309,.T.);
#74897=ORIENTED_EDGE('',*,*,#52310,.T.);
#74898=ORIENTED_EDGE('',*,*,#52311,.T.);
#74899=ORIENTED_EDGE('',*,*,#52312,.T.);
#74900=ORIENTED_EDGE('',*,*,#52306,.F.);
#74901=ORIENTED_EDGE('',*,*,#52313,.F.);
#74902=ORIENTED_EDGE('',*,*,#52275,.T.);
#74903=ORIENTED_EDGE('',*,*,#52314,.F.);
#74904=ORIENTED_EDGE('',*,*,#52315,.F.);
#74905=ORIENTED_EDGE('',*,*,#52316,.F.);
#74906=ORIENTED_EDGE('',*,*,#52317,.T.);
#74907=ORIENTED_EDGE('',*,*,#52318,.F.);
#74908=ORIENTED_EDGE('',*,*,#52319,.F.);
#74909=ORIENTED_EDGE('',*,*,#52320,.F.);
#74910=ORIENTED_EDGE('',*,*,#52321,.F.);
#74911=ORIENTED_EDGE('',*,*,#52322,.T.);
#74912=ORIENTED_EDGE('',*,*,#52323,.T.);
#74913=ORIENTED_EDGE('',*,*,#52324,.F.);
#74914=ORIENTED_EDGE('',*,*,#52325,.F.);
#74915=ORIENTED_EDGE('',*,*,#52318,.T.);
#74916=ORIENTED_EDGE('',*,*,#52326,.F.);
#74917=ORIENTED_EDGE('',*,*,#52327,.F.);
#74918=ORIENTED_EDGE('',*,*,#52324,.T.);
#74919=ORIENTED_EDGE('',*,*,#52328,.T.);
#74920=ORIENTED_EDGE('',*,*,#52329,.F.);
#74921=ORIENTED_EDGE('',*,*,#52330,.F.);
#74922=ORIENTED_EDGE('',*,*,#52326,.T.);
#74923=ORIENTED_EDGE('',*,*,#52331,.T.);
#74924=ORIENTED_EDGE('',*,*,#52332,.F.);
#74925=ORIENTED_EDGE('',*,*,#52333,.F.);
#74926=ORIENTED_EDGE('',*,*,#52334,.F.);
#74927=ORIENTED_EDGE('',*,*,#52335,.F.);
#74928=ORIENTED_EDGE('',*,*,#52336,.T.);
#74929=ORIENTED_EDGE('',*,*,#52337,.T.);
#74930=ORIENTED_EDGE('',*,*,#52338,.F.);
#74931=ORIENTED_EDGE('',*,*,#52339,.F.);
#74932=ORIENTED_EDGE('',*,*,#52332,.T.);
#74933=ORIENTED_EDGE('',*,*,#52340,.F.);
#74934=ORIENTED_EDGE('',*,*,#52341,.F.);
#74935=ORIENTED_EDGE('',*,*,#52338,.T.);
#74936=ORIENTED_EDGE('',*,*,#52342,.T.);
#74937=ORIENTED_EDGE('',*,*,#52343,.F.);
#74938=ORIENTED_EDGE('',*,*,#52344,.F.);
#74939=ORIENTED_EDGE('',*,*,#52340,.T.);
#74940=ORIENTED_EDGE('',*,*,#52345,.T.);
#74941=ORIENTED_EDGE('',*,*,#52346,.F.);
#74942=ORIENTED_EDGE('',*,*,#52347,.F.);
#74943=ORIENTED_EDGE('',*,*,#52348,.F.);
#74944=ORIENTED_EDGE('',*,*,#52349,.F.);
#74945=ORIENTED_EDGE('',*,*,#52350,.F.);
#74946=ORIENTED_EDGE('',*,*,#52351,.T.);
#74947=ORIENTED_EDGE('',*,*,#52352,.T.);
#74948=ORIENTED_EDGE('',*,*,#52353,.F.);
#74949=ORIENTED_EDGE('',*,*,#52354,.F.);
#74950=ORIENTED_EDGE('',*,*,#52355,.T.);
#74951=ORIENTED_EDGE('',*,*,#52350,.T.);
#74952=ORIENTED_EDGE('',*,*,#52356,.F.);
#74953=ORIENTED_EDGE('',*,*,#52357,.F.);
#74954=ORIENTED_EDGE('',*,*,#52358,.T.);
#74955=ORIENTED_EDGE('',*,*,#52354,.T.);
#74956=ORIENTED_EDGE('',*,*,#52359,.F.);
#74957=ORIENTED_EDGE('',*,*,#52360,.F.);
#74958=ORIENTED_EDGE('',*,*,#52361,.T.);
#74959=ORIENTED_EDGE('',*,*,#52362,.T.);
#74960=ORIENTED_EDGE('',*,*,#52363,.T.);
#74961=ORIENTED_EDGE('',*,*,#52364,.F.);
#74962=ORIENTED_EDGE('',*,*,#52365,.F.);
#74963=ORIENTED_EDGE('',*,*,#52366,.F.);
#74964=ORIENTED_EDGE('',*,*,#52367,.T.);
#74965=ORIENTED_EDGE('',*,*,#52360,.T.);
#74966=ORIENTED_EDGE('',*,*,#52368,.F.);
#74967=ORIENTED_EDGE('',*,*,#52369,.T.);
#74968=ORIENTED_EDGE('',*,*,#52366,.T.);
#74969=ORIENTED_EDGE('',*,*,#52370,.F.);
#74970=ORIENTED_EDGE('',*,*,#52371,.F.);
#74971=ORIENTED_EDGE('',*,*,#52372,.T.);
#74972=ORIENTED_EDGE('',*,*,#52368,.T.);
#74973=ORIENTED_EDGE('',*,*,#52373,.F.);
#74974=ORIENTED_EDGE('',*,*,#52374,.F.);
#74975=ORIENTED_EDGE('',*,*,#52375,.T.);
#74976=ORIENTED_EDGE('',*,*,#52376,.T.);
#74977=ORIENTED_EDGE('',*,*,#52377,.F.);
#74978=ORIENTED_EDGE('',*,*,#52378,.F.);
#74979=ORIENTED_EDGE('',*,*,#52379,.F.);
#74980=ORIENTED_EDGE('',*,*,#52380,.T.);
#74981=ORIENTED_EDGE('',*,*,#52374,.T.);
#74982=ORIENTED_EDGE('',*,*,#52381,.T.);
#74983=ORIENTED_EDGE('',*,*,#52382,.T.);
#74984=ORIENTED_EDGE('',*,*,#52383,.F.);
#74985=ORIENTED_EDGE('',*,*,#52384,.T.);
#74986=ORIENTED_EDGE('',*,*,#52385,.T.);
#74987=ORIENTED_EDGE('',*,*,#52384,.F.);
#74988=ORIENTED_EDGE('',*,*,#52371,.T.);
#74989=ORIENTED_EDGE('',*,*,#52386,.F.);
#74990=ORIENTED_EDGE('',*,*,#52352,.F.);
#74991=ORIENTED_EDGE('',*,*,#52387,.T.);
#74992=ORIENTED_EDGE('',*,*,#52357,.T.);
#74993=ORIENTED_EDGE('',*,*,#52388,.F.);
#74994=ORIENTED_EDGE('',*,*,#52389,.F.);
#74995=ORIENTED_EDGE('',*,*,#52390,.T.);
#74996=ORIENTED_EDGE('',*,*,#52391,.T.);
#74997=ORIENTED_EDGE('',*,*,#52392,.T.);
#74998=ORIENTED_EDGE('',*,*,#52393,.T.);
#74999=ORIENTED_EDGE('',*,*,#52394,.T.);
#75000=ORIENTED_EDGE('',*,*,#52395,.F.);
#75001=ORIENTED_EDGE('',*,*,#52346,.T.);
#75002=ORIENTED_EDGE('',*,*,#52396,.F.);
#75003=ORIENTED_EDGE('',*,*,#52397,.T.);
#75004=ORIENTED_EDGE('',*,*,#52398,.T.);
#75005=ORIENTED_EDGE('',*,*,#52335,.T.);
#75006=ORIENTED_EDGE('',*,*,#52399,.F.);
#75007=ORIENTED_EDGE('',*,*,#52400,.F.);
#75008=ORIENTED_EDGE('',*,*,#52343,.T.);
#75009=ORIENTED_EDGE('',*,*,#52401,.T.);
#75010=ORIENTED_EDGE('',*,*,#52402,.T.);
#75011=ORIENTED_EDGE('',*,*,#52321,.T.);
#75012=ORIENTED_EDGE('',*,*,#52403,.F.);
#75013=ORIENTED_EDGE('',*,*,#52404,.F.);
#75014=ORIENTED_EDGE('',*,*,#52329,.T.);
#75015=ORIENTED_EDGE('',*,*,#52405,.T.);
#75016=ORIENTED_EDGE('',*,*,#52406,.T.);
#75017=ORIENTED_EDGE('',*,*,#52407,.T.);
#75018=ORIENTED_EDGE('',*,*,#52408,.F.);
#75019=ORIENTED_EDGE('',*,*,#52409,.F.);
#75020=ORIENTED_EDGE('',*,*,#52410,.T.);
#75021=ORIENTED_EDGE('',*,*,#52411,.T.);
#75022=ORIENTED_EDGE('',*,*,#52412,.F.);
#75023=ORIENTED_EDGE('',*,*,#52407,.F.);
#75024=ORIENTED_EDGE('',*,*,#52336,.F.);
#75025=ORIENTED_EDGE('',*,*,#52413,.F.);
#75026=ORIENTED_EDGE('',*,*,#52414,.F.);
#75027=ORIENTED_EDGE('',*,*,#52272,.F.);
#75028=ORIENTED_EDGE('',*,*,#52268,.F.);
#75029=ORIENTED_EDGE('',*,*,#52265,.F.);
#75030=ORIENTED_EDGE('',*,*,#52262,.F.);
#75031=ORIENTED_EDGE('',*,*,#52415,.T.);
#75032=ORIENTED_EDGE('',*,*,#52402,.F.);
#75033=ORIENTED_EDGE('',*,*,#52401,.F.);
#75034=ORIENTED_EDGE('',*,*,#52345,.F.);
#75035=ORIENTED_EDGE('',*,*,#52342,.F.);
#75036=ORIENTED_EDGE('',*,*,#52337,.F.);
#75037=ORIENTED_EDGE('',*,*,#52322,.F.);
#75038=ORIENTED_EDGE('',*,*,#52415,.F.);
#75039=ORIENTED_EDGE('',*,*,#52261,.F.);
#75040=ORIENTED_EDGE('',*,*,#52258,.F.);
#75041=ORIENTED_EDGE('',*,*,#52254,.F.);
#75042=ORIENTED_EDGE('',*,*,#52251,.F.);
#75043=ORIENTED_EDGE('',*,*,#52248,.F.);
#75044=ORIENTED_EDGE('',*,*,#52416,.T.);
#75045=ORIENTED_EDGE('',*,*,#52406,.F.);
#75046=ORIENTED_EDGE('',*,*,#52405,.F.);
#75047=ORIENTED_EDGE('',*,*,#52331,.F.);
#75048=ORIENTED_EDGE('',*,*,#52328,.F.);
#75049=ORIENTED_EDGE('',*,*,#52323,.F.);
#75050=ORIENTED_EDGE('',*,*,#52417,.T.);
#75051=ORIENTED_EDGE('',*,*,#52410,.F.);
#75052=ORIENTED_EDGE('',*,*,#52416,.F.);
#75053=ORIENTED_EDGE('',*,*,#52247,.F.);
#75054=ORIENTED_EDGE('',*,*,#52246,.F.);
#75055=ORIENTED_EDGE('',*,*,#52245,.F.);
#75056=ORIENTED_EDGE('',*,*,#52418,.F.);
#75057=ORIENTED_EDGE('',*,*,#52411,.F.);
#75058=ORIENTED_EDGE('',*,*,#52417,.F.);
#75059=ORIENTED_EDGE('',*,*,#52243,.F.);
#75060=ORIENTED_EDGE('',*,*,#52419,.F.);
#75061=ORIENTED_EDGE('',*,*,#52412,.T.);
#75062=ORIENTED_EDGE('',*,*,#52418,.T.);
#75063=ORIENTED_EDGE('',*,*,#52244,.F.);
#75064=ORIENTED_EDGE('',*,*,#52257,.F.);
#75065=ORIENTED_EDGE('',*,*,#52420,.F.);
#75066=ORIENTED_EDGE('',*,*,#52320,.T.);
#75067=ORIENTED_EDGE('',*,*,#52319,.T.);
#75068=ORIENTED_EDGE('',*,*,#52325,.T.);
#75069=ORIENTED_EDGE('',*,*,#52327,.T.);
#75070=ORIENTED_EDGE('',*,*,#52330,.T.);
#75071=ORIENTED_EDGE('',*,*,#52409,.T.);
#75072=ORIENTED_EDGE('',*,*,#52408,.T.);
#75073=ORIENTED_EDGE('',*,*,#52419,.T.);
#75074=ORIENTED_EDGE('',*,*,#52242,.F.);
#75075=ORIENTED_EDGE('',*,*,#52238,.F.);
#75076=ORIENTED_EDGE('',*,*,#52250,.F.);
#75077=ORIENTED_EDGE('',*,*,#52253,.F.);
#75078=ORIENTED_EDGE('',*,*,#52271,.F.);
#75079=ORIENTED_EDGE('',*,*,#52421,.F.);
#75080=ORIENTED_EDGE('',*,*,#52334,.T.);
#75081=ORIENTED_EDGE('',*,*,#52333,.T.);
#75082=ORIENTED_EDGE('',*,*,#52339,.T.);
#75083=ORIENTED_EDGE('',*,*,#52341,.T.);
#75084=ORIENTED_EDGE('',*,*,#52344,.T.);
#75085=ORIENTED_EDGE('',*,*,#52404,.T.);
#75086=ORIENTED_EDGE('',*,*,#52403,.T.);
#75087=ORIENTED_EDGE('',*,*,#52420,.T.);
#75088=ORIENTED_EDGE('',*,*,#52256,.F.);
#75089=ORIENTED_EDGE('',*,*,#52260,.F.);
#75090=ORIENTED_EDGE('',*,*,#52264,.F.);
#75091=ORIENTED_EDGE('',*,*,#52267,.F.);
#75092=ORIENTED_EDGE('',*,*,#52413,.T.);
#75093=ORIENTED_EDGE('',*,*,#52398,.F.);
#75094=ORIENTED_EDGE('',*,*,#52397,.F.);
#75095=ORIENTED_EDGE('',*,*,#52422,.F.);
#75096=ORIENTED_EDGE('',*,*,#52378,.T.);
#75097=ORIENTED_EDGE('',*,*,#52377,.T.);
#75098=ORIENTED_EDGE('',*,*,#52376,.F.);
#75099=ORIENTED_EDGE('',*,*,#52423,.F.);
#75100=ORIENTED_EDGE('',*,*,#52424,.F.);
#75101=ORIENTED_EDGE('',*,*,#52425,.F.);
#75102=ORIENTED_EDGE('',*,*,#52426,.F.);
#75103=ORIENTED_EDGE('',*,*,#52395,.T.);
#75104=ORIENTED_EDGE('',*,*,#52427,.F.);
#75105=ORIENTED_EDGE('',*,*,#52304,.F.);
#75106=ORIENTED_EDGE('',*,*,#52305,.F.);
#75107=ORIENTED_EDGE('',*,*,#52428,.T.);
#75108=ORIENTED_EDGE('',*,*,#52393,.F.);
#75109=ORIENTED_EDGE('',*,*,#52429,.T.);
#75110=ORIENTED_EDGE('',*,*,#52430,.F.);
#75111=ORIENTED_EDGE('',*,*,#52427,.T.);
#75112=ORIENTED_EDGE('',*,*,#52394,.F.);
#75113=ORIENTED_EDGE('',*,*,#52428,.F.);
#75114=ORIENTED_EDGE('',*,*,#52313,.T.);
#75115=ORIENTED_EDGE('',*,*,#52431,.T.);
#75116=ORIENTED_EDGE('',*,*,#52278,.T.);
#75117=ORIENTED_EDGE('',*,*,#52432,.T.);
#75118=ORIENTED_EDGE('',*,*,#52433,.T.);
#75119=ORIENTED_EDGE('',*,*,#52434,.F.);
#75120=ORIENTED_EDGE('',*,*,#52363,.F.);
#75121=ORIENTED_EDGE('',*,*,#52435,.F.);
#75122=ORIENTED_EDGE('',*,*,#52436,.F.);
#75123=ORIENTED_EDGE('',*,*,#52437,.T.);
#75124=ORIENTED_EDGE('',*,*,#52438,.T.);
#75125=ORIENTED_EDGE('',*,*,#52389,.T.);
#75126=ORIENTED_EDGE('',*,*,#52439,.T.);
#75127=ORIENTED_EDGE('',*,*,#52362,.F.);
#75128=ORIENTED_EDGE('',*,*,#52361,.F.);
#75129=ORIENTED_EDGE('',*,*,#52367,.F.);
#75130=ORIENTED_EDGE('',*,*,#52369,.F.);
#75131=ORIENTED_EDGE('',*,*,#52372,.F.);
#75132=ORIENTED_EDGE('',*,*,#52387,.F.);
#75133=ORIENTED_EDGE('',*,*,#52440,.F.);
#75134=ORIENTED_EDGE('',*,*,#52294,.F.);
#75135=ORIENTED_EDGE('',*,*,#52298,.F.);
#75136=ORIENTED_EDGE('',*,*,#52302,.F.);
#75137=ORIENTED_EDGE('',*,*,#52441,.F.);
#75138=ORIENTED_EDGE('',*,*,#52309,.F.);
#75139=ORIENTED_EDGE('',*,*,#52442,.T.);
#75140=ORIENTED_EDGE('',*,*,#52432,.F.);
#75141=ORIENTED_EDGE('',*,*,#52439,.F.);
#75142=ORIENTED_EDGE('',*,*,#52443,.F.);
#75143=ORIENTED_EDGE('',*,*,#52308,.T.);
#75144=ORIENTED_EDGE('',*,*,#52444,.F.);
#75145=ORIENTED_EDGE('',*,*,#52433,.F.);
#75146=ORIENTED_EDGE('',*,*,#52442,.F.);
#75147=ORIENTED_EDGE('',*,*,#52445,.F.);
#75148=ORIENTED_EDGE('',*,*,#52434,.T.);
#75149=ORIENTED_EDGE('',*,*,#52444,.T.);
#75150=ORIENTED_EDGE('',*,*,#52307,.F.);
#75151=ORIENTED_EDGE('',*,*,#52312,.F.);
#75152=ORIENTED_EDGE('',*,*,#52364,.T.);
#75153=ORIENTED_EDGE('',*,*,#52445,.T.);
#75154=ORIENTED_EDGE('',*,*,#52311,.F.);
#75155=ORIENTED_EDGE('',*,*,#52446,.F.);
#75156=ORIENTED_EDGE('',*,*,#52303,.F.);
#75157=ORIENTED_EDGE('',*,*,#52300,.F.);
#75158=ORIENTED_EDGE('',*,*,#52447,.F.);
#75159=ORIENTED_EDGE('',*,*,#52386,.T.);
#75160=ORIENTED_EDGE('',*,*,#52373,.T.);
#75161=ORIENTED_EDGE('',*,*,#52370,.T.);
#75162=ORIENTED_EDGE('',*,*,#52365,.T.);
#75163=ORIENTED_EDGE('',*,*,#52289,.F.);
#75164=ORIENTED_EDGE('',*,*,#52448,.F.);
#75165=ORIENTED_EDGE('',*,*,#52388,.T.);
#75166=ORIENTED_EDGE('',*,*,#52359,.T.);
#75167=ORIENTED_EDGE('',*,*,#52356,.T.);
#75168=ORIENTED_EDGE('',*,*,#52353,.T.);
#75169=ORIENTED_EDGE('',*,*,#52447,.T.);
#75170=ORIENTED_EDGE('',*,*,#52299,.F.);
#75171=ORIENTED_EDGE('',*,*,#52296,.F.);
#75172=ORIENTED_EDGE('',*,*,#52292,.F.);
#75173=ORIENTED_EDGE('',*,*,#52280,.F.);
#75174=ORIENTED_EDGE('',*,*,#52279,.F.);
#75175=ORIENTED_EDGE('',*,*,#52431,.F.);
#75176=ORIENTED_EDGE('',*,*,#52317,.F.);
#75177=ORIENTED_EDGE('',*,*,#52449,.F.);
#75178=ORIENTED_EDGE('',*,*,#52450,.T.);
#75179=ORIENTED_EDGE('',*,*,#52435,.T.);
#75180=ORIENTED_EDGE('',*,*,#52448,.T.);
#75181=ORIENTED_EDGE('',*,*,#52288,.F.);
#75182=ORIENTED_EDGE('',*,*,#52285,.F.);
#75183=ORIENTED_EDGE('',*,*,#52281,.F.);
#75184=ORIENTED_EDGE('',*,*,#52310,.F.);
#75185=ORIENTED_EDGE('',*,*,#52443,.T.);
#75186=ORIENTED_EDGE('',*,*,#52441,.T.);
#75187=ORIENTED_EDGE('',*,*,#52301,.T.);
#75188=ORIENTED_EDGE('',*,*,#52446,.T.);
#75189=ORIENTED_EDGE('',*,*,#52295,.F.);
#75190=ORIENTED_EDGE('',*,*,#52440,.T.);
#75191=ORIENTED_EDGE('',*,*,#52351,.F.);
#75192=ORIENTED_EDGE('',*,*,#52355,.F.);
#75193=ORIENTED_EDGE('',*,*,#52358,.F.);
#75194=ORIENTED_EDGE('',*,*,#52390,.F.);
#75195=ORIENTED_EDGE('',*,*,#52451,.F.);
#75196=ORIENTED_EDGE('',*,*,#52283,.F.);
#75197=ORIENTED_EDGE('',*,*,#52287,.F.);
#75198=ORIENTED_EDGE('',*,*,#52291,.F.);
#75199=ORIENTED_EDGE('',*,*,#52438,.F.);
#75200=ORIENTED_EDGE('',*,*,#52452,.F.);
#75201=ORIENTED_EDGE('',*,*,#52453,.T.);
#75202=ORIENTED_EDGE('',*,*,#52315,.T.);
#75203=ORIENTED_EDGE('',*,*,#52314,.T.);
#75204=ORIENTED_EDGE('',*,*,#52274,.F.);
#75205=ORIENTED_EDGE('',*,*,#52277,.F.);
#75206=ORIENTED_EDGE('',*,*,#52284,.F.);
#75207=ORIENTED_EDGE('',*,*,#52451,.T.);
#75208=ORIENTED_EDGE('',*,*,#52454,.F.);
#75209=ORIENTED_EDGE('',*,*,#52455,.T.);
#75210=ORIENTED_EDGE('',*,*,#52456,.T.);
#75211=ORIENTED_EDGE('',*,*,#52455,.F.);
#75212=ORIENTED_EDGE('',*,*,#52457,.F.);
#75213=ORIENTED_EDGE('',*,*,#52454,.T.);
#75214=ORIENTED_EDGE('',*,*,#52458,.T.);
#75215=ORIENTED_EDGE('',*,*,#52459,.F.);
#75216=ORIENTED_EDGE('',*,*,#52458,.F.);
#75217=ORIENTED_EDGE('',*,*,#52457,.T.);
#75218=ORIENTED_EDGE('',*,*,#52450,.F.);
#75219=ORIENTED_EDGE('',*,*,#52449,.T.);
#75220=ORIENTED_EDGE('',*,*,#52316,.T.);
#75221=ORIENTED_EDGE('',*,*,#52453,.F.);
#75222=ORIENTED_EDGE('',*,*,#52452,.T.);
#75223=ORIENTED_EDGE('',*,*,#52437,.F.);
#75224=ORIENTED_EDGE('',*,*,#52436,.T.);
#75225=ORIENTED_EDGE('',*,*,#52459,.T.);
#75226=ORIENTED_EDGE('',*,*,#52456,.F.);
#75227=ORIENTED_EDGE('',*,*,#52385,.F.);
#75228=ORIENTED_EDGE('',*,*,#52460,.T.);
#75229=ORIENTED_EDGE('',*,*,#52383,.T.);
#75230=ORIENTED_EDGE('',*,*,#52460,.F.);
#75231=ORIENTED_EDGE('',*,*,#52461,.T.);
#75232=ORIENTED_EDGE('',*,*,#52462,.F.);
#75233=ORIENTED_EDGE('',*,*,#52461,.F.);
#75234=ORIENTED_EDGE('',*,*,#52462,.T.);
#75235=ORIENTED_EDGE('',*,*,#52463,.T.);
#75236=ORIENTED_EDGE('',*,*,#52464,.F.);
#75237=ORIENTED_EDGE('',*,*,#52463,.F.);
#75238=ORIENTED_EDGE('',*,*,#52396,.T.);
#75239=ORIENTED_EDGE('',*,*,#52349,.T.);
#75240=ORIENTED_EDGE('',*,*,#52465,.T.);
#75241=ORIENTED_EDGE('',*,*,#52379,.T.);
#75242=ORIENTED_EDGE('',*,*,#52422,.T.);
#75243=ORIENTED_EDGE('',*,*,#52464,.T.);
#75244=ORIENTED_EDGE('',*,*,#52269,.T.);
#75245=ORIENTED_EDGE('',*,*,#52414,.T.);
#75246=ORIENTED_EDGE('',*,*,#52423,.T.);
#75247=ORIENTED_EDGE('',*,*,#52375,.F.);
#75248=ORIENTED_EDGE('',*,*,#52382,.F.);
#75249=ORIENTED_EDGE('',*,*,#52466,.T.);
#75250=ORIENTED_EDGE('',*,*,#52467,.T.);
#75251=ORIENTED_EDGE('',*,*,#52468,.T.);
#75252=ORIENTED_EDGE('',*,*,#52466,.F.);
#75253=ORIENTED_EDGE('',*,*,#52381,.F.);
#75254=ORIENTED_EDGE('',*,*,#52380,.F.);
#75255=ORIENTED_EDGE('',*,*,#52465,.F.);
#75256=ORIENTED_EDGE('',*,*,#52348,.T.);
#75257=ORIENTED_EDGE('',*,*,#52347,.T.);
#75258=ORIENTED_EDGE('',*,*,#52400,.T.);
#75259=ORIENTED_EDGE('',*,*,#52399,.T.);
#75260=ORIENTED_EDGE('',*,*,#52421,.T.);
#75261=ORIENTED_EDGE('',*,*,#52270,.F.);
#75262=ORIENTED_EDGE('',*,*,#52468,.F.);
#75263=ORIENTED_EDGE('',*,*,#52467,.F.);
#75264=ORIENTED_EDGE('',*,*,#52469,.F.);
#75265=ORIENTED_EDGE('',*,*,#52470,.T.);
#75266=ORIENTED_EDGE('',*,*,#52391,.F.);
#75267=ORIENTED_EDGE('',*,*,#52426,.T.);
#75268=ORIENTED_EDGE('',*,*,#52471,.T.);
#75269=ORIENTED_EDGE('',*,*,#52240,.F.);
#75270=ORIENTED_EDGE('',*,*,#52241,.F.);
#75271=ORIENTED_EDGE('',*,*,#52471,.F.);
#75272=ORIENTED_EDGE('',*,*,#52425,.T.);
#75273=ORIENTED_EDGE('',*,*,#52392,.F.);
#75274=ORIENTED_EDGE('',*,*,#52470,.F.);
#75275=ORIENTED_EDGE('',*,*,#52472,.T.);
#75276=ORIENTED_EDGE('',*,*,#52429,.F.);
#75277=ORIENTED_EDGE('',*,*,#52472,.F.);
#75278=ORIENTED_EDGE('',*,*,#52469,.T.);
#75279=ORIENTED_EDGE('',*,*,#52424,.T.);
#75280=ORIENTED_EDGE('',*,*,#52430,.T.);
#75301=SPHERICAL_SURFACE('',#86124,68.);
#75302=SPHERICAL_SURFACE('',#86146,67.);
#79238=ADVANCED_FACE('',(#23808),#2344,.T.);
#79239=ADVANCED_FACE('',(#23809),#2345,.T.);
#79240=ADVANCED_FACE('',(#23810),#2346,.T.);
#79241=ADVANCED_FACE('',(#23811),#2347,.T.);
#79242=ADVANCED_FACE('',(#23812),#2348,.T.);
#79243=ADVANCED_FACE('',(#23813),#2349,.T.);
#79244=ADVANCED_FACE('',(#23814),#2350,.T.);
#79245=ADVANCED_FACE('',(#23815),#2351,.T.);
#79246=ADVANCED_FACE('',(#23816),#2352,.T.);
#79247=ADVANCED_FACE('',(#23817),#2353,.T.);
#79248=ADVANCED_FACE('',(#23818),#2354,.T.);
#79249=ADVANCED_FACE('',(#23819),#2355,.T.);
#79250=ADVANCED_FACE('',(#23820),#2356,.T.);
#79251=ADVANCED_FACE('',(#23821),#2357,.T.);
#79252=ADVANCED_FACE('',(#23822),#2358,.T.);
#79253=ADVANCED_FACE('',(#23823),#2359,.T.);
#79254=ADVANCED_FACE('',(#23824),#2360,.T.);
#79255=ADVANCED_FACE('',(#23825),#1969,.T.);
#79256=ADVANCED_FACE('',(#23826),#2361,.T.);
#79257=ADVANCED_FACE('',(#23827),#2362,.T.);
#79258=ADVANCED_FACE('',(#23828),#2363,.T.);
#79259=ADVANCED_FACE('',(#23829),#2364,.T.);
#79260=ADVANCED_FACE('',(#23830),#2365,.T.);
#79261=ADVANCED_FACE('',(#23831),#2366,.T.);
#79262=ADVANCED_FACE('',(#23832),#2367,.T.);
#79263=ADVANCED_FACE('',(#23833),#2368,.T.);
#79264=ADVANCED_FACE('',(#23834),#2369,.T.);
#79265=ADVANCED_FACE('',(#23835),#2370,.T.);
#79266=ADVANCED_FACE('',(#23836),#2371,.T.);
#79267=ADVANCED_FACE('',(#23837),#2372,.T.);
#79268=ADVANCED_FACE('',(#23838),#2373,.T.);
#79269=ADVANCED_FACE('',(#23839),#2374,.T.);
#79270=ADVANCED_FACE('',(#23840),#2375,.T.);
#79271=ADVANCED_FACE('',(#23841),#2376,.T.);
#79272=ADVANCED_FACE('',(#23842),#1970,.T.);
#79273=ADVANCED_FACE('',(#23843),#1971,.T.);
#79274=ADVANCED_FACE('',(#23844),#2377,.F.);
#79275=ADVANCED_FACE('',(#23845),#2378,.T.);
#79276=ADVANCED_FACE('',(#23846),#2379,.T.);
#79277=ADVANCED_FACE('',(#23847),#2380,.T.);
#79278=ADVANCED_FACE('',(#23848),#2381,.T.);
#79279=ADVANCED_FACE('',(#23849),#2382,.T.);
#79280=ADVANCED_FACE('',(#23850),#2383,.T.);
#79281=ADVANCED_FACE('',(#23851),#226,.F.);
#79282=ADVANCED_FACE('',(#23852),#227,.F.);
#79283=ADVANCED_FACE('',(#23853),#228,.F.);
#79284=ADVANCED_FACE('',(#23854),#229,.F.);
#79285=ADVANCED_FACE('',(#23855),#19865,.F.);
#79286=ADVANCED_FACE('',(#23856),#230,.F.);
#79287=ADVANCED_FACE('',(#23857),#231,.F.);
#79288=ADVANCED_FACE('',(#23858),#232,.F.);
#79289=ADVANCED_FACE('',(#23859),#233,.F.);
#79290=ADVANCED_FACE('',(#23860),#19866,.T.);
#79291=ADVANCED_FACE('',(#23861),#75301,.T.);
#79292=ADVANCED_FACE('',(#23862),#1972,.T.);
#79293=ADVANCED_FACE('',(#23863),#234,.F.);
#79294=ADVANCED_FACE('',(#23864),#235,.F.);
#79295=ADVANCED_FACE('',(#23865),#236,.F.);
#79296=ADVANCED_FACE('',(#23866),#237,.F.);
#79297=ADVANCED_FACE('',(#23867),#19867,.F.);
#79298=ADVANCED_FACE('',(#23868),#238,.F.);
#79299=ADVANCED_FACE('',(#23869),#239,.F.);
#79300=ADVANCED_FACE('',(#23870),#240,.F.);
#79301=ADVANCED_FACE('',(#23871),#241,.F.);
#79302=ADVANCED_FACE('',(#23872),#2384,.T.);
#79303=ADVANCED_FACE('',(#23873),#242,.F.);
#79304=ADVANCED_FACE('',(#23874),#243,.F.);
#79305=ADVANCED_FACE('',(#23875),#2385,.F.);
#79306=ADVANCED_FACE('',(#23876),#1973,.F.);
#79307=ADVANCED_FACE('',(#23877,#1725),#19868,.F.);
#79308=ADVANCED_FACE('',(#23878,#1726),#19869,.F.);
#79309=ADVANCED_FACE('',(#23879,#1727),#19870,.T.);
#79310=ADVANCED_FACE('',(#23880),#2386,.F.);
#79311=ADVANCED_FACE('',(#23881),#1974,.F.);
#79312=ADVANCED_FACE('',(#23882,#1728),#19871,.T.);
#79313=ADVANCED_FACE('',(#23883),#2387,.T.);
#79314=ADVANCED_FACE('',(#23884),#244,.F.);
#79315=ADVANCED_FACE('',(#23885),#75302,.T.);
#79316=ADVANCED_FACE('',(#23886),#19872,.T.);
#79317=ADVANCED_FACE('',(#23887),#2388,.T.);
#79335=CLOSED_SHELL('',(#79238,#79239,#79240,#79241,#79242,#79243,#79244,
#79245,#79246,#79247,#79248,#79249,#79250,#79251,#79252,#79253,#79254,#79255,
#79256,#79257,#79258,#79259,#79260,#79261,#79262,#79263,#79264,#79265,#79266,
#79267,#79268,#79269,#79270,#79271,#79272,#79273,#79274,#79275,#79276,#79277,
#79278,#79279,#79280,#79281,#79282,#79283,#79284,#79285,#79286,#79287,#79288,
#79289,#79290,#79291,#79292,#79293,#79294,#79295,#79296,#79297,#79298,#79299,
#79300,#79301,#79302,#79303,#79304,#79305,#79306,#79307,#79308,#79309,#79310,
#79311,#79312,#79313,#79314,#79315,#79316,#79317));
#86059=AXIS2_PLACEMENT_3D('',#212789,#106324,#106325);
#86060=AXIS2_PLACEMENT_3D('',#212790,#106326,#106327);
#86061=AXIS2_PLACEMENT_3D('',#212862,#106330,#106331);
#86062=AXIS2_PLACEMENT_3D('',#212863,#106332,#106333);
#86063=AXIS2_PLACEMENT_3D('',#212959,#106335,#106336);
#86064=AXIS2_PLACEMENT_3D('',#213099,#106338,#106339);
#86065=AXIS2_PLACEMENT_3D('',#213235,#106341,#106342);
#86066=AXIS2_PLACEMENT_3D('',#213378,#106344,#106345);
#86067=AXIS2_PLACEMENT_3D('',#213515,#106347,#106348);
#86068=AXIS2_PLACEMENT_3D('',#213651,#106350,#106351);
#86069=AXIS2_PLACEMENT_3D('',#213787,#106353,#106354);
#86070=AXIS2_PLACEMENT_3D('',#213914,#106356,#106357);
#86071=AXIS2_PLACEMENT_3D('',#213927,#106359,#106360);
#86072=AXIS2_PLACEMENT_3D('',#213928,#106361,#106362);
#86073=AXIS2_PLACEMENT_3D('',#213997,#106364,#106365);
#86074=AXIS2_PLACEMENT_3D('',#214062,#106366,#106367);
#86075=AXIS2_PLACEMENT_3D('',#214203,#106369,#106370);
#86076=AXIS2_PLACEMENT_3D('',#214368,#106372,#106373);
#86077=AXIS2_PLACEMENT_3D('',#214526,#106375,#106376);
#86078=AXIS2_PLACEMENT_3D('',#214693,#106378,#106379);
#86079=AXIS2_PLACEMENT_3D('',#214858,#106381,#106382);
#86080=AXIS2_PLACEMENT_3D('',#215018,#106384,#106385);
#86081=AXIS2_PLACEMENT_3D('',#215021,#106386,#106387);
#86082=AXIS2_PLACEMENT_3D('',#215022,#106388,#106389);
#86083=AXIS2_PLACEMENT_3D('',#215118,#106393,#106394);
#86084=AXIS2_PLACEMENT_3D('',#215174,#106396,#106397);
#86085=AXIS2_PLACEMENT_3D('',#215233,#106398,#106399);
#86086=AXIS2_PLACEMENT_3D('',#215269,#106402,#106403);
#86087=AXIS2_PLACEMENT_3D('',#215411,#106405,#106406);
#86088=AXIS2_PLACEMENT_3D('',#215561,#106408,#106409);
#86089=AXIS2_PLACEMENT_3D('',#215707,#106411,#106412);
#86090=AXIS2_PLACEMENT_3D('',#215735,#106415,#106416);
#86091=AXIS2_PLACEMENT_3D('',#215875,#106418,#106419);
#86092=AXIS2_PLACEMENT_3D('',#216011,#106421,#106422);
#86093=AXIS2_PLACEMENT_3D('',#216149,#106424,#106425);
#86094=AXIS2_PLACEMENT_3D('',#216165,#106427,#106428);
#86095=AXIS2_PLACEMENT_3D('',#216166,#106429,#106430);
#86096=AXIS2_PLACEMENT_3D('',#216246,#106432,#106433);
#86097=AXIS2_PLACEMENT_3D('',#216319,#106434,#106435);
#86098=AXIS2_PLACEMENT_3D('',#216477,#106437,#106438);
#86099=AXIS2_PLACEMENT_3D('',#216635,#106440,#106441);
#86100=AXIS2_PLACEMENT_3D('',#216693,#106444,#106445);
#86101=AXIS2_PLACEMENT_3D('',#216853,#106447,#106448);
#86102=AXIS2_PLACEMENT_3D('',#217013,#106450,#106451);
#86103=AXIS2_PLACEMENT_3D('',#217173,#106453,#106454);
#86104=AXIS2_PLACEMENT_3D('',#217178,#106456,#106457);
#86105=AXIS2_PLACEMENT_3D('',#217251,#106458,#106459);
#86106=AXIS2_PLACEMENT_3D('',#217289,#106460,#106461);
#86107=AXIS2_PLACEMENT_3D('',#217303,#106462,#106463);
#86108=AXIS2_PLACEMENT_3D('',#217304,#106464,#106465);
#86109=AXIS2_PLACEMENT_3D('',#217306,#106466,#106467);
#86110=AXIS2_PLACEMENT_3D('',#217309,#106469,#106470);
#86111=AXIS2_PLACEMENT_3D('',#217310,#106471,#106472);
#86112=AXIS2_PLACEMENT_3D('',#217327,#106473,#106474);
#86113=AXIS2_PLACEMENT_3D('',#217362,#106475,#106476);
#86114=AXIS2_PLACEMENT_3D('',#217395,#106477,#106478);
#86115=AXIS2_PLACEMENT_3D('',#217429,#106481,#106482);
#86116=AXIS2_PLACEMENT_3D('',#217431,#106483,#106484);
#86117=AXIS2_PLACEMENT_3D('',#217560,#106485,#106486);
#86118=AXIS2_PLACEMENT_3D('',#217673,#106487,#106488);
#86119=AXIS2_PLACEMENT_3D('',#218475,#106492,#106493);
#86120=AXIS2_PLACEMENT_3D('',#219142,#106496,#106497);
#86121=AXIS2_PLACEMENT_3D('',#219147,#106499,#106500);
#86122=AXIS2_PLACEMENT_3D('',#219148,#106501,#106502);
#86123=AXIS2_PLACEMENT_3D('',#219149,#106503,#106504);
#86124=AXIS2_PLACEMENT_3D('',#219150,#106505,#106506);
#86125=AXIS2_PLACEMENT_3D('',#219151,#106507,#106508);
#86126=AXIS2_PLACEMENT_3D('',#219153,#106509,#106510);
#86127=AXIS2_PLACEMENT_3D('',#219164,#106511,#106512);
#86128=AXIS2_PLACEMENT_3D('',#220233,#106515,#106516);
#86129=AXIS2_PLACEMENT_3D('',#221041,#106519,#106520);
#86130=AXIS2_PLACEMENT_3D('',#221462,#106522,#106523);
#86131=AXIS2_PLACEMENT_3D('',#221465,#106524,#106525);
#86132=AXIS2_PLACEMENT_3D('',#221468,#106527,#106528);
#86133=AXIS2_PLACEMENT_3D('',#221469,#106529,#106530);
#86134=AXIS2_PLACEMENT_3D('',#221470,#106531,#106532);
#86135=AXIS2_PLACEMENT_3D('',#221473,#106534,#106535);
#86136=AXIS2_PLACEMENT_3D('',#221474,#106536,#106537);
#86137=AXIS2_PLACEMENT_3D('',#221475,#106538,#106539);
#86138=AXIS2_PLACEMENT_3D('',#221476,#106540,#106541);
#86139=AXIS2_PLACEMENT_3D('',#221478,#106542,#106543);
#86140=AXIS2_PLACEMENT_3D('',#221479,#106544,#106545);
#86141=AXIS2_PLACEMENT_3D('',#221482,#106547,#106548);
#86142=AXIS2_PLACEMENT_3D('',#221483,#106549,#106550);
#86143=AXIS2_PLACEMENT_3D('',#221486,#106552,#106553);
#86144=AXIS2_PLACEMENT_3D('',#221487,#106554,#106555);
#86145=AXIS2_PLACEMENT_3D('',#221494,#106556,#106557);
#86146=AXIS2_PLACEMENT_3D('',#221603,#106558,#106559);
#86147=AXIS2_PLACEMENT_3D('',#221615,#106560,#106561);
#86148=AXIS2_PLACEMENT_3D('',#221616,#106562,#106563);
#86149=AXIS2_PLACEMENT_3D('',#221617,#106564,#106565);
#86150=AXIS2_PLACEMENT_3D('',#221619,#106567,#106568);
#106324=DIRECTION('axis',(0.,0.,1.));
#106325=DIRECTION('refdir',(1.,0.,0.));
#106326=DIRECTION('center_axis',(-1.,0.,0.));
#106327=DIRECTION('ref_axis',(0.,-0.924224592736303,-0.381849318686592));
#106328=DIRECTION('',(1.,0.,0.));
#106329=DIRECTION('',(1.,0.,0.));
#106330=DIRECTION('center_axis',(-1.,0.,0.));
#106331=DIRECTION('ref_axis',(0.,0.924224592736302,0.381849318686594));
#106332=DIRECTION('center_axis',(-1.,0.,0.));
#106333=DIRECTION('ref_axis',(0.,0.924224592736302,0.381849318686594));
#106334=DIRECTION('',(-1.,0.,0.));
#106335=DIRECTION('center_axis',(-1.,0.,0.));
#106336=DIRECTION('ref_axis',(0.,-0.924224592736303,-0.381849318686592));
#106337=DIRECTION('',(1.,0.,0.));
#106338=DIRECTION('center_axis',(-1.,0.,0.));
#106339=DIRECTION('ref_axis',(0.,-0.924224592736303,-0.381849318686592));
#106340=DIRECTION('',(1.,0.,0.));
#106341=DIRECTION('center_axis',(-1.,0.,0.));
#106342=DIRECTION('ref_axis',(0.,-0.924224592736303,-0.381849318686592));
#106343=DIRECTION('',(1.,0.,0.));
#106344=DIRECTION('center_axis',(-1.,0.,0.));
#106345=DIRECTION('ref_axis',(0.,-0.924224592736303,-0.381849318686592));
#106346=DIRECTION('',(1.,0.,0.));
#106347=DIRECTION('center_axis',(-1.,0.,0.));
#106348=DIRECTION('ref_axis',(0.,-0.924224592736303,-0.381849318686592));
#106349=DIRECTION('',(1.,0.,0.));
#106350=DIRECTION('center_axis',(-1.,0.,0.));
#106351=DIRECTION('ref_axis',(0.,-0.924224592736303,-0.381849318686592));
#106352=DIRECTION('',(1.,0.,0.));
#106353=DIRECTION('center_axis',(-1.,0.,0.));
#106354=DIRECTION('ref_axis',(0.,-0.924224592736303,-0.381849318686592));
#106355=DIRECTION('',(1.,0.,0.));
#106356=DIRECTION('center_axis',(-1.,0.,0.));
#106357=DIRECTION('ref_axis',(0.,-0.924224592736303,-0.381849318686593));
#106358=DIRECTION('',(1.,0.,0.));
#106359=DIRECTION('center_axis',(1.,0.,0.));
#106360=DIRECTION('ref_axis',(0.,0.999244149014678,-0.0388732640761329));
#106361=DIRECTION('center_axis',(-1.,0.,0.));
#106362=DIRECTION('ref_axis',(0.,-0.924224592736303,-0.381849318686593));
#106363=DIRECTION('',(1.,0.,0.));
#106364=DIRECTION('center_axis',(1.,0.,0.));
#106365=DIRECTION('ref_axis',(0.,0.999244149014678,-0.0388732640761329));
#106366=DIRECTION('center_axis',(-1.,0.,0.));
#106367=DIRECTION('ref_axis',(0.,-0.924224592736303,-0.381849318686593));
#106368=DIRECTION('',(1.,0.,0.));
#106369=DIRECTION('center_axis',(-1.,0.,0.));
#106370=DIRECTION('ref_axis',(0.,-0.924224592736303,-0.381849318686593));
#106371=DIRECTION('',(1.,0.,0.));
#106372=DIRECTION('center_axis',(-1.,0.,0.));
#106373=DIRECTION('ref_axis',(0.,-0.924224592736303,-0.381849318686593));
#106374=DIRECTION('',(1.,0.,0.));
#106375=DIRECTION('center_axis',(-1.,0.,0.));
#106376=DIRECTION('ref_axis',(0.,-0.924224592736303,-0.381849318686593));
#106377=DIRECTION('',(1.,0.,0.));
#106378=DIRECTION('center_axis',(-1.,0.,0.));
#106379=DIRECTION('ref_axis',(0.,-0.924224592736303,-0.381849318686593));
#106380=DIRECTION('',(1.,0.,0.));
#106381=DIRECTION('center_axis',(-1.,0.,0.));
#106382=DIRECTION('ref_axis',(0.,-0.924224592736303,-0.381849318686593));
#106383=DIRECTION('',(1.,0.,0.));
#106384=DIRECTION('center_axis',(-1.,0.,0.));
#106385=DIRECTION('ref_axis',(0.,-0.924224592736303,-0.381849318686593));
#106386=DIRECTION('center_axis',(1.,0.,0.));
#106387=DIRECTION('ref_axis',(0.,-0.924224592736303,-0.381849318686593));
#106388=DIRECTION('center_axis',(1.,0.,0.));
#106389=DIRECTION('ref_axis',(0.,-0.924224592736303,-0.381849318686593));
#106390=DIRECTION('',(1.,0.,0.));
#106391=DIRECTION('',(-1.,0.,0.));
#106392=DIRECTION('',(1.,0.,0.));
#106393=DIRECTION('center_axis',(-1.,7.59792509022099E-17,3.13913148593356E-17));
#106394=DIRECTION('ref_axis',(-8.2208644413218E-17,-0.924224592736303,-0.381849318686593));
#106395=DIRECTION('',(0.70710665146941,-0.653525596750962,-0.270008292167144));
#106396=DIRECTION('center_axis',(1.,0.,0.));
#106397=DIRECTION('ref_axis',(0.,-0.050910732461195,0.99870320782516));
#106398=DIRECTION('center_axis',(1.,0.,0.));
#106399=DIRECTION('ref_axis',(0.,0.924224592736303,0.381849318686593));
#106400=DIRECTION('',(-1.,0.,0.));
#106401=DIRECTION('',(0.999999999998702,-7.34588841051575E-7,-1.43405422420294E-6));
#106402=DIRECTION('center_axis',(1.,0.,0.));
#106403=DIRECTION('ref_axis',(0.,0.924224592736303,0.381849318686593));
#106404=DIRECTION('',(-1.,0.,0.));
#106405=DIRECTION('center_axis',(1.,0.,0.));
#106406=DIRECTION('ref_axis',(0.,0.924224592736303,0.381849318686593));
#106407=DIRECTION('',(-1.,0.,0.));
#106408=DIRECTION('center_axis',(1.,0.,0.));
#106409=DIRECTION('ref_axis',(0.,0.924224592736303,0.381849318686593));
#106410=DIRECTION('',(-1.,0.,0.));
#106411=DIRECTION('center_axis',(1.,0.,0.));
#106412=DIRECTION('ref_axis',(0.,0.924224592736303,0.381849318686592));
#106413=DIRECTION('',(-1.,0.,0.));
#106414=DIRECTION('',(0.999999999947399,4.18358171207589E-7,1.02482904113352E-5));
#106415=DIRECTION('center_axis',(1.,0.,0.));
#106416=DIRECTION('ref_axis',(0.,0.924224592736303,0.381849318686592));
#106417=DIRECTION('',(-1.,0.,0.));
#106418=DIRECTION('center_axis',(1.,0.,0.));
#106419=DIRECTION('ref_axis',(0.,0.924224592736303,0.381849318686592));
#106420=DIRECTION('',(-1.,0.,0.));
#106421=DIRECTION('center_axis',(1.,0.,0.));
#106422=DIRECTION('ref_axis',(0.,0.924224592736303,0.381849318686592));
#106423=DIRECTION('',(-1.,0.,0.));
#106424=DIRECTION('center_axis',(1.,0.,0.));
#106425=DIRECTION('ref_axis',(0.,0.924224592736303,0.381849318686592));
#106426=DIRECTION('',(-1.,0.,0.));
#106427=DIRECTION('center_axis',(-1.,0.,0.));
#106428=DIRECTION('ref_axis',(0.,0.924224592736303,0.381849318686592));
#106429=DIRECTION('center_axis',(1.,1.82571941840305E-14,2.33421417227065E-14));
#106430=DIRECTION('ref_axis',(-2.57869287727445E-14,0.924224592736303,0.381849318686593));
#106431=DIRECTION('',(-1.,-1.82571941840305E-14,-2.33421417227065E-14));
#106432=DIRECTION('center_axis',(-2.33885900086631E-13,-0.695858933998045,
0.71817849033169));
#106433=DIRECTION('ref_axis',(-0.0305944370088395,0.717842297079444,0.695533188962123));
#106434=DIRECTION('center_axis',(1.,1.82571941840305E-14,2.33421417227065E-14));
#106435=DIRECTION('ref_axis',(-2.57869287727445E-14,0.924224592736303,0.381849318686593));
#106436=DIRECTION('',(-1.,-1.82571941840305E-14,-2.33421417227065E-14));
#106437=DIRECTION('center_axis',(1.,1.82571941840305E-14,2.33421417227065E-14));
#106438=DIRECTION('ref_axis',(-2.57869287727445E-14,0.924224592736303,0.381849318686593));
#106439=DIRECTION('',(-1.,-1.82571941840305E-14,-2.33421417227065E-14));
#106440=DIRECTION('center_axis',(1.,0.,0.));
#106441=DIRECTION('ref_axis',(0.,0.924224592736303,0.381849318686593));
#106442=DIRECTION('',(-1.,0.,0.));
#106443=DIRECTION('',(-0.999999999940701,1.01456975879523E-5,3.95770553001597E-6));
#106444=DIRECTION('center_axis',(1.,0.,0.));
#106445=DIRECTION('ref_axis',(0.,0.924224592736303,0.381849318686593));
#106446=DIRECTION('',(-1.,0.,0.));
#106447=DIRECTION('center_axis',(1.,0.,0.));
#106448=DIRECTION('ref_axis',(0.,0.924224592736303,0.381849318686593));
#106449=DIRECTION('',(-1.,0.,0.));
#106450=DIRECTION('center_axis',(1.,0.,0.));
#106451=DIRECTION('ref_axis',(0.,0.924224592736303,0.381849318686593));
#106452=DIRECTION('',(-1.,0.,0.));
#106453=DIRECTION('center_axis',(1.,-2.54046812768854E-17,-1.04961070212471E-17));
#106454=DIRECTION('ref_axis',(2.74875625216498E-17,0.924224592736303,0.381849318686593));
#106455=DIRECTION('',(-0.707106662296841,0.653525586743986,0.270008288032699));
#106456=DIRECTION('center_axis',(-1.,0.,0.));
#106457=DIRECTION('ref_axis',(0.,-0.316348137924587,-0.948643165595814));
#106458=DIRECTION('center_axis',(-1.,0.,0.));
#106459=DIRECTION('ref_axis',(0.,-0.916443657855559,0.400163743955299));
#106460=DIRECTION('center_axis',(1.,-2.54046812768854E-17,-1.04961070212471E-17));
#106461=DIRECTION('ref_axis',(2.74875625216498E-17,0.924224592736303,0.381849318686593));
#106462=DIRECTION('center_axis',(-1.,0.,0.));
#106463=DIRECTION('ref_axis',(0.,-0.316348137924587,-0.948643165595814));
#106464=DIRECTION('center_axis',(0.965925826289076,0.239206926552251,0.0988298760355017));
#106465=DIRECTION('ref_axis',(-0.258819045102494,0.892732403415498,0.368838118670266));
#106466=DIRECTION('center_axis',(1.,2.30623636574202E-15,5.83716380003748E-15));
#106467=DIRECTION('ref_axis',(-4.36039738599217E-15,0.924224592735944,0.381849318687461));
#106468=DIRECTION('',(0.965925826289076,0.239206926552251,0.0988298760355017));
#106469=DIRECTION('center_axis',(1.,1.15311818287128E-15,2.91858190001905E-15));
#106470=DIRECTION('ref_axis',(-2.18019869299788E-15,0.924224592735703,0.381849318688045));
#106471=DIRECTION('center_axis',(1.,0.,0.));
#106472=DIRECTION('ref_axis',(0.,0.924224592736303,0.381849318686593));
#106473=DIRECTION('center_axis',(1.,1.82571941840305E-14,2.33421417227065E-14));
#106474=DIRECTION('ref_axis',(-2.57869287727445E-14,0.924224592736303,0.381849318686593));
#106475=DIRECTION('center_axis',(0.,-0.393059646019601,-0.919512976890999));
#106476=DIRECTION('ref_axis',(-0.0130647305360937,-0.919434499001734,0.39302609946599));
#106477=DIRECTION('center_axis',(0.965925826289076,0.239206926552251,0.0988298760355016));
#106478=DIRECTION('ref_axis',(-0.258819045102493,0.892732403415498,0.368838118670267));
#106479=DIRECTION('',(0.965925826289076,0.239206926552251,0.0988298760355015));
#106480=DIRECTION('',(0.965925826289076,0.239206926552251,0.0988298760355015));
#106481=DIRECTION('center_axis',(1.,0.,0.));
#106482=DIRECTION('ref_axis',(0.,0.924224592736303,0.381849318686592));
#106483=DIRECTION('center_axis',(-1.,0.,0.));
#106484=DIRECTION('ref_axis',(0.,0.924224592736303,0.381849318686592));
#106485=DIRECTION('center_axis',(1.,0.,0.));
#106486=DIRECTION('ref_axis',(0.,0.924224592736303,0.381849318686592));
#106487=DIRECTION('center_axis',(1.,0.,0.));
#106488=DIRECTION('ref_axis',(0.,0.924224592736303,0.381849318686593));
#106489=DIRECTION('',(1.,0.,0.));
#106490=DIRECTION('',(0.461762345735437,0.88626469878453,-0.0361997202927509));
#106491=DIRECTION('',(0.46176244446361,0.789444381060382,-0.404416881565523));
#106492=DIRECTION('center_axis',(0.,0.888370688458611,-0.459126910437161));
#106493=DIRECTION('ref_axis',(-1.,0.,0.));
#106494=DIRECTION('',(0.461762450482974,-0.789465505391398,0.404375636161556));
#106495=DIRECTION('',(0.461762365531073,-0.886266296190209,0.0361603376150781));
#106496=DIRECTION('center_axis',(0.,0.381849318686593,-0.924224592736303));
#106497=DIRECTION('ref_axis',(-1.,0.,0.));
#106498=DIRECTION('',(0.965925826289076,0.239206926552251,0.0988298760355015));
#106499=DIRECTION('center_axis',(-3.19816689560775E-17,0.381849318686593,
-0.924224592736303));
#106500=DIRECTION('ref_axis',(0.995486289304339,0.0877139672710818,0.0362395881964125));
#106501=DIRECTION('center_axis',(-3.19816689560775E-17,0.381849318686593,
-0.924224592736303));
#106502=DIRECTION('ref_axis',(0.995486289304339,0.0877139672710818,0.0362395881964125));
#106503=DIRECTION('center_axis',(-2.85555636349464E-16,0.381849318686593,
-0.924224592736303));
#106504=DIRECTION('ref_axis',(-0.989158808077185,-0.135722160860674,-0.0560744813139883));
#106505=DIRECTION('center_axis',(1.,0.,0.));
#106506=DIRECTION('ref_axis',(0.,-0.381849318686593,0.924224592736303));
#106507=DIRECTION('center_axis',(0.,0.924224592736303,0.381849318686593));
#106508=DIRECTION('ref_axis',(0.,0.381849318686593,-0.924224592736303));
#106509=DIRECTION('center_axis',(-8.53563043435897E-18,-0.381849318686593,
0.924224592736303));
#106510=DIRECTION('ref_axis',(-0.999927597212881,-0.0111214726821253,-0.00459490777440583));
#106511=DIRECTION('center_axis',(-1.,7.59792509022099E-17,3.13913148593356E-17));
#106512=DIRECTION('ref_axis',(-8.2208644413218E-17,-0.924224592736303,-0.381849318686593));
#106513=DIRECTION('',(-1.,0.,0.));
#106514=DIRECTION('',(-0.461755073126971,0.63699274562483,0.617270195670297));
#106515=DIRECTION('center_axis',(0.,-0.0569081128227818,-0.998379420208044));
#106516=DIRECTION('ref_axis',(0.,-0.998379420208044,0.0569081128227818));
#106517=DIRECTION('',(-0.461755065119693,-0.636985304497731,-0.617277880447891));
#106518=DIRECTION('',(-0.461755171832,0.815781579343933,-0.348256480326666));
#106519=DIRECTION('center_axis',(-1.,0.,0.));
#106520=DIRECTION('ref_axis',(0.,-0.924224592736303,-0.381849318686593));
#106521=DIRECTION('',(-0.461755171705888,-0.815781579302177,0.348256480591692));
#106522=DIRECTION('center_axis',(-1.,0.,0.));
#106523=DIRECTION('ref_axis',(0.,-0.924224592736303,-0.381849318686592));
#106524=DIRECTION('center_axis',(-1.,0.,0.));
#106525=DIRECTION('ref_axis',(0.,-0.924224592736303,-0.381849318686592));
#106526=DIRECTION('',(-1.,0.,0.));
#106527=DIRECTION('center_axis',(-1.,0.,0.));
#106528=DIRECTION('ref_axis',(0.,-0.924224592736303,-0.381849318686592));
#106529=DIRECTION('center_axis',(-1.,0.,0.));
#106530=DIRECTION('ref_axis',(0.,-0.924224592736303,-0.381849318686592));
#106531=DIRECTION('center_axis',(1.,3.80693114761575E-17,1.57285802220435E-17));
#106532=DIRECTION('ref_axis',(-4.11905415364978E-17,0.924224592736303,0.381849318686593));
#106533=DIRECTION('',(0.707106580681804,-0.653525662174577,-0.270008319197331));
#106534=DIRECTION('center_axis',(-1.,0.,0.));
#106535=DIRECTION('ref_axis',(-4.11905415364978E-17,0.924224592736303,0.381849318686593));
#106536=DIRECTION('center_axis',(-1.,0.,0.));
#106537=DIRECTION('ref_axis',(0.,0.,1.));
#106538=DIRECTION('center_axis',(-1.,0.,0.));
#106539=DIRECTION('ref_axis',(0.,0.,1.));
#106540=DIRECTION('center_axis',(-1.,0.,0.));
#106541=DIRECTION('ref_axis',(0.,0.,1.));
#106542=DIRECTION('center_axis',(-1.,0.,0.));
#106543=DIRECTION('ref_axis',(0.,-0.924224592736303,-0.381849318686592));
#106544=DIRECTION('center_axis',(-1.,0.,0.));
#106545=DIRECTION('ref_axis',(0.,-0.924224592736303,-0.381849318686592));
#106546=DIRECTION('',(-1.,0.,0.));
#106547=DIRECTION('center_axis',(1.,0.,0.));
#106548=DIRECTION('ref_axis',(0.,0.924224592736303,0.381849318686592));
#106549=DIRECTION('center_axis',(-1.,2.54488112923718E-17,1.05143396202058E-17));
#106550=DIRECTION('ref_axis',(-2.75353106727304E-17,-0.924224592736303,
-0.381849318686592));
#106551=DIRECTION('',(-0.7071070062405,0.653525268862752,0.270008156698027));
#106552=DIRECTION('center_axis',(1.,0.,0.));
#106553=DIRECTION('ref_axis',(0.,-0.924224592736303,-0.381849318686592));
#106554=DIRECTION('center_axis',(-1.,0.,0.));
#106555=DIRECTION('ref_axis',(0.,0.,1.));
#106556=DIRECTION('center_axis',(-1.,0.,0.));
#106557=DIRECTION('ref_axis',(0.,-0.924224592736303,-0.381849318686592));
#106558=DIRECTION('center_axis',(1.,0.,0.));
#106559=DIRECTION('ref_axis',(0.,-0.381849318686592,0.924224592736303));
#106560=DIRECTION('center_axis',(7.6756005494586E-17,-0.381849318686593,
0.924224592736303));
#106561=DIRECTION('ref_axis',(0.99903497276754,-0.0405935937462799,-0.0167715036332949));
#106562=DIRECTION('center_axis',(0.,0.924224592736303,0.381849318686592));
#106563=DIRECTION('ref_axis',(0.,0.381849318686592,-0.924224592736303));
#106564=DIRECTION('center_axis',(0.,-0.381849318686593,0.924224592736303));
#106565=DIRECTION('ref_axis',(-1.,0.,0.));
#106566=DIRECTION('',(0.965925826289076,0.239206926552251,0.0988298760355015));
#106567=DIRECTION('center_axis',(0.965925826289076,0.239206926552251,0.0988298760355016));
#106568=DIRECTION('ref_axis',(0.258819045102493,-0.8927324034155,-0.368838118670263));
#212789=CARTESIAN_POINT('',(0.,0.,0.));
#212790=CARTESIAN_POINT('Origin',(-45.8894114130409,66.6819786653733,69.5522455184007));
#212791=CARTESIAN_POINT('',(-50.2096235848679,76.1552807409204,73.4662010349383));
#212792=CARTESIAN_POINT('',(-49.8038356726598,76.1552807409204,73.4662010349383));
#212793=CARTESIAN_POINT('',(-45.8894114130409,76.1552807409204,73.4662010349383));
#212794=CARTESIAN_POINT('',(-48.3958698180353,76.1552807409204,73.4662010349383));
#212795=CARTESIAN_POINT('Ctrl Pts',(-48.3958698180353,76.1552807409204,
73.4662010349383));
#212796=CARTESIAN_POINT('Ctrl Pts',(-48.4037687557346,76.2613287309383,
73.20952345143));
#212797=CARTESIAN_POINT('Ctrl Pts',(-48.4116574019032,76.356944970118,72.9485353906266));
#212798=CARTESIAN_POINT('Ctrl Pts',(-48.4339259826903,76.5990765131584,
72.1939192103763));
#212799=CARTESIAN_POINT('Ctrl Pts',(-48.4481644740065,76.7191699956859,
71.6928212361976));
#212800=CARTESIAN_POINT('Ctrl Pts',(-48.4804668304725,76.9027546290379,
70.5549183741424));
#212801=CARTESIAN_POINT('Ctrl Pts',(-48.4985952978972,76.945342113167,69.9168971044106));
#212802=CARTESIAN_POINT('Ctrl Pts',(-48.5346717449819,76.9115063939614,
68.6477299765805));
#212803=CARTESIAN_POINT('Ctrl Pts',(-48.5522008346175,76.8363585270069,
68.0192878554966));
#212804=CARTESIAN_POINT('Ctrl Pts',(-48.5881874645723,76.5661488628059,
66.7600297743452));
#212805=CARTESIAN_POINT('Ctrl Pts',(-48.606734672987,76.3671254737777,66.1330050342624));
#212806=CARTESIAN_POINT('Ctrl Pts',(-48.6573395820654,75.6689354911155,
64.4968214357699));
#212807=CARTESIAN_POINT('Ctrl Pts',(-48.6880625247023,75.0616977825945,
63.5436660846541));
#212808=CARTESIAN_POINT('Ctrl Pts',(-48.739015526114,73.8608521574925,62.204934139578));
#212809=CARTESIAN_POINT('Ctrl Pts',(-48.7583175195139,73.3609449818661,
61.7477188811338));
#212810=CARTESIAN_POINT('Ctrl Pts',(-48.796059042918,72.2791716184435,60.9389186280048));
#212811=CARTESIAN_POINT('Ctrl Pts',(-48.8147908553493,71.7000674552926,
60.5891683794301));
#212812=CARTESIAN_POINT('Ctrl Pts',(-48.8432065931581,70.7940124609989,
60.1574724749579));
#212813=CARTESIAN_POINT('Ctrl Pts',(-48.852566274679,70.4905886251576,60.0304247050254));
#212814=CARTESIAN_POINT('Ctrl Pts',(-48.8912166403082,69.2128383647712,
59.5662775268822));
#212815=CARTESIAN_POINT('Ctrl Pts',(-48.919427938587,68.1965338099358,59.3624988825998));
#212816=CARTESIAN_POINT('Ctrl Pts',(-48.9579250010423,66.8377107869516,
59.2981281139376));
#212817=CARTESIAN_POINT('Ctrl Pts',(-48.9673076041839,66.5078590897387,
59.2984239158938));
#212818=CARTESIAN_POINT('Ctrl Pts',(-49.0066694303419,65.1253287082858,
59.3664024584995));
#212819=CARTESIAN_POINT('Ctrl Pts',(-49.0355301697569,64.0863348943344,
59.5804252703959));
#212820=CARTESIAN_POINT('Ctrl Pts',(-49.0821868423022,62.5422577967489,
60.1566346720196));
#212821=CARTESIAN_POINT('Ctrl Pts',(-49.0991802722636,62.0052469917899,
60.4120606482223));
#212822=CARTESIAN_POINT('Ctrl Pts',(-49.13012233562,61.0548081345769,60.9699354003627));
#212823=CARTESIAN_POINT('Ctrl Pts',(-49.1441985481586,60.6360151426799,
61.2596328958899));
#212824=CARTESIAN_POINT('Ctrl Pts',(-49.1763003526447,59.745219303344,61.9793191873202));
#212825=CARTESIAN_POINT('Ctrl Pts',(-49.1943953082071,59.2883409062802,
62.4246968243526));
#212826=CARTESIAN_POINT('Ctrl Pts',(-49.2304152812813,58.4667243851996,
63.3902298965006));
#212827=CARTESIAN_POINT('Ctrl Pts',(-49.2479248385016,58.1029727075256,
63.9076463723527));
#212828=CARTESIAN_POINT('Ctrl Pts',(-49.2838818017038,57.46313467177,65.0239820842643));
#212829=CARTESIAN_POINT('Ctrl Pts',(-49.3024121891235,57.1924629443741,
65.6226996657565));
#212830=CARTESIAN_POINT('Ctrl Pts',(-49.3595038007633,56.5445272508622,
67.5222242852832));
#212831=CARTESIAN_POINT('Ctrl Pts',(-49.3964227051368,56.3654717641162,
68.8750548908138));
#212832=CARTESIAN_POINT('Ctrl Pts',(-49.4733091228004,56.5424912469824,
71.5719324914748));
#212833=CARTESIAN_POINT('Ctrl Pts',(-49.510221663426,56.896749352501,72.8895546193486));
#212834=CARTESIAN_POINT('Ctrl Pts',(-49.574895475561,57.9055700503805,74.9269751209315));
#212835=CARTESIAN_POINT('Ctrl Pts',(-49.6003951472506,58.4244902634698,
75.6944736322653));
#212836=CARTESIAN_POINT('Ctrl Pts',(-49.6510179775926,59.6256474344797,
77.0386154294206));
#212837=CARTESIAN_POINT('Ctrl Pts',(-49.6762791927835,60.2943989035603,
77.6167589378013));
#212838=CARTESIAN_POINT('Ctrl Pts',(-49.7143859716436,61.4303856241312,
78.3678616716475));
#212839=CARTESIAN_POINT('Ctrl Pts',(-49.7277380828874,61.8502202856744,
78.6047827107537));
#212840=CARTESIAN_POINT('Ctrl Pts',(-49.7606212093148,62.9083788763079,
79.1072676512745));
#212841=CARTESIAN_POINT('Ctrl Pts',(-49.7803096542754,63.5598991735905,
79.3395385951356));
#212842=CARTESIAN_POINT('Ctrl Pts',(-49.809309783962,64.5543396785134,79.5845625527446));
#212843=CARTESIAN_POINT('Ctrl Pts',(-49.81865052876,64.8826126321066,79.6486070098387));
#212844=CARTESIAN_POINT('Ctrl Pts',(-49.8457240773373,65.8432715171764,
79.7876783315077));
#212845=CARTESIAN_POINT('Ctrl Pts',(-49.8634779845266,66.4802337956011,
79.8200011829438));
#212846=CARTESIAN_POINT('Ctrl Pts',(-49.8956682408361,67.6142406695973,
79.7719330244282));
#212847=CARTESIAN_POINT('Ctrl Pts',(-49.9099239632596,68.1102123514475,
79.7144930808446));
#212848=CARTESIAN_POINT('Ctrl Pts',(-49.9387558076608,69.116613980445,79.5227818061357));
#212849=CARTESIAN_POINT('Ctrl Pts',(-49.953298889289,69.6248619038611,79.3847674347013));
#212850=CARTESIAN_POINT('Ctrl Pts',(-49.9859711912086,70.7235642242247,
78.9935480757809));
#212851=CARTESIAN_POINT('Ctrl Pts',(-50.0041557488555,71.3053952383275,
78.7226660460105));
#212852=CARTESIAN_POINT('Ctrl Pts',(-50.0403294878874,72.4039618302109,
78.0799256841089));
#212853=CARTESIAN_POINT('Ctrl Pts',(-50.0578945679698,72.9190700521586,
77.7107451119027));
#212854=CARTESIAN_POINT('Ctrl Pts',(-50.0939331145991,73.8937406757216,
76.8656229923043));
#212855=CARTESIAN_POINT('Ctrl Pts',(-50.112507719548,74.3479961766235,76.3879723902262));
#212856=CARTESIAN_POINT('Ctrl Pts',(-50.1577532611111,75.3283343011174,
75.1355452762459));
#212857=CARTESIAN_POINT('Ctrl Pts',(-50.1834334662563,75.799782406457,74.3266459468684));
#212858=CARTESIAN_POINT('Ctrl Pts',(-50.2096235848679,76.1552807409204,
73.4662010349383));
#212859=CARTESIAN_POINT('',(-47.5675364832709,76.1552807409204,73.4662010349383));
#212860=CARTESIAN_POINT('',(-45.8894114130409,76.1552807409204,73.4662010349383));
#212861=CARTESIAN_POINT('',(-47.5675364832709,70.5959341819109,60.0789434428536));
#212862=CARTESIAN_POINT('Origin',(-47.5675364832709,66.6819786653733,69.5522455184007));
#212863=CARTESIAN_POINT('Origin',(-47.5675364832709,66.6819786653733,69.5522455184007));
#212864=CARTESIAN_POINT('',(-47.8635970591063,60.3603339176624,77.6206672715226));
#212865=CARTESIAN_POINT('Ctrl Pts',(-47.8635486253615,60.3604524711489,
77.6207526030933));
#212866=CARTESIAN_POINT('Ctrl Pts',(-47.8770447229994,60.7414549300527,
77.9192609886897));
#212867=CARTESIAN_POINT('Ctrl Pts',(-47.8905699687029,61.1431211104073,
78.1904064651098));
#212868=CARTESIAN_POINT('Ctrl Pts',(-47.9176346715792,61.9720633411651,
78.6683172933885));
#212869=CARTESIAN_POINT('Ctrl Pts',(-47.9311325378684,62.3975386486738,
78.8758519992523));
#212870=CARTESIAN_POINT('Ctrl Pts',(-47.9711994802859,63.7080824833602,
79.4063805704902));
#212871=CARTESIAN_POINT('Ctrl Pts',(-47.9969646798076,64.6248316482197,
79.6376897355961));
#212872=CARTESIAN_POINT('Ctrl Pts',(-48.0398256239384,66.1291426136006,
79.8033176844058));
#212873=CARTESIAN_POINT('Ctrl Pts',(-48.0562070950184,66.7023248501976,
79.818194081424));
#212874=CARTESIAN_POINT('Ctrl Pts',(-48.0866516956205,67.7844183957181,
79.7556167899161));
#212875=CARTESIAN_POINT('Ctrl Pts',(-48.1008081906234,68.2921655831365,
79.687898482524));
#212876=CARTESIAN_POINT('Ctrl Pts',(-48.1330139191397,69.416612921757,79.4512727059462));
#212877=CARTESIAN_POINT('Ctrl Pts',(-48.1511303476015,70.0268823608628,
79.2620636919761));
#212878=CARTESIAN_POINT('Ctrl Pts',(-48.1871871027352,71.1986750551804,
78.7750785443067));
#212879=CARTESIAN_POINT('Ctrl Pts',(-48.2047095997858,71.7581107735901,
78.4793996937978));
#212880=CARTESIAN_POINT('Ctrl Pts',(-48.2406862556106,72.836087400015,77.7753770145317));
#212881=CARTESIAN_POINT('Ctrl Pts',(-48.2592278354088,73.3496821753642,
77.3647138069101));
#212882=CARTESIAN_POINT('Ctrl Pts',(-48.309762124485,74.6244967766751,76.1275155310904));
#212883=CARTESIAN_POINT('Ctrl Pts',(-48.340424579748,75.295158013161,75.2206601665416));
#212884=CARTESIAN_POINT('Ctrl Pts',(-48.380049771524,75.9325315626513,73.9757254447151));
#212885=CARTESIAN_POINT('Ctrl Pts',(-48.3879633739574,76.0491319732533,
73.7231225397456));
#212886=CARTESIAN_POINT('Ctrl Pts',(-48.3958698180353,76.1552807409204,
73.4662010349383));
#212887=CARTESIAN_POINT('',(-47.8257920924624,57.2086760965966,65.6382911956718));
#212888=CARTESIAN_POINT('Ctrl Pts',(-47.8635940884285,60.3587924756686,
77.6194517516841));
#212889=CARTESIAN_POINT('Ctrl Pts',(-47.8609618681876,59.70088034951,77.1037712608345));
#212890=CARTESIAN_POINT('Ctrl Pts',(-47.8579335141401,59.1085127669503,
76.5095387599098));
#212891=CARTESIAN_POINT('Ctrl Pts',(-47.8536397962645,58.0877004162917,
75.1986881766103));
#212892=CARTESIAN_POINT('Ctrl Pts',(-47.852298616386,57.6610466594423,74.4885092324322));
#212893=CARTESIAN_POINT('Ctrl Pts',(-47.8482467829846,57.0964955300793,
73.2254447666302));
#212894=CARTESIAN_POINT('Ctrl Pts',(-47.8461648680152,56.9107710683298,
72.6982574235018));
#212895=CARTESIAN_POINT('Ctrl Pts',(-47.840752948818,56.4876427420712,71.0889018852209));
#212896=CARTESIAN_POINT('Ctrl Pts',(-47.838841880717,56.3813930332953,69.9807652008249));
#212897=CARTESIAN_POINT('Ctrl Pts',(-47.8332362516958,56.5277260695749,
67.7636920917063));
#212898=CARTESIAN_POINT('Ctrl Pts',(-47.828574338379,56.7825592211427,66.6696609455421));
#212899=CARTESIAN_POINT('Ctrl Pts',(-47.8257920924624,57.2086760965966,
65.6382911956718));
#212900=CARTESIAN_POINT('',(-47.8068141272352,61.9759278335054,60.4464459619263));
#212901=CARTESIAN_POINT('Ctrl Pts',(-47.8257920924624,57.2086760965966,
65.6382911956718));
#212902=CARTESIAN_POINT('Ctrl Pts',(-47.8243052474299,57.4363949174851,
65.0871224509692));
#212903=CARTESIAN_POINT('Ctrl Pts',(-47.8231856641482,57.7117738155594,
64.5568916645672));
#212904=CARTESIAN_POINT('Ctrl Pts',(-47.8203484488529,58.3555242944295,
63.5441620336238));
#212905=CARTESIAN_POINT('Ctrl Pts',(-47.8182709902653,58.7237180922336,
63.0643356310678));
#212906=CARTESIAN_POINT('Ctrl Pts',(-47.8141911238361,59.5401196520457,
62.1752216331245));
#212907=CARTESIAN_POINT('Ctrl Pts',(-47.8123348538898,59.9867042257069,
61.7676494127296));
#212908=CARTESIAN_POINT('Ctrl Pts',(-47.8093723566015,60.9409141176522,
61.0399854921903));
#212909=CARTESIAN_POINT('Ctrl Pts',(-47.8082478401419,61.4459602057308,
60.7203433366149));
#212910=CARTESIAN_POINT('Ctrl Pts',(-47.8068141268167,61.9759278333883,
60.446445961702));
#212911=CARTESIAN_POINT('',(-48.1735608262671,61.9759278335638,60.4464459619211));
#212912=CARTESIAN_POINT('',(-47.8068954859909,61.9759278333895,60.4464459616985));
#212913=CARTESIAN_POINT('',(-48.5599506281375,57.2086985431952,65.6382368665521));
#212914=CARTESIAN_POINT('Ctrl Pts',(-48.1735608267226,61.9759278334593,
60.4464459616654));
#212915=CARTESIAN_POINT('Ctrl Pts',(-48.2057390453445,61.4459676212693,
60.720339504118));
#212916=CARTESIAN_POINT('Ctrl Pts',(-48.2381635012091,60.9409268906735,
61.0399772116217));
#212917=CARTESIAN_POINT('Ctrl Pts',(-48.3027869041061,59.9867342135912,
61.7676250678449));
#212918=CARTESIAN_POINT('Ctrl Pts',(-48.3348415809302,59.5401513749368,
62.1751899810842));
#212919=CARTESIAN_POINT('Ctrl Pts',(-48.3987590450242,58.7236761239669,
63.0643784397394));
#212920=CARTESIAN_POINT('Ctrl Pts',(-48.4306399072594,58.3554424481484,
63.5442696368759));
#212921=CARTESIAN_POINT('Ctrl Pts',(-48.4954405792784,57.7117295276132,
64.5569822372555));
#212922=CARTESIAN_POINT('Ctrl Pts',(-48.5278559888906,57.4363874184328,
65.0871495574296));
#212923=CARTESIAN_POINT('Ctrl Pts',(-48.5599506281375,57.2086985431952,
65.6382368665521));
#212924=CARTESIAN_POINT('',(-49.2715796128967,60.3604384525828,77.6207039925157));
#212925=CARTESIAN_POINT('Ctrl Pts',(-48.5599506281375,57.2086985431952,
65.6382368665521));
#212926=CARTESIAN_POINT('Ctrl Pts',(-48.6200116739718,56.7826076977302,
66.6695268548047));
#212927=CARTESIAN_POINT('Ctrl Pts',(-48.6777501611375,56.5277719080271,
67.7634817707358));
#212928=CARTESIAN_POINT('Ctrl Pts',(-48.7973670931621,56.3813781413118,
69.9805110412448));
#212929=CARTESIAN_POINT('Ctrl Pts',(-48.8573471180376,56.4876125809909,
71.0887662129764));
#212930=CARTESIAN_POINT('Ctrl Pts',(-48.945646231306,56.9107583214791,72.6982195125108));
#212931=CARTESIAN_POINT('Ctrl Pts',(-48.9749440674501,57.0964827935491,
73.225411282841));
#212932=CARTESIAN_POINT('Ctrl Pts',(-49.0488658367832,57.6610336028653,
74.4884874003299));
#212933=CARTESIAN_POINT('Ctrl Pts',(-49.0938910637438,58.0876892930809,
75.1986713149217));
#212934=CARTESIAN_POINT('Ctrl Pts',(-49.1831733484294,59.1084952031266,
76.5095188164509));
#212935=CARTESIAN_POINT('Ctrl Pts',(-49.2270302012072,59.7008638570257,
77.1037580932682));
#212936=CARTESIAN_POINT('Ctrl Pts',(-49.2714848090302,60.3587906487603,
77.6194503197282));
#212937=CARTESIAN_POINT('Ctrl Pts',(-49.8038356726598,76.1552807409204,
73.4662010349383));
#212938=CARTESIAN_POINT('Ctrl Pts',(-49.7955673541574,76.0420944588995,
73.7401560750152));
#212939=CARTESIAN_POINT('Ctrl Pts',(-49.7873093511155,75.9170383668382,
74.0091679731417));
#212940=CARTESIAN_POINT('Ctrl Pts',(-49.760094216857,75.4696311167998,74.8715676798369));
#212941=CARTESIAN_POINT('Ctrl Pts',(-49.7409083974812,75.1004089147373,
75.4385040151837));
#212942=CARTESIAN_POINT('Ctrl Pts',(-49.702549221666,74.255343090125,76.4922298043504));
#212943=CARTESIAN_POINT('Ctrl Pts',(-49.683863456909,73.7814231596948,76.9763360851991));
#212944=CARTESIAN_POINT('Ctrl Pts',(-49.6332831714931,72.3961975764906,
78.1365052775401));
#212945=CARTESIAN_POINT('Ctrl Pts',(-49.6009500500924,71.4148252078506,
78.7142310089962));
#212946=CARTESIAN_POINT('Ctrl Pts',(-49.5510767881416,69.745458940248,79.3558000519022));
#212947=CARTESIAN_POINT('Ctrl Pts',(-49.5327091028253,69.1106161156783,
79.5320402969566));
#212948=CARTESIAN_POINT('Ctrl Pts',(-49.4960964344567,67.8407209724448,
79.756140657928));
#212949=CARTESIAN_POINT('Ctrl Pts',(-49.4781072698155,67.2093150345555,
79.8081751924792));
#212950=CARTESIAN_POINT('Ctrl Pts',(-49.4452938123236,66.034101362473,79.7961551901444));
#212951=CARTESIAN_POINT('Ctrl Pts',(-49.4302001837212,65.4923566763925,
79.7474516421501));
#212952=CARTESIAN_POINT('Ctrl Pts',(-49.3917423264305,64.1486951600251,
79.518058201218));
#212953=CARTESIAN_POINT('Ctrl Pts',(-49.3682725668919,63.3598305636744,
79.2835506009118));
#212954=CARTESIAN_POINT('Ctrl Pts',(-49.333283631228,62.2098911532063,78.7853691760749));
#212955=CARTESIAN_POINT('Ctrl Pts',(-49.3212478541936,61.823730788727,78.5881498016359));
#212956=CARTESIAN_POINT('Ctrl Pts',(-49.2966979351889,61.0719719741154,
78.1420527743269));
#212957=CARTESIAN_POINT('Ctrl Pts',(-49.284203110542,60.7076560545366,77.8927747027456));
#212958=CARTESIAN_POINT('Ctrl Pts',(-49.2716572296685,60.3605315571557,
77.6208145648926));
#212959=CARTESIAN_POINT('Origin',(-45.8894114130409,66.6819786653733,69.5522455184007));
#212960=CARTESIAN_POINT('',(-52.0239203182307,76.1552807426645,73.4662010307169));
#212961=CARTESIAN_POINT('',(-51.6180871401245,76.1552807409204,73.4662010349383));
#212962=CARTESIAN_POINT('',(-45.8894114130409,76.1552807409204,73.4662010349383));
#212963=CARTESIAN_POINT('Ctrl Pts',(-50.2096235848679,76.1552807409204,
73.4662010349383));
#212964=CARTESIAN_POINT('Ctrl Pts',(-50.215258731149,76.2317708533604,73.2810650675328));
#212965=CARTESIAN_POINT('Ctrl Pts',(-50.2209205166869,76.3028933202327,
73.0935429919239));
#212966=CARTESIAN_POINT('Ctrl Pts',(-50.2421792944852,76.5482161061884,
72.3845326047184));
#212967=CARTESIAN_POINT('Ctrl Pts',(-50.2579032979113,76.6858529284356,
71.8515923228482));
#212968=CARTESIAN_POINT('Ctrl Pts',(-50.2878406499036,76.8685535542951,
70.8021108337046));
#212969=CARTESIAN_POINT('Ctrl Pts',(-50.3021105145622,76.9185322949097,
70.288075520397));
#212970=CARTESIAN_POINT('Ctrl Pts',(-50.3344513860224,76.9433267853221,
69.1343003712923));
#212971=CARTESIAN_POINT('Ctrl Pts',(-50.3525860612613,76.8973985777643,
68.4962506051938));
#212972=CARTESIAN_POINT('Ctrl Pts',(-50.3886731043959,76.6885542782653,
67.2435798090027));
#212973=CARTESIAN_POINT('Ctrl Pts',(-50.406205972037,76.5273071317408,66.63145727533));
#212974=CARTESIAN_POINT('Ctrl Pts',(-50.4421982095905,76.0856698302883,
65.4213772383649));
#212975=CARTESIAN_POINT('Ctrl Pts',(-50.4607485014187,75.8018687172566,
64.8277274844651));
#212976=CARTESIAN_POINT('Ctrl Pts',(-50.5113921507919,74.8836043771975,
63.3025446990711));
#212977=CARTESIAN_POINT('Ctrl Pts',(-50.5421483544674,74.1495408268806,
62.4416229161454));
#212978=CARTESIAN_POINT('Ctrl Pts',(-50.5931362890703,72.7739063837983,
61.281355191233));
#212979=CARTESIAN_POINT('Ctrl Pts',(-50.6124378411329,72.2154848808551,
60.8977936531927));
#212980=CARTESIAN_POINT('Ctrl Pts',(-50.6501790766708,71.0321009746581,
60.2466336853865));
#212981=CARTESIAN_POINT('Ctrl Pts',(-50.668911435612,70.4101277642476,59.9804704590969));
#212982=CARTESIAN_POINT('Ctrl Pts',(-50.7026488261878,69.2737759090788,
59.6218847490646));
#212983=CARTESIAN_POINT('Ctrl Pts',(-50.7174214577685,68.7699775366072,
59.5038756888099));
#212984=CARTESIAN_POINT('Ctrl Pts',(-50.7413547345326,67.9318869727926,
59.3733398517201));
#212985=CARTESIAN_POINT('Ctrl Pts',(-50.7505851433635,67.6020559068877,
59.3382428579477));
#212986=CARTESIAN_POINT('Ctrl Pts',(-50.7975213204535,65.9217355564926,
59.2415055227305));
#212987=CARTESIAN_POINT('Ctrl Pts',(-50.8360007821808,64.5702333574334,
59.4314817097669));
#212988=CARTESIAN_POINT('Ctrl Pts',(-50.9113416243312,62.0203364285534,
60.3243343480095));
#212989=CARTESIAN_POINT('Ctrl Pts',(-50.9497759551382,60.8467192401891,
61.0179025958921));
#212990=CARTESIAN_POINT('Ctrl Pts',(-51.0047808895067,59.3779771638567,
62.3341359280543));
#212991=CARTESIAN_POINT('Ctrl Pts',(-51.0221410764556,58.9534349461415,
62.7906518478777));
#212992=CARTESIAN_POINT('Ctrl Pts',(-51.0542450765866,58.2609288019876,
63.6863618893438));
#212993=CARTESIAN_POINT('Ctrl Pts',(-51.0688308864643,57.9795001410016,
64.1126185471515));
#212994=CARTESIAN_POINT('Ctrl Pts',(-51.1022187659112,57.401244650137,65.1490151296938));
#212995=CARTESIAN_POINT('Ctrl Pts',(-51.1208774390134,57.1308498382281,
65.7711860632812));
#212996=CARTESIAN_POINT('Ctrl Pts',(-51.1548729987492,56.7615727896548,
66.9199684144007));
#212997=CARTESIAN_POINT('Ctrl Pts',(-51.1699759240402,56.6387670726264,
67.436298939574));
#212998=CARTESIAN_POINT('Ctrl Pts',(-51.2117835909392,56.409960425321,68.8911604270164));
#212999=CARTESIAN_POINT('Ctrl Pts',(-51.2375992875244,56.3926845550487,
69.8382887136384));
#213000=CARTESIAN_POINT('Ctrl Pts',(-51.2824202947342,56.5816756122398,
71.4120497051338));
#213001=CARTESIAN_POINT('Ctrl Pts',(-51.3008195271194,56.7180181712124,
72.0411193268221));
#213002=CARTESIAN_POINT('Ctrl Pts',(-51.3329146097462,57.0641612981642,
73.1316242487666));
#213003=CARTESIAN_POINT('Ctrl Pts',(-51.3468118683537,57.2509199578285,
73.5981691204401));
#213004=CARTESIAN_POINT('Ctrl Pts',(-51.3702006408015,57.6168709078841,
74.3477352292522));
#213005=CARTESIAN_POINT('Ctrl Pts',(-51.3795720312953,57.777074511288,74.6390500289914));
#213006=CARTESIAN_POINT('Ctrl Pts',(-51.4025097249837,58.2006412733255,
75.3277306857662));
#213007=CARTESIAN_POINT('Ctrl Pts',(-51.4161202137029,58.4781100706131,
75.7155119559278));
#213008=CARTESIAN_POINT('Ctrl Pts',(-51.4429325966715,59.0846579218839,
76.4493165724212));
#213009=CARTESIAN_POINT('Ctrl Pts',(-51.4561078238984,59.4129517352115,
76.7944913294035));
#213010=CARTESIAN_POINT('Ctrl Pts',(-51.4875650093103,60.2430336687177,
77.5537380621337));
#213011=CARTESIAN_POINT('Ctrl Pts',(-51.5059390037119,60.7625703287845,
77.9453668480491));
#213012=CARTESIAN_POINT('Ctrl Pts',(-51.5339183197109,61.6006904643938,
78.4603850333636));
#213013=CARTESIAN_POINT('Ctrl Pts',(-51.5434030417052,61.8941545437064,
78.6214893759789));
#213014=CARTESIAN_POINT('Ctrl Pts',(-51.5729128059712,62.8412318771266,
79.0826086525093));
#213015=CARTESIAN_POINT('Ctrl Pts',(-51.5927914030891,63.5187973148232,
79.3284127139547));
#213016=CARTESIAN_POINT('Ctrl Pts',(-51.627422427949,64.7069477918233,79.6228502184274));
#213017=CARTESIAN_POINT('Ctrl Pts',(-51.64185928514,65.2057244561556,79.7079580209407));
#213018=CARTESIAN_POINT('Ctrl Pts',(-51.6735664554794,66.3219861829472,
79.8144286228162));
#213019=CARTESIAN_POINT('Ctrl Pts',(-51.690559709204,66.9392594697799,79.8175173393829));
#213020=CARTESIAN_POINT('Ctrl Pts',(-51.7267421583254,68.2253519616075,
79.7078230822468));
#213021=CARTESIAN_POINT('Ctrl Pts',(-51.7459449177058,68.8903332106317,
79.5842398505121));
#213022=CARTESIAN_POINT('Ctrl Pts',(-51.7941678792632,70.5221966859855,
79.1107358518104));
#213023=CARTESIAN_POINT('Ctrl Pts',(-51.8221806889857,71.4577310668171,
78.6793590652402));
#213024=CARTESIAN_POINT('Ctrl Pts',(-51.8681523655424,72.8122167852181,
77.7886683920298));
#213025=CARTESIAN_POINT('Ctrl Pts',(-51.8852020977137,73.2811631637889,
77.4179469403853));
#213026=CARTESIAN_POINT('Ctrl Pts',(-51.9241413610066,74.2930967616012,
76.4634319740288));
#213027=CARTESIAN_POINT('Ctrl Pts',(-51.9461415204161,74.8056691700268,
75.8529812943268));
#213028=CARTESIAN_POINT('Ctrl Pts',(-51.9865585443683,75.589107391047,74.6632673224413));
#213029=CARTESIAN_POINT('Ctrl Pts',(-52.0045251847382,75.8863758838689,
74.1062080654862));
#213030=CARTESIAN_POINT('Ctrl Pts',(-52.0227265369482,76.1388961978591,
73.505682972861));
#213031=CARTESIAN_POINT('Ctrl Pts',(-52.0233235272473,76.14711965887,73.4859540432173));
#213032=CARTESIAN_POINT('Ctrl Pts',(-52.0239203182307,76.1552807444086,
73.4662010264956));
#213033=CARTESIAN_POINT('Ctrl Pts',(-51.6180871401244,76.1552807409204,
73.4662010349383));
#213034=CARTESIAN_POINT('Ctrl Pts',(-51.608868021914,76.0304223264424,73.7684071974832));
#213035=CARTESIAN_POINT('Ctrl Pts',(-51.5995742545812,75.8909546857845,
74.0649988866438));
#213036=CARTESIAN_POINT('Ctrl Pts',(-51.5808374233716,75.5823062716353,
74.6469438444561));
#213037=CARTESIAN_POINT('Ctrl Pts',(-51.5714220806443,75.4133747445076,
74.9313259570918));
#213038=CARTESIAN_POINT('Ctrl Pts',(-51.5488061946735,74.9704115815491,
75.60100464812));
#213039=CARTESIAN_POINT('Ctrl Pts',(-51.5357249876376,74.682904723647,75.9764804561156));
#213040=CARTESIAN_POINT('Ctrl Pts',(-51.5132823918292,74.1520734221524,
76.5785749741797));
#213041=CARTESIAN_POINT('Ctrl Pts',(-51.5040042547753,73.921766249813,76.815653470945));
#213042=CARTESIAN_POINT('Ctrl Pts',(-51.4804745361526,73.3140027491484,
77.3836095300202));
#213043=CARTESIAN_POINT('Ctrl Pts',(-51.466148886558,72.9229552981338,77.6986688597706));
#213044=CARTESIAN_POINT('Ctrl Pts',(-51.4337100285468,71.9797236645986,
78.3506898251033));
#213045=CARTESIAN_POINT('Ctrl Pts',(-51.415927136167,71.4155743166433,78.6666187043906));
#213046=CARTESIAN_POINT('Ctrl Pts',(-51.3715379616585,69.9682202306324,
79.3062992100124));
#213047=CARTESIAN_POINT('Ctrl Pts',(-51.344650347868,69.0630318258767,79.5658133489809));
#213048=CARTESIAN_POINT('Ctrl Pts',(-51.3040111510123,67.6239691693562,
79.7719282461753));
#213049=CARTESIAN_POINT('Ctrl Pts',(-51.2896819770196,67.1078944552536,
79.8064084279483));
#213050=CARTESIAN_POINT('Ctrl Pts',(-51.2561246723312,65.915211626826,79.7958712874477));
#213051=CARTESIAN_POINT('Ctrl Pts',(-51.2367833257127,65.2412543980353,
79.7229927781949));
#213052=CARTESIAN_POINT('Ctrl Pts',(-51.2020430143689,64.037273773024,79.4706552983997));
#213053=CARTESIAN_POINT('Ctrl Pts',(-51.1867380171011,63.5052434517304,
79.313273794622));
#213054=CARTESIAN_POINT('Ctrl Pts',(-51.1397423602316,61.9392746274684,
78.7083636173971));
#213055=CARTESIAN_POINT('Ctrl Pts',(-51.1075820319353,60.96385046603,78.1330818339147));
#213056=CARTESIAN_POINT('Ctrl Pts',(-51.0579012620402,59.5980236625747,
76.9893960511723));
#213057=CARTESIAN_POINT('Ctrl Pts',(-51.0395589195514,59.1362774011232,
76.5204597823409));
#213058=CARTESIAN_POINT('Ctrl Pts',(-51.0029847118296,58.3245251594762,
75.5200386220687));
#213059=CARTESIAN_POINT('Ctrl Pts',(-50.9850016462149,57.9726797226433,
74.9937262870521));
#213060=CARTESIAN_POINT('Ctrl Pts',(-50.9495338631929,57.3671496842344,
73.8770771803941));
#213061=CARTESIAN_POINT('Ctrl Pts',(-50.931788174642,57.1158852502217,73.2885620467056));
#213062=CARTESIAN_POINT('Ctrl Pts',(-50.8990900924942,56.7633089730634,
72.1884355348597));
#213063=CARTESIAN_POINT('Ctrl Pts',(-50.884318789014,56.643041943573,71.6851433128602));
#213064=CARTESIAN_POINT('Ctrl Pts',(-50.8543697421257,56.4751158280907,
70.6377859722055));
#213065=CARTESIAN_POINT('Ctrl Pts',(-50.8393342677898,56.4318924015049,
70.094630897655));
#213066=CARTESIAN_POINT('Ctrl Pts',(-50.7920628773332,56.4321606123153,
68.4057208376649));
#213067=CARTESIAN_POINT('Ctrl Pts',(-50.7593468225165,56.6241629378768,
67.2689077627035));
#213068=CARTESIAN_POINT('Ctrl Pts',(-50.6897388705989,57.4435640292053,
64.9111296610566));
#213069=CARTESIAN_POINT('Ctrl Pts',(-50.6512748709611,58.1351583630064,
63.7350182101061));
#213070=CARTESIAN_POINT('Ctrl Pts',(-50.5953317222099,59.4708205207166,
62.2385426218951));
#213071=CARTESIAN_POINT('Ctrl Pts',(-50.5770569961627,59.9525180000706,
61.7930314647408));
#213072=CARTESIAN_POINT('Ctrl Pts',(-50.540579454897,60.9752307744137,61.0144877782618));
#213073=CARTESIAN_POINT('Ctrl Pts',(-50.522607632927,61.5112610278961,60.6795923034354));
#213074=CARTESIAN_POINT('Ctrl Pts',(-50.4872521942371,62.6419766901064,
60.1106238810853));
#213075=CARTESIAN_POINT('Ctrl Pts',(-50.4696151902856,63.2345912966788,
59.8784999691666));
#213076=CARTESIAN_POINT('Ctrl Pts',(-50.437442117871,64.3275149771177,59.5636879839881));
#213077=CARTESIAN_POINT('Ctrl Pts',(-50.4230938276373,64.8197308052738,
59.4603274320877));
#213078=CARTESIAN_POINT('Ctrl Pts',(-50.3908112378872,65.9508156837442,
59.3084092275465));
#213079=CARTESIAN_POINT('Ctrl Pts',(-50.3731959748618,66.5906628475814,
59.2827545477454));
#213080=CARTESIAN_POINT('Ctrl Pts',(-50.3286438051655,68.1768670943357,
59.3674848671068));
#213081=CARTESIAN_POINT('Ctrl Pts',(-50.3014079559287,69.1133879687202,
59.5496309642269));
#213082=CARTESIAN_POINT('Ctrl Pts',(-50.2559043856523,70.6532771957255,
60.0784980654637));
#213083=CARTESIAN_POINT('Ctrl Pts',(-50.2370734900478,71.2716715836135,
60.3621519386172));
#213084=CARTESIAN_POINT('Ctrl Pts',(-50.2030497788706,72.3090274993817,
60.968977524793));
#213085=CARTESIAN_POINT('Ctrl Pts',(-50.1880912515587,72.7396902152464,
61.2673015705171));
#213086=CARTESIAN_POINT('Ctrl Pts',(-50.1589096202985,73.5425331237562,
61.9196349199222));
#213087=CARTESIAN_POINT('Ctrl Pts',(-50.1447648340832,73.9146903458592,
62.2713226589861));
#213088=CARTESIAN_POINT('Ctrl Pts',(-50.1131010384993,74.6769982649702,
63.1080767011721));
#213089=CARTESIAN_POINT('Ctrl Pts',(-50.0955377374664,75.0524179368028,
63.6038521619826));
#213090=CARTESIAN_POINT('Ctrl Pts',(-50.0394765787788,76.0948692088835,
65.2763779318886));
#213091=CARTESIAN_POINT('Ctrl Pts',(-50.0025913316872,76.5756587319114,
66.5521388207159));
#213092=CARTESIAN_POINT('Ctrl Pts',(-49.9257292001042,77.0153057608379,
69.2179582231263));
#213093=CARTESIAN_POINT('Ctrl Pts',(-49.8888061641626,76.9693013427971,
70.5819990789817));
#213094=CARTESIAN_POINT('Ctrl Pts',(-49.8409269575123,76.5841559806981,
72.2204391079391));
#213095=CARTESIAN_POINT('Ctrl Pts',(-49.8314919310145,76.4926971245251,
72.5392471507234));
#213096=CARTESIAN_POINT('Ctrl Pts',(-49.8160235298243,76.3155897230452,
73.0599197033263));
#213097=CARTESIAN_POINT('Ctrl Pts',(-49.8099262462807,76.2386555387497,
73.2644014380888));
#213098=CARTESIAN_POINT('Ctrl Pts',(-49.8038356726598,76.1552807409204,
73.4662010349383));
#213099=CARTESIAN_POINT('Origin',(-45.8894114130409,66.6819786653733,69.5522455184007));
#213100=CARTESIAN_POINT('',(-53.8378263137955,76.1552807455499,73.466201023733));
#213101=CARTESIAN_POINT('',(-53.4317936414903,76.1552807404427,73.4662010360945));
#213102=CARTESIAN_POINT('',(-45.8894114130409,76.1552807409204,73.4662010349383));
#213103=CARTESIAN_POINT('Ctrl Pts',(-52.0239203182307,76.1552807444086,
73.4662010264956));
#213104=CARTESIAN_POINT('Ctrl Pts',(-52.0422770108351,76.4063075573506,
72.858618026633));
#213105=CARTESIAN_POINT('Ctrl Pts',(-52.0605483699871,76.5983190601092,
72.2282486121129));
#213106=CARTESIAN_POINT('Ctrl Pts',(-52.0942628601814,76.8342785922126,
71.0613553893792));
#213107=CARTESIAN_POINT('Ctrl Pts',(-52.109509966037,76.8990097012618,70.5314701813668));
#213108=CARTESIAN_POINT('Ctrl Pts',(-52.1377410506788,76.9426856907785,
69.5302689434039));
#213109=CARTESIAN_POINT('Ctrl Pts',(-52.1507348112528,76.9309299040568,
69.060722143021));
#213110=CARTESIAN_POINT('Ctrl Pts',(-52.1731866449851,76.8558199394255,
68.2611254536285));
#213111=CARTESIAN_POINT('Ctrl Pts',(-52.182565470545,76.8083537049086,67.9303442100052));
#213112=CARTESIAN_POINT('Ctrl Pts',(-52.2061707517896,76.6496055737009,
67.1110392915593));
#213113=CARTESIAN_POINT('Ctrl Pts',(-52.2204691358635,76.5185141995445,
66.6272430319727));
#213114=CARTESIAN_POINT('Ctrl Pts',(-52.2531015304926,76.13624179264,65.5390740212308));
#213115=CARTESIAN_POINT('Ctrl Pts',(-52.2710913175403,75.8615386249818,
64.9452597677298));
#213116=CARTESIAN_POINT('Ctrl Pts',(-52.3083464588001,75.1917083740434,
63.7987522187586));
#213117=CARTESIAN_POINT('Ctrl Pts',(-52.3275849779464,74.7944341841179,
63.2509572402287));
#213118=CARTESIAN_POINT('Ctrl Pts',(-52.3708967128673,73.7800974002242,
62.1087183049267));
#213119=CARTESIAN_POINT('Ctrl Pts',(-52.3942775022462,73.136655343858,61.5443408291167));
#213120=CARTESIAN_POINT('Ctrl Pts',(-52.4439219816563,71.6801798906722,
60.5576647839447));
#213121=CARTESIAN_POINT('Ctrl Pts',(-52.4697742856366,70.8653966181718,
60.1509939030528));
#213122=CARTESIAN_POINT('Ctrl Pts',(-52.5133914193336,69.3859793698436,
59.6435101412514));
#213123=CARTESIAN_POINT('Ctrl Pts',(-52.5317610538993,68.7450850115821,
59.4905240162853));
#213124=CARTESIAN_POINT('Ctrl Pts',(-52.5683761301054,67.4677768854099,
59.312874055583));
#213125=CARTESIAN_POINT('Ctrl Pts',(-52.5863652927878,66.834855705855,59.2839032554923));
#213126=CARTESIAN_POINT('Ctrl Pts',(-52.621881454637,65.5640769392124,59.3433129011005));
#213127=CARTESIAN_POINT('Ctrl Pts',(-52.6396720718213,64.929050677876,59.4329941080809));
#213128=CARTESIAN_POINT('Ctrl Pts',(-52.6726107951199,63.7972573546196,
59.702627298489));
#213129=CARTESIAN_POINT('Ctrl Pts',(-52.6875812703577,63.2980145759789,
59.8627986517121));
#213130=CARTESIAN_POINT('Ctrl Pts',(-52.7167181006459,62.3414922092398,
60.2526675518071));
#213131=CARTESIAN_POINT('Ctrl Pts',(-52.7308100180983,61.8847714051643,
60.4798269051936));
#213132=CARTESIAN_POINT('Ctrl Pts',(-52.7624846259668,60.911250173591,61.0581723455944));
#213133=CARTESIAN_POINT('Ctrl Pts',(-52.7801148938693,60.405791269077,61.4245124404429));
#213134=CARTESIAN_POINT('Ctrl Pts',(-52.8362389070056,58.920195166244,62.72290451597));
#213135=CARTESIAN_POINT('Ctrl Pts',(-52.873120682505,58.0891313782455,63.8034934717983));
#213136=CARTESIAN_POINT('Ctrl Pts',(-52.9499786041311,56.8929508538953,
66.2259399742553));
#213137=CARTESIAN_POINT('Ctrl Pts',(-52.9869012557287,56.5400992482972,
67.5443463850443));
#213138=CARTESIAN_POINT('Ctrl Pts',(-53.0347819082646,56.4318730028817,
69.2240060578812));
#213139=CARTESIAN_POINT('Ctrl Pts',(-53.0442180124622,56.4266191738947,
69.5556842528337));
#213140=CARTESIAN_POINT('Ctrl Pts',(-53.0681022151183,56.454357797048,70.4044855926411));
#213141=CARTESIAN_POINT('Ctrl Pts',(-53.0824246531834,56.5104483288861,
70.9199142260153));
#213142=CARTESIAN_POINT('Ctrl Pts',(-53.1266168860895,56.7992540037837,
72.4706668034623));
#213143=CARTESIAN_POINT('Ctrl Pts',(-53.1569590297803,57.1536527929157,
73.47607560508));
#213144=CARTESIAN_POINT('Ctrl Pts',(-53.1957257818166,57.8120892038211,
74.6997072152807));
#213145=CARTESIAN_POINT('Ctrl Pts',(-53.2049081400309,57.9823192739764,
74.9824597831962));
#213146=CARTESIAN_POINT('Ctrl Pts',(-53.233067126294,58.5413841432443,75.8171068980668));
#213147=CARTESIAN_POINT('Ctrl Pts',(-53.2522686043099,58.9713201288318,
76.3392548366998));
#213148=CARTESIAN_POINT('Ctrl Pts',(-53.3008078933674,60.183185559936,77.5460228505117));
#213149=CARTESIAN_POINT('Ctrl Pts',(-53.3291196223283,61.0234471184008,
78.1612994266001));
#213150=CARTESIAN_POINT('Ctrl Pts',(-53.3759450656259,62.4870612315103,
78.9247423505657));
#213151=CARTESIAN_POINT('Ctrl Pts',(-53.3935081856289,63.0570763679768,
79.1595931372414));
#213152=CARTESIAN_POINT('Ctrl Pts',(-53.4244969909968,64.1155870140249,
79.4879995130162));
#213153=CARTESIAN_POINT('Ctrl Pts',(-53.4381749346214,64.5963962045297,
79.5999278243685));
#213154=CARTESIAN_POINT('Ctrl Pts',(-53.4710148892474,65.7506402816098,
79.7821738248868));
#213155=CARTESIAN_POINT('Ctrl Pts',(-53.490309821711,66.4266669170699,79.8213070598965));
#213156=CARTESIAN_POINT('Ctrl Pts',(-53.527766563879,67.7495178345174,79.7671049500467));
#213157=CARTESIAN_POINT('Ctrl Pts',(-53.545638863395,68.3934461201163,79.6791341956534));
#213158=CARTESIAN_POINT('Ctrl Pts',(-53.5899561994073,69.9313494250157,
79.3180706904847));
#213159=CARTESIAN_POINT('Ctrl Pts',(-53.6166731041434,70.8047365182997,
78.9826552089806));
#213160=CARTESIAN_POINT('Ctrl Pts',(-53.6567756194245,72.0616229129678,
78.291527030328));
#213161=CARTESIAN_POINT('Ctrl Pts',(-53.6707331929619,72.484028000018,78.0169863498192));
#213162=CARTESIAN_POINT('Ctrl Pts',(-53.7038802475189,73.4225833970076,
77.3035970690918));
#213163=CARTESIAN_POINT('Ctrl Pts',(-53.723194591918,73.9188374929165,76.8424486978672));
#213164=CARTESIAN_POINT('Ctrl Pts',(-53.7593927199058,74.766232090873,75.882563003819));
#213165=CARTESIAN_POINT('Ctrl Pts',(-53.7760763651848,75.1254906812906,
75.3947775192488));
#213166=CARTESIAN_POINT('Ctrl Pts',(-53.8078513762937,75.7146324498198,
74.4260243596755));
#213167=CARTESIAN_POINT('Ctrl Pts',(-53.8228144662272,75.9537821606758,
73.9539063542217));
#213168=CARTESIAN_POINT('Ctrl Pts',(-53.8378263134509,76.1552807455537,
73.466201023724));
#213169=CARTESIAN_POINT('Ctrl Pts',(-53.4317936414903,76.155280739965,73.4662010372508));
#213170=CARTESIAN_POINT('Ctrl Pts',(-53.4314659962319,76.1508777158183,
73.476858076551));
#213171=CARTESIAN_POINT('Ctrl Pts',(-53.4311383819964,76.1464565428961,
73.4875080872006));
#213172=CARTESIAN_POINT('Ctrl Pts',(-53.4128952715418,75.8992278722724,
74.0802219161308));
#213173=CARTESIAN_POINT('Ctrl Pts',(-53.3954072233106,75.6032360752142,
74.6386413343921));
#213174=CARTESIAN_POINT('Ctrl Pts',(-53.3594844790862,74.8992699569684,
75.7139926929329));
#213175=CARTESIAN_POINT('Ctrl Pts',(-53.3409746459319,74.4890956478663,
76.2260685416729));
#213176=CARTESIAN_POINT('Ctrl Pts',(-53.2839183526019,73.0912392500936,
77.6645611382443));
#213177=CARTESIAN_POINT('Ctrl Pts',(-53.2470045196131,71.9671807972707,
78.4379034421667));
#213178=CARTESIAN_POINT('Ctrl Pts',(-53.1760057255058,69.6738585008067,
79.4224570090448));
#213179=CARTESIAN_POINT('Ctrl Pts',(-53.1446794675824,68.5539268955872,
79.6946439382857));
#213180=CARTESIAN_POINT('Ctrl Pts',(-53.0968240154157,66.8695047064349,
79.814968195707));
#213181=CARTESIAN_POINT('Ctrl Pts',(-53.0812542410977,66.3244701339641,
79.8104536841581));
#213182=CARTESIAN_POINT('Ctrl Pts',(-53.0514361458559,65.2676801161755,
79.7173440425143));
#213183=CARTESIAN_POINT('Ctrl Pts',(-53.0371402952996,64.7571477762161,
79.6331432604136));
#213184=CARTESIAN_POINT('Ctrl Pts',(-53.0022205705923,63.5464698036927,
79.3381092421604));
#213185=CARTESIAN_POINT('Ctrl Pts',(-52.9814285047767,62.8582526126167,
79.0902559045379));
#213186=CARTESIAN_POINT('Ctrl Pts',(-52.951284040001,61.9011854719671,78.6252011403551));
#213187=CARTESIAN_POINT('Ctrl Pts',(-52.9419242939361,61.607512904031,78.4642770173353));
#213188=CARTESIAN_POINT('Ctrl Pts',(-52.9143597158301,60.7651940655475,
77.9475554461948));
#213189=CARTESIAN_POINT('Ctrl Pts',(-52.8961354568477,60.2421097217891,
77.55334853467));
#213190=CARTESIAN_POINT('Ctrl Pts',(-52.8641346518973,59.410075329003,76.791526311064));
#213191=CARTESIAN_POINT('Ctrl Pts',(-52.8505713097694,59.0827081741547,
76.4470879423885));
#213192=CARTESIAN_POINT('Ctrl Pts',(-52.8238139978596,58.4778270199905,
75.7150387416729));
#213193=CARTESIAN_POINT('Ctrl Pts',(-52.8106602608988,58.2010832150992,
75.3282771917183));
#213194=CARTESIAN_POINT('Ctrl Pts',(-52.7880664001766,57.7775813447986,
74.6399941606678));
#213195=CARTESIAN_POINT('Ctrl Pts',(-52.7787101072543,57.6169406943703,
74.3479271681421));
#213196=CARTESIAN_POINT('Ctrl Pts',(-52.7550857351583,57.2505846291851,
73.5974083152818));
#213197=CARTESIAN_POINT('Ctrl Pts',(-52.7407446071513,57.0638046904065,
73.1306895624294));
#213198=CARTESIAN_POINT('Ctrl Pts',(-52.7084130093088,56.7181436842887,
72.041273235225));
#213199=CARTESIAN_POINT('Ctrl Pts',(-52.6907451184286,56.5820362161555,
71.4135437557124));
#213200=CARTESIAN_POINT('Ctrl Pts',(-52.6462484222969,56.3924438733585,
69.8385019542338));
#213201=CARTESIAN_POINT('Ctrl Pts',(-52.6191261781079,56.409875066736,68.8886457120217));
#213202=CARTESIAN_POINT('Ctrl Pts',(-52.5776949972587,56.6409096623561,
67.4244244104058));
#213203=CARTESIAN_POINT('Ctrl Pts',(-52.5628004968698,56.7661086461411,
66.901545438304));
#213204=CARTESIAN_POINT('Ctrl Pts',(-52.5286159491664,57.1404901287403,
65.7468748791583));
#213205=CARTESIAN_POINT('Ctrl Pts',(-52.5092323715014,57.4125885703912,
65.1251422765157));
#213206=CARTESIAN_POINT('Ctrl Pts',(-52.4763357891551,57.9838006896954,
64.1075959623724));
#213207=CARTESIAN_POINT('Ctrl Pts',(-52.462775196895,58.253933658796,63.6981383530843));
#213208=CARTESIAN_POINT('Ctrl Pts',(-52.4309630398224,58.9467892134872,
62.7958510850989));
#213209=CARTESIAN_POINT('Ctrl Pts',(-52.4126301421501,59.3890721713321,
62.3206812564263));
#213210=CARTESIAN_POINT('Ctrl Pts',(-52.3846926948985,60.1232844105761,
61.6682144426206));
#213211=CARTESIAN_POINT('Ctrl Pts',(-52.3752083042255,60.3840820643844,
61.4583639214501));
#213212=CARTESIAN_POINT('Ctrl Pts',(-52.3457945900397,61.2332793232641,
60.8409940997788));
#213213=CARTESIAN_POINT('Ctrl Pts',(-52.3260119706135,61.8543300575416,
60.4820724925773));
#213214=CARTESIAN_POINT('Ctrl Pts',(-52.2915787960311,62.9660902412387,
59.9863372313077));
#213215=CARTESIAN_POINT('Ctrl Pts',(-52.27724080382,63.4388995537073,59.8158774645287));
#213216=CARTESIAN_POINT('Ctrl Pts',(-52.2448876252375,64.5403538432876,
59.507953324019));
#213217=CARTESIAN_POINT('Ctrl Pts',(-52.2271965762748,65.1732813415432,
59.3935941786054));
#213218=CARTESIAN_POINT('Ctrl Pts',(-52.182722997773,66.7531234704477,59.2591326564387));
#213219=CARTESIAN_POINT('Ctrl Pts',(-52.1556494594568,67.7000717842061,
59.3093587972366));
#213220=CARTESIAN_POINT('Ctrl Pts',(-52.1143881196541,69.1494645880636,
59.5894407375375));
#213221=CARTESIAN_POINT('Ctrl Pts',(-52.0996164392368,69.6635432057282,
59.7310318151772));
#213222=CARTESIAN_POINT('Ctrl Pts',(-52.0655683577469,70.8008720402759,
60.1418613680364));
#213223=CARTESIAN_POINT('Ctrl Pts',(-52.0461939530619,71.4131075471757,
60.4342951777518));
#213224=CARTESIAN_POINT('Ctrl Pts',(-52.0129298404671,72.4219705123723,
61.0453279018358));
#213225=CARTESIAN_POINT('Ctrl Pts',(-51.999021691533,72.8321732375763,61.3369996558632));
#213226=CARTESIAN_POINT('Ctrl Pts',(-51.9673054183399,73.7055664631982,
62.0602315082084));
#213227=CARTESIAN_POINT('Ctrl Pts',(-51.9494382004535,74.1535709799477,
62.5069382812588));
#213228=CARTESIAN_POINT('Ctrl Pts',(-51.8930940034553,75.4213424280378,
64.0289120405076));
#213229=CARTESIAN_POINT('Ctrl Pts',(-51.8562261475554,76.0718418595893,
65.2262598337549));
#213230=CARTESIAN_POINT('Ctrl Pts',(-51.7793862998523,76.8721659737517,
67.8060300810223));
#213231=CARTESIAN_POINT('Ctrl Pts',(-51.7424659076742,77.0133878904221,
69.1634389134832));
#213232=CARTESIAN_POINT('Ctrl Pts',(-51.6749180973905,76.791730248281,71.5275396952808));
#213233=CARTESIAN_POINT('Ctrl Pts',(-51.6468253635685,76.5444946475245,
72.5241512610753));
#213234=CARTESIAN_POINT('Ctrl Pts',(-51.6180871401245,76.1552807409204,
73.4662010349383));
#213235=CARTESIAN_POINT('Origin',(-45.8894114130409,66.6819786653733,69.5522455184007));
#213236=CARTESIAN_POINT('',(-55.6519493945588,76.1552807409204,73.4662010349383));
#213237=CARTESIAN_POINT('',(-55.2458788384028,76.1552807409204,73.4662010349383));
#213238=CARTESIAN_POINT('',(-45.8894114130409,76.1552807409204,73.4662010349383));
#213239=CARTESIAN_POINT('',(-54.9945936623312,57.5592308793253,74.2253572046497));
#213240=CARTESIAN_POINT('Ctrl Pts',(-54.9945936623312,57.5592308793253,
74.2253572046497));
#213241=CARTESIAN_POINT('Ctrl Pts',(-55.0084372590718,57.7855821470804,
74.6672352647992));
#213242=CARTESIAN_POINT('Ctrl Pts',(-55.0223123077768,58.0437377263266,
75.0920812588877));
#213243=CARTESIAN_POINT('Ctrl Pts',(-55.0500493198654,58.6121913701251,
75.8906232303414));
#213244=CARTESIAN_POINT('Ctrl Pts',(-55.0638656775378,58.920268216079,76.2643500438473));
#213245=CARTESIAN_POINT('Ctrl Pts',(-55.1051653283116,59.9255405894118,
77.3216780637746));
#213246=CARTESIAN_POINT('Ctrl Pts',(-55.1318714947715,60.6949359305111,
77.9289311633348));
#213247=CARTESIAN_POINT('Ctrl Pts',(-55.1730512387199,61.9505392495489,
78.6573496489838));
#213248=CARTESIAN_POINT('Ctrl Pts',(-55.1866646088001,62.3787647802416,
78.8673832391282));
#213249=CARTESIAN_POINT('Ctrl Pts',(-55.2150290111367,63.311710122981,79.2468586413377));
#213250=CARTESIAN_POINT('Ctrl Pts',(-55.2297040018442,63.8181737520004,
79.4083533588378));
#213251=CARTESIAN_POINT('Ctrl Pts',(-55.2635851799419,64.9956836599146,
79.6853476283084));
#213252=CARTESIAN_POINT('Ctrl Pts',(-55.2828822587737,65.6703126693746,
79.7747630098718));
#213253=CARTESIAN_POINT('Ctrl Pts',(-55.3200521570506,66.9784724279672,
79.8173075347476));
#213254=CARTESIAN_POINT('Ctrl Pts',(-55.337507810066,67.6086897567368,79.7796897600188));
#213255=CARTESIAN_POINT('Ctrl Pts',(-55.3773061078025,69.0158950847412,
79.5644914169816));
#213256=CARTESIAN_POINT('Ctrl Pts',(-55.3998750351786,69.7837514486007,
79.353837768276));
#213257=CARTESIAN_POINT('Ctrl Pts',(-55.4392788189713,71.0726734457158,
78.8334141112913));
#213258=CARTESIAN_POINT('Ctrl Pts',(-55.4557763960126,71.6052193096335,
78.5622396134129));
#213259=CARTESIAN_POINT('Ctrl Pts',(-55.5011128136525,72.9800616350833,
77.7036912942383));
#213260=CARTESIAN_POINT('Ctrl Pts',(-55.5304852313319,73.7627295822315,
77.0338820012117));
#213261=CARTESIAN_POINT('Ctrl Pts',(-55.577991334307,74.8745375971509,75.7489967300131));
#213262=CARTESIAN_POINT('Ctrl Pts',(-55.5966995204025,75.2645755879978,
75.1964263112878));
#213263=CARTESIAN_POINT('Ctrl Pts',(-55.6251264558726,75.7602715179669,
74.3225663411172));
#213264=CARTESIAN_POINT('Ctrl Pts',(-55.6345161010389,75.9091114434636,
74.027888642471));
#213265=CARTESIAN_POINT('Ctrl Pts',(-55.646586044891,76.0819598875626,73.6402500653772));
#213266=CARTESIAN_POINT('Ctrl Pts',(-55.6492703896237,76.1192295478691,
73.5534590123262));
#213267=CARTESIAN_POINT('Ctrl Pts',(-55.6519493945588,76.1552807409204,
73.4662010349383));
#213268=CARTESIAN_POINT('Ctrl Pts',(-53.8378263134509,76.1552807455537,
73.466201023724));
#213269=CARTESIAN_POINT('Ctrl Pts',(-53.8522474144839,76.3488499584049,
72.9976878727012));
#213270=CARTESIAN_POINT('Ctrl Pts',(-53.8665858984656,76.5076744897429,
72.5147867212634));
#213271=CARTESIAN_POINT('Ctrl Pts',(-53.8899527568025,76.7093946581641,
71.7020543778137));
#213272=CARTESIAN_POINT('Ctrl Pts',(-53.8991093787747,76.7732299909849,
71.3790996265538));
#213273=CARTESIAN_POINT('Ctrl Pts',(-53.9378312622193,76.9756655140685,
70.0119776316187));
#213274=CARTESIAN_POINT('Ctrl Pts',(-53.9679861255333,76.9684723074621,
68.952747027349));
#213275=CARTESIAN_POINT('Ctrl Pts',(-54.0065619492763,76.7473926300935,
67.5879195820092));
#213276=CARTESIAN_POINT('Ctrl Pts',(-54.0157365034357,76.6790277257479,
67.2652946459151));
#213277=CARTESIAN_POINT('Ctrl Pts',(-54.0539158267811,76.3327208626224,
65.9477968743099));
#213278=CARTESIAN_POINT('Ctrl Pts',(-54.083497459971,75.9207775580982,64.9944523687732));
#213279=CARTESIAN_POINT('Ctrl Pts',(-54.1214905131542,75.1990667965299,
63.839992244076));
#213280=CARTESIAN_POINT('Ctrl Pts',(-54.1306414926061,75.0114421441789,
63.5697154926513));
#213281=CARTESIAN_POINT('Ctrl Pts',(-54.1695411982524,74.1656992385936,
62.468507946713));
#213282=CARTESIAN_POINT('Ctrl Pts',(-54.1998831053543,73.3938081254763,
61.7332453362441));
#213283=CARTESIAN_POINT('Ctrl Pts',(-54.2386496142671,72.2519730235472,
60.9414114358815));
#213284=CARTESIAN_POINT('Ctrl Pts',(-54.247831961414,71.9720065996045,60.7666377017056));
#213285=CARTESIAN_POINT('Ctrl Pts',(-54.2759909336803,71.0951687493672,
60.2763886497195));
#213286=CARTESIAN_POINT('Ctrl Pts',(-54.2951924069054,70.4751608137961,
60.0060672344893));
#213287=CARTESIAN_POINT('Ctrl Pts',(-54.3437331660042,68.8477003097819,
59.4802772900666));
#213288=CARTESIAN_POINT('Ctrl Pts',(-54.3720462930882,67.8197122229352,
59.3130826041624));
#213289=CARTESIAN_POINT('Ctrl Pts',(-54.4188763753811,66.168872058537,59.2966184682286));
#213290=CARTESIAN_POINT('Ctrl Pts',(-54.4364425234928,65.5542343895586,
59.3459056636689));
#213291=CARTESIAN_POINT('Ctrl Pts',(-54.4674489004025,64.4613015187775,
59.5335287842442));
#213292=CARTESIAN_POINT('Ctrl Pts',(-54.4811414040499,63.9815337580726,
59.6520591737922));
#213293=CARTESIAN_POINT('Ctrl Pts',(-54.5139972835219,62.8697597235691,
60.0135963485974));
#213294=CARTESIAN_POINT('Ctrl Pts',(-54.5332931809973,62.2495741251418,
60.2854976560029));
#213295=CARTESIAN_POINT('Ctrl Pts',(-54.5706830646895,61.0973819238806,
60.9329499567827));
#213296=CARTESIAN_POINT('Ctrl Pts',(-54.5884923418836,60.5652905220523,
61.3020270385938));
#213297=CARTESIAN_POINT('Ctrl Pts',(-54.6328612068691,59.3565286821881,
62.3220677315632));
#213298=CARTESIAN_POINT('Ctrl Pts',(-54.6596992020544,58.7275211877893,
63.0204538552515));
#213299=CARTESIAN_POINT('Ctrl Pts',(-54.7001769534581,57.9141518712627,
64.2183634506065));
#213300=CARTESIAN_POINT('Ctrl Pts',(-54.7143931148832,57.6584966712826,
64.6632929281237));
#213301=CARTESIAN_POINT('Ctrl Pts',(-54.7478249708634,57.1452019521253,
65.735247376952));
#213302=CARTESIAN_POINT('Ctrl Pts',(-54.7671576445172,56.9142648049202,
66.3724127761249));
#213303=CARTESIAN_POINT('Ctrl Pts',(-54.8023434816488,56.6075074454265,
67.5794990132264));
#213304=CARTESIAN_POINT('Ctrl Pts',(-54.8180706895508,56.5134928585929,
68.14206878208));
#213305=CARTESIAN_POINT('Ctrl Pts',(-54.8604034816512,56.3892128592203,
69.6485737620773));
#213306=CARTESIAN_POINT('Ctrl Pts',(-54.8874311493389,56.4415970092537,
70.5938250436981));
#213307=CARTESIAN_POINT('Ctrl Pts',(-54.9270660553076,56.7131276846823,
71.9829717459558));
#213308=CARTESIAN_POINT('Ctrl Pts',(-54.9401815920977,56.8359557255954,
72.4405415227217));
#213309=CARTESIAN_POINT('Ctrl Pts',(-54.9670530131731,57.1478277224444,
73.3466886280764));
#213310=CARTESIAN_POINT('Ctrl Pts',(-54.9807860052725,57.3380653584498,
73.7936026652801));
#213311=CARTESIAN_POINT('Ctrl Pts',(-54.9945874883696,57.5592309567654,
74.2253573558264));
#213312=CARTESIAN_POINT('Ctrl Pts',(-55.2458788384028,76.1552807409204,
73.4662010349383));
#213313=CARTESIAN_POINT('Ctrl Pts',(-55.2243124915029,75.8599701795553,
74.180968012256));
#213314=CARTESIAN_POINT('Ctrl Pts',(-55.2025647280681,75.4840079051681,
74.8617220383151));
#213315=CARTESIAN_POINT('Ctrl Pts',(-55.1469981393143,74.3515537139317,
76.4532424940862));
#213316=CARTESIAN_POINT('Ctrl Pts',(-55.1147951169291,73.5096645610282,
77.2871576634901));
#213317=CARTESIAN_POINT('Ctrl Pts',(-55.0664437014297,72.1104937279418,
78.2628168623936));
#213318=CARTESIAN_POINT('Ctrl Pts',(-55.051298710415,71.6533815832847,78.5315542634988));
#213319=CARTESIAN_POINT('Ctrl Pts',(-55.0173903034329,70.5696060050378,
79.0604785237848));
#213320=CARTESIAN_POINT('Ctrl Pts',(-54.9987323542363,69.9337692211884,
79.2962698052724));
#213321=CARTESIAN_POINT('Ctrl Pts',(-54.9581124061482,68.5394305632959,
79.6615195359488));
#213322=CARTESIAN_POINT('Ctrl Pts',(-54.9361746118771,67.7801351488511,
79.7719133506492));
#213323=CARTESIAN_POINT('Ctrl Pts',(-54.8958423061881,66.3409028041523,
79.818789892051));
#213324=CARTESIAN_POINT('Ctrl Pts',(-54.877165535705,65.6656342445293,79.7740512914097));
#213325=CARTESIAN_POINT('Ctrl Pts',(-54.8389851930708,64.3325458542862,
79.5522483951396));
#213326=CARTESIAN_POINT('Ctrl Pts',(-54.8196031415924,63.6780289190024,
79.3754927901739));
#213327=CARTESIAN_POINT('Ctrl Pts',(-54.7817047194038,62.4142616155419,
78.8959714791988));
#213328=CARTESIAN_POINT('Ctrl Pts',(-54.7630394630545,61.8080437372174,
78.594556454494));
#213329=CARTESIAN_POINT('Ctrl Pts',(-54.7240902845646,60.6392221738559,
77.8614960599658));
#213330=CARTESIAN_POINT('Ctrl Pts',(-54.7039000764441,60.0827100559538,
77.4267749513204));
#213331=CARTESIAN_POINT('Ctrl Pts',(-54.6702884916899,59.2185387844903,
76.5952922282852));
#213332=CARTESIAN_POINT('Ctrl Pts',(-54.6565774184773,58.8872209795158,
76.2267639897297));
#213333=CARTESIAN_POINT('Ctrl Pts',(-54.625092293712,58.199101303284,75.3399177304646));
#213334=CARTESIAN_POINT('Ctrl Pts',(-54.6072442516165,57.8607302600861,
74.8098040166607));
#213335=CARTESIAN_POINT('Ctrl Pts',(-54.5715079278915,57.2838667216351,
73.6917566269042));
#213336=CARTESIAN_POINT('Ctrl Pts',(-54.554027115688,57.0470780046594,73.1059411198935));
#213337=CARTESIAN_POINT('Ctrl Pts',(-54.5181163178736,56.6773304307878,
71.875511919092));
#213338=CARTESIAN_POINT('Ctrl Pts',(-54.4996139683888,56.549466915596,71.2323477821425));
#213339=CARTESIAN_POINT('Ctrl Pts',(-54.4495571938241,56.3727762684054,
69.4814802870216));
#213340=CARTESIAN_POINT('Ctrl Pts',(-54.4193029272258,56.440451973092,68.3708037207158));
#213341=CARTESIAN_POINT('Ctrl Pts',(-54.372011124297,56.808511139124,66.7424089895317));
#213342=CARTESIAN_POINT('Ctrl Pts',(-54.355871334505,56.9780284385155,66.2035297033478));
#213343=CARTESIAN_POINT('Ctrl Pts',(-54.3256092730652,57.3848256021668,
65.2061158091956));
#213344=CARTESIAN_POINT('Ctrl Pts',(-54.3114066674863,57.6140630165044,
64.7461235116986));
#213345=CARTESIAN_POINT('Ctrl Pts',(-54.2704474398064,58.3621786160401,
63.4906836068886));
#213346=CARTESIAN_POINT('Ctrl Pts',(-54.2432433980074,58.9582583690056,
62.7474123375254));
#213347=CARTESIAN_POINT('Ctrl Pts',(-54.1978537859097,60.1386360227913,
61.6337711224434));
#213348=CARTESIAN_POINT('Ctrl Pts',(-54.1791599386208,60.6738137336899,
61.2204075412817));
#213349=CARTESIAN_POINT('Ctrl Pts',(-54.1507294596653,61.5259552401333,
60.6873033667533));
#213350=CARTESIAN_POINT('Ctrl Pts',(-54.1413243075175,61.8145190729074,
60.5256396912466));
#213351=CARTESIAN_POINT('Ctrl Pts',(-54.106385453136,62.914022822591,59.9777370919764));
#213352=CARTESIAN_POINT('Ctrl Pts',(-54.0816685970493,63.766804995361,59.6845977050456));
#213353=CARTESIAN_POINT('Ctrl Pts',(-54.0333038138775,65.4517072700732,
59.3432611125962));
#213354=CARTESIAN_POINT('Ctrl Pts',(-54.0097423741449,66.2732798037355,
59.2775239016227));
#213355=CARTESIAN_POINT('Ctrl Pts',(-53.9731697700608,67.5786574994477,
59.3300208643908));
#213356=CARTESIAN_POINT('Ctrl Pts',(-53.9597186847645,68.0614602011573,
59.3839151786058));
#213357=CARTESIAN_POINT('Ctrl Pts',(-53.9265874021746,69.2224689976322,
59.5977533672385));
#213358=CARTESIAN_POINT('Ctrl Pts',(-53.9067471765375,69.8917217836102,
59.7929660144528));
#213359=CARTESIAN_POINT('Ctrl Pts',(-53.8775898947858,70.8458210187467,
60.1801224750558));
#213360=CARTESIAN_POINT('Ctrl Pts',(-53.8682463981352,71.1492749555572,
60.3209109392519));
#213361=CARTESIAN_POINT('Ctrl Pts',(-53.8411009308922,72.0110396946509,
60.7731898745245));
#213362=CARTESIAN_POINT('Ctrl Pts',(-53.8232780321355,72.5477690435606,
61.1223460234573));
#213363=CARTESIAN_POINT('Ctrl Pts',(-53.7910712414706,73.4377327987901,
61.8276766968787));
#213364=CARTESIAN_POINT('Ctrl Pts',(-53.7768719520978,73.8040404404524,
62.1640512086842));
#213365=CARTESIAN_POINT('Ctrl Pts',(-53.7438427360603,74.6085507419804,
63.0184749854055));
#213366=CARTESIAN_POINT('Ctrl Pts',(-53.7251832826996,75.0226277241806,
63.5560561509127));
#213367=CARTESIAN_POINT('Ctrl Pts',(-53.6910623951486,75.6633881270673,
64.5841027553956));
#213368=CARTESIAN_POINT('Ctrl Pts',(-53.6758314564432,75.9101849166998,
65.0590995070581));
#213369=CARTESIAN_POINT('Ctrl Pts',(-53.6338431560758,76.4875329605039,
66.4208152873592));
#213370=CARTESIAN_POINT('Ctrl Pts',(-53.6079792362328,76.7342739860762,
67.3372712705771));
#213371=CARTESIAN_POINT('Ctrl Pts',(-53.5631322447755,76.9319766110032,
68.9108520115754));
#213372=CARTESIAN_POINT('Ctrl Pts',(-53.5447588668118,76.9520249426517,
69.5533128542441));
#213373=CARTESIAN_POINT('Ctrl Pts',(-53.5126853153771,76.8805045666242,
70.6944122332943));
#213374=CARTESIAN_POINT('Ctrl Pts',(-53.4987850526581,76.812344483354,71.1924183457376));
#213375=CARTESIAN_POINT('Ctrl Pts',(-53.4672275751477,76.5783393297752,
72.2932815484876));
#213376=CARTESIAN_POINT('Ctrl Pts',(-53.4495081764723,76.3933355363178,
72.8900153894336));
#213377=CARTESIAN_POINT('Ctrl Pts',(-53.4317936414903,76.155280739965,73.4662010372508));
#213378=CARTESIAN_POINT('Origin',(-45.8894114130409,66.6819786653733,69.5522455184007));
#213379=CARTESIAN_POINT('',(-57.4656305641639,76.1552807494535,73.4662010142848));
#213380=CARTESIAN_POINT('',(-57.0597576325586,76.1552807409204,73.4662010349383));
#213381=CARTESIAN_POINT('',(-45.8894114130409,76.1552807409204,73.4662010349383));
#213382=CARTESIAN_POINT('Ctrl Pts',(-55.6519493945588,76.1552807409204,
73.4662010349383));
#213383=CARTESIAN_POINT('Ctrl Pts',(-55.6746958093889,76.4613777478853,
72.7253266435083));
#213384=CARTESIAN_POINT('Ctrl Pts',(-55.6967311479311,76.6796366011113,
71.9507821246546));
#213385=CARTESIAN_POINT('Ctrl Pts',(-55.7421069158573,76.9322895411356,
70.3583648508813));
#213386=CARTESIAN_POINT('Ctrl Pts',(-55.7653466256031,76.9639372508576,
69.5460762671887));
#213387=CARTESIAN_POINT('Ctrl Pts',(-55.806925292861,76.8460434176339,68.0656456112224));
#213388=CARTESIAN_POINT('Ctrl Pts',(-55.82560912636,76.7261109082097,67.3996653582486));
#213389=CARTESIAN_POINT('Ctrl Pts',(-55.8578065452673,76.4146828609178,
66.3037895256571));
#213390=CARTESIAN_POINT('Ctrl Pts',(-55.8710467590946,76.2575969551468,
65.8663903296937));
#213391=CARTESIAN_POINT('Ctrl Pts',(-55.9015061502112,75.8269700354966,
64.8828707740773));
#213392=CARTESIAN_POINT('Ctrl Pts',(-55.9183723033464,75.5332283220548,
64.3475064800913));
#213393=CARTESIAN_POINT('Ctrl Pts',(-55.9642808919294,74.6185712654834,
62.984258552835));
#213394=CARTESIAN_POINT('Ctrl Pts',(-55.9938741312891,73.9172839314932,
62.2188756965993));
#213395=CARTESIAN_POINT('Ctrl Pts',(-56.0415967105518,72.5881977023298,
61.1478221903385));
#213396=CARTESIAN_POINT('Ctrl Pts',(-56.0603060724811,72.0223100023036,
60.7773600349768));
#213397=CARTESIAN_POINT('Ctrl Pts',(-56.088732412173,71.1316852544978,60.3125792487002));
#213398=CARTESIAN_POINT('Ctrl Pts',(-56.0981205329324,70.8320354863306,
60.1741674261336));
#213399=CARTESIAN_POINT('Ctrl Pts',(-56.1376559883003,69.543270156717,59.6527561343609));
#213400=CARTESIAN_POINT('Ctrl Pts',(-56.1666755817687,68.5045214558714,
59.4099960162732));
#213401=CARTESIAN_POINT('Ctrl Pts',(-56.213397765002,66.8588571896004,59.2868087178602));
#213402=CARTESIAN_POINT('Ctrl Pts',(-56.2302860349057,66.2678997718162,
59.2936382150129));
#213403=CARTESIAN_POINT('Ctrl Pts',(-56.2658276588423,65.0081500307784,
59.4172744788482));
#213404=CARTESIAN_POINT('Ctrl Pts',(-56.2844862109658,64.3436587722586,
59.5496654525987));
#213405=CARTESIAN_POINT('Ctrl Pts',(-56.3178429932004,63.2122255775121,
59.8940807117341));
#213406=CARTESIAN_POINT('Ctrl Pts',(-56.3322909912631,62.7390163823665,
60.0774169095307));
#213407=CARTESIAN_POINT('Ctrl Pts',(-56.3642103686336,61.7233069579406,
60.5602593341932));
#213408=CARTESIAN_POINT('Ctrl Pts',(-56.3813164175117,61.1904262552062,
60.8754319085674));
#213409=CARTESIAN_POINT('Ctrl Pts',(-56.4168192794982,60.1603499538491,
61.6177787778474));
#213410=CARTESIAN_POINT('Ctrl Pts',(-56.4352685726779,59.6690857904514,
62.0484650065876));
#213411=CARTESIAN_POINT('Ctrl Pts',(-56.4847043251642,58.4771130954218,
63.3134442904562));
#213412=CARTESIAN_POINT('Ctrl Pts',(-56.5144312187865,57.8625515955255,
64.2174375450141));
#213413=CARTESIAN_POINT('Ctrl Pts',(-56.5614677909185,57.1575056607049,
65.7211836639762));
#213414=CARTESIAN_POINT('Ctrl Pts',(-56.5779136226738,56.9577674094946,
66.2609931461306));
#213415=CARTESIAN_POINT('Ctrl Pts',(-56.6084175060458,56.6677089626359,
67.307583325813));
#213416=CARTESIAN_POINT('Ctrl Pts',(-56.6225730702787,56.5681892132335,
67.810013278484));
#213417=CARTESIAN_POINT('Ctrl Pts',(-56.6547733103649,56.4298267965272,
68.9504896347172));
#213418=CARTESIAN_POINT('Ctrl Pts',(-56.6728850392413,56.4122481955756,
69.5889895371447));
#213419=CARTESIAN_POINT('Ctrl Pts',(-56.7089331308968,56.4955145498018,
70.8549562551205));
#213420=CARTESIAN_POINT('Ctrl Pts',(-56.7264522871935,56.5950685835595,
71.4797711172831));
#213421=CARTESIAN_POINT('Ctrl Pts',(-56.7624239808063,56.9139695724793,
72.7269537020968));
#213422=CARTESIAN_POINT('Ctrl Pts',(-56.7809628328593,57.1370950324909,
73.3453913173354));
#213423=CARTESIAN_POINT('Ctrl Pts',(-56.8380682761259,57.9960908523302,
75.1597803461317));
#213424=CARTESIAN_POINT('Ctrl Pts',(-56.8749886634776,58.8103360011574,
76.2549562375439));
#213425=CARTESIAN_POINT('Ctrl Pts',(-56.9393984543463,60.4909328726403,
77.7721164903898));
#213426=CARTESIAN_POINT('Ctrl Pts',(-56.9645961674213,61.2469785226243,
78.2904440043893));
#213427=CARTESIAN_POINT('Ctrl Pts',(-57.0145366542064,62.8336518914627,
79.0916868218928));
#213428=CARTESIAN_POINT('Ctrl Pts',(-57.0393538750368,63.6519495740406,
79.3822755591976));
#213429=CARTESIAN_POINT('Ctrl Pts',(-57.082448978218,65.1565013419189,79.7105473689902));
#213430=CARTESIAN_POINT('Ctrl Pts',(-57.1011421541805,65.8286271481142,
79.788942745876));
#213431=CARTESIAN_POINT('Ctrl Pts',(-57.1385964345675,67.1532251391229,
79.8120024934277));
#213432=CARTESIAN_POINT('Ctrl Pts',(-57.1572121997389,67.8024927481622,
79.7615130239616));
#213433=CARTESIAN_POINT('Ctrl Pts',(-57.1894880445944,68.9360918926912,
79.5638593128264));
#213434=CARTESIAN_POINT('Ctrl Pts',(-57.2033605279661,69.4226124385091,
79.4417534316169));
#213435=CARTESIAN_POINT('Ctrl Pts',(-57.2374376203684,70.5764964570531,
79.0604255012093));
#213436=CARTESIAN_POINT('Ctrl Pts',(-57.2578086786501,71.2294539039164,
78.7659963548634));
#213437=CARTESIAN_POINT('Ctrl Pts',(-57.294600289576,72.3514686598769,78.1115201994638));
#213438=CARTESIAN_POINT('Ctrl Pts',(-57.3107630531777,72.8303406105761,
77.7742857865217));
#213439=CARTESIAN_POINT('Ctrl Pts',(-57.355556261234,74.0559448204746,76.7439384096182));
#213440=CARTESIAN_POINT('Ctrl Pts',(-57.3847050489666,74.7324172633522,
75.9776842499415));
#213441=CARTESIAN_POINT('Ctrl Pts',(-57.4306208500471,75.6251682462822,
74.5993554303877));
#213442=CARTESIAN_POINT('Ctrl Pts',(-57.4479646045207,75.9164493598438,
74.0442663252789));
#213443=CARTESIAN_POINT('Ctrl Pts',(-57.4656305635332,76.1552807494603,
73.4662010142683));
#213444=CARTESIAN_POINT('',(-56.4026916770479,57.5592259231377,74.2253475292746));
#213445=CARTESIAN_POINT('Ctrl Pts',(-56.4026916770479,57.5592259231377,
74.2253475292746));
#213446=CARTESIAN_POINT('Ctrl Pts',(-56.389088155609,57.3368004938124,73.7911322712726));
#213447=CARTESIAN_POINT('Ctrl Pts',(-56.3754551144229,57.1456610282986,
73.3415934269327));
#213448=CARTESIAN_POINT('Ctrl Pts',(-56.3481953671734,56.8327947824228,
72.4301667046301));
#213449=CARTESIAN_POINT('Ctrl Pts',(-56.3346117192863,56.7098440227171,
71.9699678589818));
#213450=CARTESIAN_POINT('Ctrl Pts',(-56.2942042303519,56.4384143469144,
70.5697661844793));
#213451=CARTESIAN_POINT('Ctrl Pts',(-56.2681802563034,56.3881991142826,
69.6159961022789));
#213452=CARTESIAN_POINT('Ctrl Pts',(-56.2257203683172,56.5173224467139,
68.1230596009114));
#213453=CARTESIAN_POINT('Ctrl Pts',(-56.2100416967376,56.6082508580759,
67.5817580222648));
#213454=CARTESIAN_POINT('Ctrl Pts',(-56.1756348109084,56.907086450217,66.3945036641586));
#213455=CARTESIAN_POINT('Ctrl Pts',(-56.1569777938711,57.1366591444924,
65.7566249072161));
#213456=CARTESIAN_POINT('Ctrl Pts',(-56.1233002220583,57.6502426864429,
64.6779224322218));
#213457=CARTESIAN_POINT('Ctrl Pts',(-56.1085221247771,57.9083002920568,
64.2274129090497));
#213458=CARTESIAN_POINT('Ctrl Pts',(-56.0671772523844,58.7259404725428,
63.0220068134701));
#213459=CARTESIAN_POINT('Ctrl Pts',(-56.0414886867618,59.3566494640493,
62.3216082655819));
#213460=CARTESIAN_POINT('Ctrl Pts',(-55.9967337203048,60.5666241009019,
61.3011483520127));
#213461=CARTESIAN_POINT('Ctrl Pts',(-55.9782634496156,61.097590930154,60.9329191081807));
#213462=CARTESIAN_POINT('Ctrl Pts',(-55.9412289858562,62.2484962784064,
60.2860127608426));
#213463=CARTESIAN_POINT('Ctrl Pts',(-55.9225668534959,62.8686539055051,
60.0140383592924));
#213464=CARTESIAN_POINT('Ctrl Pts',(-55.8833053485378,64.1915962962261,
59.5836618985219));
#213465=CARTESIAN_POINT('Ctrl Pts',(-55.8627876392765,64.8934658696332,
59.4341481077287));
#213466=CARTESIAN_POINT('Ctrl Pts',(-55.8238098344682,66.2766548428917,
59.2880291180159));
#213467=CARTESIAN_POINT('Ctrl Pts',(-55.8051399099569,66.9535088606638,
59.2836184812238));
#213468=CARTESIAN_POINT('Ctrl Pts',(-55.7665497361985,68.3141750195008,
59.40945217659));
#213469=CARTESIAN_POINT('Ctrl Pts',(-55.7467365157939,68.9942841791439,
59.5425714904494));
#213470=CARTESIAN_POINT('Ctrl Pts',(-55.7084286876881,70.3020656894231,
59.9390509222948));
#213471=CARTESIAN_POINT('Ctrl Pts',(-55.6897617569757,70.9273840402981,
60.1983651290787));
#213472=CARTESIAN_POINT('Ctrl Pts',(-55.6509522504458,72.1389852901321,
60.8475054328729));
#213473=CARTESIAN_POINT('Ctrl Pts',(-55.6309086384268,72.719923744177,61.239926358534));
#213474=CARTESIAN_POINT('Ctrl Pts',(-55.5974228927443,73.6364737528791,
62.0061903735278));
#213475=CARTESIAN_POINT('Ctrl Pts',(-55.5836980689193,73.9930298871489,
62.3511009808872));
#213476=CARTESIAN_POINT('Ctrl Pts',(-55.5521817069278,74.7419573403004,
63.1887643642372));
#213477=CARTESIAN_POINT('Ctrl Pts',(-55.5343160631464,75.1167285258278,
63.6945898270689));
#213478=CARTESIAN_POINT('Ctrl Pts',(-55.4985615269735,75.7701296843823,
64.7704486766459));
#213479=CARTESIAN_POINT('Ctrl Pts',(-55.4810803503927,76.0470085755227,
65.3384244954077));
#213480=CARTESIAN_POINT('Ctrl Pts',(-55.4451689454345,76.5012685317673,
66.5402490532224));
#213481=CARTESIAN_POINT('Ctrl Pts',(-55.4266662118752,76.6734640365655,
67.1730058975518));
#213482=CARTESIAN_POINT('Ctrl Pts',(-55.3696226465601,77.0127962394095,
69.149469887891));
#213483=CARTESIAN_POINT('Ctrl Pts',(-55.3327110137903,76.975882711877,70.5132611827388));
#213484=CARTESIAN_POINT('Ctrl Pts',(-55.2779314050506,76.5478670960637,
72.3906925793006));
#213485=CARTESIAN_POINT('Ctrl Pts',(-55.2618238758761,76.3736180415815,
72.9377394326584));
#213486=CARTESIAN_POINT('Ctrl Pts',(-55.2458788384028,76.1552807409204,
73.4662010349383));
#213487=CARTESIAN_POINT('Ctrl Pts',(-57.0597576325586,76.1552807409204,
73.4662010349383));
#213488=CARTESIAN_POINT('Ctrl Pts',(-57.0573264371889,76.1220824344896,
73.5465539116859));
#213489=CARTESIAN_POINT('Ctrl Pts',(-57.0548982484733,76.0878506663623,
73.6265113407856));
#213490=CARTESIAN_POINT('Ctrl Pts',(-57.0432786636594,75.9190847628144,
74.0072319048199));
#213491=CARTESIAN_POINT('Ctrl Pts',(-57.0341088716949,75.7711357874271,
74.3017986694038));
#213492=CARTESIAN_POINT('Ctrl Pts',(-56.9957885762682,75.0992476589838,
75.4927358238407));
#213493=CARTESIAN_POINT('Ctrl Pts',(-56.9660576349432,74.4548694757294,
76.3140514136448));
#213494=CARTESIAN_POINT('Ctrl Pts',(-56.9279130819348,73.4583336590304,
77.2497627599759));
#213495=CARTESIAN_POINT('Ctrl Pts',(-56.9187560496566,73.2077666176067,
77.4633042281827));
#213496=CARTESIAN_POINT('Ctrl Pts',(-56.8800484754342,72.1143958811979,
78.3077617050326));
#213497=CARTESIAN_POINT('Ctrl Pts',(-56.8499085692913,71.1872894119421,
78.8189818871622));
#213498=CARTESIAN_POINT('Ctrl Pts',(-56.811347805582,69.8891147015116,79.293159231546));
#213499=CARTESIAN_POINT('Ctrl Pts',(-56.8021738211618,69.5742688114049,
79.3912382909656));
#213500=CARTESIAN_POINT('Ctrl Pts',(-56.7639701171207,68.2547933773763,
79.7334530962459));
#213501=CARTESIAN_POINT('Ctrl Pts',(-56.7343632675314,67.2208270205417,
79.8401211356915));
#213502=CARTESIAN_POINT('Ctrl Pts',(-56.6963451969654,65.8599854096043,
79.774524049877));
#213503=CARTESIAN_POINT('Ctrl Pts',(-56.6871933048202,65.5324560266127,
79.7428906714159));
#213504=CARTESIAN_POINT('Ctrl Pts',(-56.6483561336814,64.1606193960235,
79.543408852849));
#213505=CARTESIAN_POINT('Ctrl Pts',(-56.618077292278,63.1440448474573,79.230242652439));
#213506=CARTESIAN_POINT('Ctrl Pts',(-56.5735389156253,61.708965591362,78.531221992244));
#213507=CARTESIAN_POINT('Ctrl Pts',(-56.5585384715947,61.2438784419826,
78.2574129661823));
#213508=CARTESIAN_POINT('Ctrl Pts',(-56.5206383555161,60.1447937104879,
77.4877590858182));
#213509=CARTESIAN_POINT('Ctrl Pts',(-56.4976849102169,59.5434899221976,
76.9515131398106));
#213510=CARTESIAN_POINT('Ctrl Pts',(-56.4633784313638,58.7282296931324,
76.031603029883));
#213511=CARTESIAN_POINT('Ctrl Pts',(-56.4515293700947,58.4656868142205,
75.6952695211716));
#213512=CARTESIAN_POINT('Ctrl Pts',(-56.4273567704757,57.9795111395256,
74.9853022222109));
#213513=CARTESIAN_POINT('Ctrl Pts',(-56.4150514704382,57.7571893384102,
74.6118084623104));
#213514=CARTESIAN_POINT('Ctrl Pts',(-56.4026978510105,57.5592258456979,
74.2253473780977));
#213515=CARTESIAN_POINT('Origin',(-45.8894114130409,66.6819786653733,69.5522455184007));
#213516=CARTESIAN_POINT('',(-59.2798347108578,76.1552807432749,73.4662010292395));
#213517=CARTESIAN_POINT('',(-58.8740778711611,76.1552807409204,73.4662010349383));
#213518=CARTESIAN_POINT('',(-45.8894114130409,76.1552807409204,73.4662010349383));
#213519=CARTESIAN_POINT('Ctrl Pts',(-57.4656305635332,76.1552807494603,
73.4662010142683));
#213520=CARTESIAN_POINT('Ctrl Pts',(-57.467015478482,76.1740038293382,73.4208838429784));
#213521=CARTESIAN_POINT('Ctrl Pts',(-57.4684018508168,76.1924045744336,
73.3754254530908));
#213522=CARTESIAN_POINT('Ctrl Pts',(-57.4791268110136,76.3321029248102,
73.0230530886952));
#213523=CARTESIAN_POINT('Ctrl Pts',(-57.4885180256257,76.4388381018525,
72.7105830796696));
#213524=CARTESIAN_POINT('Ctrl Pts',(-57.5234071649755,76.7789118976196,
71.5318265754218));
#213525=CARTESIAN_POINT('Ctrl Pts',(-57.548081462003,76.9133480225109,70.6412313736066));
#213526=CARTESIAN_POINT('Ctrl Pts',(-57.5888899472172,76.9405547933868,
69.1913898745211));
#213527=CARTESIAN_POINT('Ctrl Pts',(-57.6046512409984,76.9061305640136,
68.6382920006278));
#213528=CARTESIAN_POINT('Ctrl Pts',(-57.6381300269269,76.7379961738035,
67.471202685675));
#213529=CARTESIAN_POINT('Ctrl Pts',(-57.6554659860436,76.5921995880529,
66.8611953949494));
#213530=CARTESIAN_POINT('Ctrl Pts',(-57.6912072352798,76.1826351896035,
65.650227797998));
#213531=CARTESIAN_POINT('Ctrl Pts',(-57.7096703604995,75.9150563337205,
65.0535258809456));
#213532=CARTESIAN_POINT('Ctrl Pts',(-57.7592658898742,75.0532745094317,
63.5377100374715));
#213533=CARTESIAN_POINT('Ctrl Pts',(-57.7891281575416,74.365922388328,62.6812739258004));
#213534=CARTESIAN_POINT('Ctrl Pts',(-57.8362286934362,73.1324183228756,
61.5659286972865));
#213535=CARTESIAN_POINT('Ctrl Pts',(-57.8525941770464,72.6769632259057,
61.2186032224233));
#213536=CARTESIAN_POINT('Ctrl Pts',(-57.8830343509336,71.7633527920207,
60.6357324287105));
#213537=CARTESIAN_POINT('Ctrl Pts',(-57.8972020711146,71.3117553325347,
60.3931112262922));
#213538=CARTESIAN_POINT('Ctrl Pts',(-57.9294173302583,70.2613766767877,
59.9264068332462));
#213539=CARTESIAN_POINT('Ctrl Pts',(-57.9475315653734,69.6559529717776,
59.7224783141321));
#213540=CARTESIAN_POINT('Ctrl Pts',(-57.9835838838913,68.4210159102935,
59.4311340719715));
#213541=CARTESIAN_POINT('Ctrl Pts',(-58.0011045049236,67.7944202696037,
59.3432482785523));
#213542=CARTESIAN_POINT('Ctrl Pts',(-58.037078420087,66.508443372804,59.2827403411216));
#213543=CARTESIAN_POINT('Ctrl Pts',(-58.0556185294718,65.8517130605504,
59.314887703157));
#213544=CARTESIAN_POINT('Ctrl Pts',(-58.1127259894106,63.8652087101706,
59.6046365097492));
#213545=CARTESIAN_POINT('Ctrl Pts',(-58.1496465648698,62.5795290112645,
60.0623024095847));
#213546=CARTESIAN_POINT('Ctrl Pts',(-58.2140602109587,60.6364591286289,
61.2247457994848));
#213547=CARTESIAN_POINT('Ctrl Pts',(-58.239261910165,59.9192867258378,61.7958566469786));
#213548=CARTESIAN_POINT('Ctrl Pts',(-58.2892121356522,58.6881528212927,
63.0784745967642));
#213549=CARTESIAN_POINT('Ctrl Pts',(-58.3140360354789,58.1704875432274,
63.7759588221726));
#213550=CARTESIAN_POINT('Ctrl Pts',(-58.3571375745576,57.4158586407829,
65.1186017190906));
#213551=CARTESIAN_POINT('Ctrl Pts',(-58.3758307916097,57.1440556581665,
65.7382969422851));
#213552=CARTESIAN_POINT('Ctrl Pts',(-58.413283526736,56.7340904429182,66.9980073249814));
#213553=CARTESIAN_POINT('Ctrl Pts',(-58.431897657372,56.5922226913977,67.6335361595996));
#213554=CARTESIAN_POINT('Ctrl Pts',(-58.4641721348272,56.4492006941421,
68.7752647657879));
#213555=CARTESIAN_POINT('Ctrl Pts',(-58.4780448026808,56.4234574692962,
69.2762201526426));
#213556=CARTESIAN_POINT('Ctrl Pts',(-58.501263199602,56.4416173325673,70.1040382693353));
#213557=CARTESIAN_POINT('Ctrl Pts',(-58.5104876105461,56.4644375849527,
70.4304981763454));
#213558=CARTESIAN_POINT('Ctrl Pts',(-58.5334900665772,56.5596121598773,
71.2357751792123));
#213559=CARTESIAN_POINT('Ctrl Pts',(-58.5473187248335,56.6503451183651,
71.7116215901185));
#213560=CARTESIAN_POINT('Ctrl Pts',(-58.5745365302001,56.8981014858657,
72.6460147409833));
#213561=CARTESIAN_POINT('Ctrl Pts',(-58.5879052191749,57.0546854938996,
73.10342730167));
#213562=CARTESIAN_POINT('Ctrl Pts',(-58.618885913421,57.4864607270938,74.1233723398853));
#213563=CARTESIAN_POINT('Ctrl Pts',(-58.636565387954,57.7820738379356,74.6751774283459));
#213564=CARTESIAN_POINT('Ctrl Pts',(-58.6927354152295,58.869456319419,76.3234632986077));
#213565=CARTESIAN_POINT('Ctrl Pts',(-58.7296145133947,59.8281828204287,
77.2924245069557));
#213566=CARTESIAN_POINT('Ctrl Pts',(-58.8064690912451,62.0673178743056,
78.803961807114));
#213567=CARTESIAN_POINT('Ctrl Pts',(-58.8433913930995,63.3261654160311,
79.3311957990547));
#213568=CARTESIAN_POINT('Ctrl Pts',(-58.8912730138153,64.9759640755396,
79.6647104567306));
#213569=CARTESIAN_POINT('Ctrl Pts',(-58.9007099114221,65.3039499037962,
79.714601179347));
#213570=CARTESIAN_POINT('Ctrl Pts',(-58.9246479319593,66.1507039200396,
79.8016496087106));
#213571=CARTESIAN_POINT('Ctrl Pts',(-58.9390230634061,66.6709254233852,
79.8154039115158));
#213572=CARTESIAN_POINT('Ctrl Pts',(-58.9830883241446,68.2417342164512,
79.7374628040431));
#213573=CARTESIAN_POINT('Ctrl Pts',(-59.0132451353013,69.2792255166301,
79.5234944200773));
#213574=CARTESIAN_POINT('Ctrl Pts',(-59.0518229434675,70.5746421187004,
79.040043347047));
#213575=CARTESIAN_POINT('Ctrl Pts',(-59.0609975786872,70.8776998603756,
78.9099727849275));
#213576=CARTESIAN_POINT('Ctrl Pts',(-59.0991745161019,72.1020906034945,
78.3130146834841));
#213577=CARTESIAN_POINT('Ctrl Pts',(-59.1287536205988,72.9565327629299,
77.7228433579753));
#213578=CARTESIAN_POINT('Ctrl Pts',(-59.1667441086041,73.9477299291393,
76.7896127231644));
#213579=CARTESIAN_POINT('Ctrl Pts',(-59.1758949855277,74.1761531570951,
76.552815053904));
#213580=CARTESIAN_POINT('Ctrl Pts',(-59.2147979782659,75.0910456081536,
75.5081892252033));
#213581=CARTESIAN_POINT('Ctrl Pts',(-59.2451433370461,75.6614373004834,
74.6074410484701));
#213582=CARTESIAN_POINT('Ctrl Pts',(-59.2764194054209,76.1080083511556,
73.5791817217942));
#213583=CARTESIAN_POINT('Ctrl Pts',(-59.2781271442582,76.1318989104646,
73.5227942033599));
#213584=CARTESIAN_POINT('Ctrl Pts',(-59.2798347108578,76.1552807456294,
73.4662010235407));
#213585=CARTESIAN_POINT('Ctrl Pts',(-58.8740778711611,76.1552807409204,
73.4662010349383));
#213586=CARTESIAN_POINT('Ctrl Pts',(-58.8654806787207,76.0383768587021,
73.7491541204752));
#213587=CARTESIAN_POINT('Ctrl Pts',(-58.8568298367276,75.90878836642,74.0268879792384));
#213588=CARTESIAN_POINT('Ctrl Pts',(-58.8302237446842,75.4747103220283,
74.8577554124336));
#213589=CARTESIAN_POINT('Ctrl Pts',(-58.8122496817308,75.1315460085142,
75.388802228158));
#213590=CARTESIAN_POINT('Ctrl Pts',(-58.7768679551842,74.3488587311254,
76.3849487576114));
#213591=CARTESIAN_POINT('Ctrl Pts',(-58.7592049358076,73.9102993558927,
76.8473302188392));
#213592=CARTESIAN_POINT('Ctrl Pts',(-58.7269131362887,73.0513189722705,
77.5989542394252));
#213593=CARTESIAN_POINT('Ctrl Pts',(-58.7124707373962,72.646803865238,77.9032259682973));
#213594=CARTESIAN_POINT('Ctrl Pts',(-58.6807977859588,71.7043343448384,
78.5085980765727));
#213595=CARTESIAN_POINT('Ctrl Pts',(-58.6638417719715,71.1583389362967,
78.793593297296));
#213596=CARTESIAN_POINT('Ctrl Pts',(-58.6276988074985,69.9663460640599,
79.2852149710834));
#213597=CARTESIAN_POINT('Ctrl Pts',(-58.6084968950721,69.3187055868823,
79.4802573030972));
#213598=CARTESIAN_POINT('Ctrl Pts',(-58.5600660604257,67.6442285837402,
79.8090006783218));
#213599=CARTESIAN_POINT('Ctrl Pts',(-58.5318568413971,66.6076070209451,
79.853770689239));
#213600=CARTESIAN_POINT('Ctrl Pts',(-58.4853315968718,64.9767548724265,
79.6777139821547));
#213601=CARTESIAN_POINT('Ctrl Pts',(-58.4679512565759,64.3786780257699,
79.5586295355342));
#213602=CARTESIAN_POINT('Ctrl Pts',(-58.4380529585056,63.3530690024533,
79.2575385648589));
#213603=CARTESIAN_POINT('Ctrl Pts',(-58.4252826161563,62.9206670011429,
79.0982859507564));
#213604=CARTESIAN_POINT('Ctrl Pts',(-58.3934258607863,61.8841174279368,
78.6351257548048));
#213605=CARTESIAN_POINT('Ctrl Pts',(-58.3741846239427,61.2965120122271,
78.299526150952));
#213606=CARTESIAN_POINT('Ctrl Pts',(-58.331302717783,60.0633423854162,77.4235669864371));
#213607=CARTESIAN_POINT('Ctrl Pts',(-58.3083255357522,59.442522328844,76.8566497643465));
#213608=CARTESIAN_POINT('Ctrl Pts',(-58.2592759945427,58.3112313678633,
75.5360167756007));
#213609=CARTESIAN_POINT('Ctrl Pts',(-58.2335467836475,57.817687165605,74.7771172273428));
#213610=CARTESIAN_POINT('Ctrl Pts',(-58.1901612235394,57.1482227094101,
73.3729767633361));
#213611=CARTESIAN_POINT('Ctrl Pts',(-58.1719011545338,56.923856123056,72.7568556656188));
#213612=CARTESIAN_POINT('Ctrl Pts',(-58.1354437498611,56.6015724733037,
71.5132272243054));
#213613=CARTESIAN_POINT('Ctrl Pts',(-58.1174736775659,56.5000540132254,
70.8895808585808));
#213614=CARTESIAN_POINT('Ctrl Pts',(-58.0823674528289,56.4132050083097,
69.6358101939047));
#213615=CARTESIAN_POINT('Ctrl Pts',(-58.0649788425391,56.4272759715382,
69.0084018077861));
#213616=CARTESIAN_POINT('Ctrl Pts',(-58.0333067844926,56.554698426862,67.8955662288894));
#213617=CARTESIAN_POINT('Ctrl Pts',(-58.0192056868718,56.6462646928936,
67.4096225844261));
#213618=CARTESIAN_POINT('Ctrl Pts',(-57.9849711817108,56.9553018835286,
66.2407983865155));
#213619=CARTESIAN_POINT('Ctrl Pts',(-57.9652950581261,57.2099560940189,
65.5704477543328));
#213620=CARTESIAN_POINT('Ctrl Pts',(-57.9262115605762,57.83679855784,64.3290633884311));
#213621=CARTESIAN_POINT('Ctrl Pts',(-57.906915621022,58.200157196157,63.7576331955304));
#213622=CARTESIAN_POINT('Ctrl Pts',(-57.8695297520541,59.0157679561456,
62.7178464370234));
#213623=CARTESIAN_POINT('Ctrl Pts',(-57.8517243389694,59.4616146862542,
62.2484010846137));
#213624=CARTESIAN_POINT('Ctrl Pts',(-57.8073541786503,60.654170304857,61.2093691844293));
#213625=CARTESIAN_POINT('Ctrl Pts',(-57.7805104802939,61.4405265081503,
60.694184432741));
#213626=CARTESIAN_POINT('Ctrl Pts',(-57.7400124097595,62.749174302271,60.0728650906821));
#213627=CARTESIAN_POINT('Ctrl Pts',(-57.7257819053405,63.2283970108871,
59.8879619274299));
#213628=CARTESIAN_POINT('Ctrl Pts',(-57.6923337372342,64.3667012515537,
59.5442925133128));
#213629=CARTESIAN_POINT('Ctrl Pts',(-57.6729996626182,65.0317028118234,
59.4133990380026));
#213630=CARTESIAN_POINT('Ctrl Pts',(-57.6378936609327,66.2687727896728,
59.2949151779632));
#213631=CARTESIAN_POINT('Ctrl Pts',(-57.6222427104545,66.8363256955812,
59.2877560179656));
#213632=CARTESIAN_POINT('Ctrl Pts',(-57.5755586861321,68.4994021601375,
59.4047971992212));
#213633=CARTESIAN_POINT('Ctrl Pts',(-57.5440731569583,69.5776699381353,
59.6583730909056));
#213634=CARTESIAN_POINT('Ctrl Pts',(-57.4951466382518,71.1990127732355,
60.3280309135308));
#213635=CARTESIAN_POINT('Ctrl Pts',(-57.4769062785586,71.7778865356518,
60.6347656474687));
#213636=CARTESIAN_POINT('Ctrl Pts',(-57.4404755134304,72.8498076454491,
61.3414219801888));
#213637=CARTESIAN_POINT('Ctrl Pts',(-57.4225074259785,73.3429084055756,
61.7361231035919));
#213638=CARTESIAN_POINT('Ctrl Pts',(-57.3879561490331,74.2332210615537,
62.5945827351945));
#213639=CARTESIAN_POINT('Ctrl Pts',(-57.3711201580598,74.6315892901806,
63.0534746806907));
#213640=CARTESIAN_POINT('Ctrl Pts',(-57.340421131451,75.2684352083772,63.9339023404445));
#213641=CARTESIAN_POINT('Ctrl Pts',(-57.3267248928043,75.5221454235618,
64.3422105789097));
#213642=CARTESIAN_POINT('Ctrl Pts',(-57.2874445637386,76.1687356212143,
65.5669425758004));
#213643=CARTESIAN_POINT('Ctrl Pts',(-57.2626574740573,76.4833659815526,
66.4195142259108));
#213644=CARTESIAN_POINT('Ctrl Pts',(-57.2233290994146,76.788802993578,67.7770247493286));
#213645=CARTESIAN_POINT('Ctrl Pts',(-57.2094406741909,76.8616773711026,
68.2587859908722));
#213646=CARTESIAN_POINT('Ctrl Pts',(-57.1729484303027,76.9632227952369,
69.5423857028234));
#213647=CARTESIAN_POINT('Ctrl Pts',(-57.1509568701997,76.932577635555,70.3455300793908));
#213648=CARTESIAN_POINT('Ctrl Pts',(-57.1055800295041,76.6835918978208,
71.9366919129624));
#213649=CARTESIAN_POINT('Ctrl Pts',(-57.0823786178288,76.4641733992887,
72.7185600744632));
#213650=CARTESIAN_POINT('Ctrl Pts',(-57.0597576325586,76.1552807409204,
73.4662010349383));
#213651=CARTESIAN_POINT('Origin',(-45.8894114130409,66.6819786653733,69.5522455184007));
#213652=CARTESIAN_POINT('',(-61.0939133588288,76.1552807409204,73.4662010349383));
#213653=CARTESIAN_POINT('',(-60.6878802914039,76.1552807419561,73.4662010324316));
#213654=CARTESIAN_POINT('',(-45.8894114130409,76.1552807409204,73.4662010349383));
#213655=CARTESIAN_POINT('Ctrl Pts',(-59.2798347108578,76.1552807456294,
73.4662010235407));
#213656=CARTESIAN_POINT('Ctrl Pts',(-59.2873239377944,76.2578312814522,
73.2179886452789));
#213657=CARTESIAN_POINT('Ctrl Pts',(-59.2948125599407,76.3505958902946,
72.9658202019355));
#213658=CARTESIAN_POINT('Ctrl Pts',(-59.3212550248658,76.6412408841389,
72.0683661022729));
#213659=CARTESIAN_POINT('Ctrl Pts',(-59.3404565657508,76.7852352409474,
71.4074966004155));
#213660=CARTESIAN_POINT('Ctrl Pts',(-59.3889800804819,76.9829003351291,
69.7092774286031));
#213661=CARTESIAN_POINT('Ctrl Pts',(-59.4172768981262,76.9461688502664,
68.6690429788179));
#213662=CARTESIAN_POINT('Ctrl Pts',(-59.4640581665987,76.6404227144672,
67.0484062161532));
#213663=CARTESIAN_POINT('Ctrl Pts',(-59.4815942391593,76.4725145859891,
66.4562414461179));
#213664=CARTESIAN_POINT('Ctrl Pts',(-59.5124154203648,76.0779084293696,
65.4270660907031));
#213665=CARTESIAN_POINT('Ctrl Pts',(-59.5259528021725,75.8709055245387,
64.9845081081328));
#213666=CARTESIAN_POINT('Ctrl Pts',(-59.5586389464261,75.3041133707561,
63.9685683013047));
#213667=CARTESIAN_POINT('Ctrl Pts',(-59.5779246567413,74.9175650253119,
63.4127211099847));
#213668=CARTESIAN_POINT('Ctrl Pts',(-59.6160754061338,74.0425641561455,
62.3872807913945));
#213669=CARTESIAN_POINT('Ctrl Pts',(-59.6346024318829,73.5566506811219,
61.9198261856102));
#213670=CARTESIAN_POINT('Ctrl Pts',(-59.6724351197661,72.4983354380824,
61.0853544833108));
#213671=CARTESIAN_POINT('Ctrl Pts',(-59.6916891483082,71.9282138895974,
60.7207535829762));
#213672=CARTESIAN_POINT('Ctrl Pts',(-59.7328542569981,70.6331193165802,
60.0624708439655));
#213673=CARTESIAN_POINT('Ctrl Pts',(-59.7542186705655,69.9019725341391,
59.7901260313104));
#213674=CARTESIAN_POINT('Ctrl Pts',(-59.7951715089607,68.4901351827486,
59.4403144874627));
#213675=CARTESIAN_POINT('Ctrl Pts',(-59.8145446091965,67.8186828647086,
59.3430110164237));
#213676=CARTESIAN_POINT('Ctrl Pts',(-59.8478622232024,66.6385684477296,
59.2899291105759));
#213677=CARTESIAN_POINT('Ctrl Pts',(-59.8618209806189,66.1335879871315,
59.304499705822));
#213678=CARTESIAN_POINT('Ctrl Pts',(-59.8935251446396,65.0060535038607,
59.4206410901775));
#213679=CARTESIAN_POINT('Ctrl Pts',(-59.9113264579511,64.3876333714385,
59.5425452453374));
#213680=CARTESIAN_POINT('Ctrl Pts',(-59.967609771616,62.4896831880558,60.1019125225695));
#213681=CARTESIAN_POINT('Ctrl Pts',(-60.0044817633918,61.2830797298608,
60.7354424055245));
#213682=CARTESIAN_POINT('Ctrl Pts',(-60.0813271442445,59.1832849088952,
62.4347426735237));
#213683=CARTESIAN_POINT('Ctrl Pts',(-60.1182483120269,58.3111222160689,
63.4844601762531));
#213684=CARTESIAN_POINT('Ctrl Pts',(-60.1661319992958,57.5098768998731,
64.9647575329513));
#213685=CARTESIAN_POINT('Ctrl Pts',(-60.175570853064,57.3662509499148,65.2639221863736));
#213686=CARTESIAN_POINT('Ctrl Pts',(-60.1996436772939,57.0335944489885,
66.0527814412899));
#213687=CARTESIAN_POINT('Ctrl Pts',(-60.2141508145759,56.8671983647576,
66.5509691579901));
#213688=CARTESIAN_POINT('Ctrl Pts',(-60.2579230862595,56.4873765134373,
68.0660100749166));
#213689=CARTESIAN_POINT('Ctrl Pts',(-60.2876399944278,56.3893297683789,
69.1048132112122));
#213690=CARTESIAN_POINT('Ctrl Pts',(-60.3257703432487,56.4677601315748,
70.4690258915158));
#213691=CARTESIAN_POINT('Ctrl Pts',(-60.3349268208386,56.5024479063959,
70.7963916758307));
#213692=CARTESIAN_POINT('Ctrl Pts',(-60.3736532148053,56.7140616379533,
72.162289314325));
#213693=CARTESIAN_POINT('Ctrl Pts',(-60.4038128271924,57.0347519115952,
73.1720137110355));
#213694=CARTESIAN_POINT('Ctrl Pts',(-60.4423934893387,57.6503102991411,
74.4102394881232));
#213695=CARTESIAN_POINT('Ctrl Pts',(-60.4515682410964,57.8111861304835,
74.6981349684982));
#213696=CARTESIAN_POINT('Ctrl Pts',(-60.4897417630452,58.5321412935251,
75.8537195879102));
#213697=CARTESIAN_POINT('Ctrl Pts',(-60.5193172463587,59.2078496718595,
76.6420853490512));
#213698=CARTESIAN_POINT('Ctrl Pts',(-60.5573040612076,60.2389420037159,
77.5308356752901));
#213699=CARTESIAN_POINT('Ctrl Pts',(-60.5664547917166,60.4981936958185,
77.7334083585058));
#213700=CARTESIAN_POINT('Ctrl Pts',(-60.6053624474569,61.6323858776986,
78.5348762542881));
#213701=CARTESIAN_POINT('Ctrl Pts',(-60.6357127054609,62.5877081838141,
79.0086189465251));
#213702=CARTESIAN_POINT('Ctrl Pts',(-60.674487735492,63.9131697130843,79.4267077905138));
#213703=CARTESIAN_POINT('Ctrl Pts',(-60.6836704322661,64.2323578677275,
79.5106924671336));
#213704=CARTESIAN_POINT('Ctrl Pts',(-60.7118298660933,65.21508558333,79.7191521568226));
#213705=CARTESIAN_POINT('Ctrl Pts',(-60.7310315029189,65.8873448685828,
79.7936470979331));
#213706=CARTESIAN_POINT('Ctrl Pts',(-60.7795309967203,67.5960717486121,
79.8136461475118));
#213707=CARTESIAN_POINT('Ctrl Pts',(-60.8078051086568,68.6260197611533,
79.6691923839409));
#213708=CARTESIAN_POINT('Ctrl Pts',(-60.85451944694,70.2039656251719,79.1976383421178));
#213709=CARTESIAN_POINT('Ctrl Pts',(-60.8720146380996,70.7741772355134,
78.969884356699));
#213710=CARTESIAN_POINT('Ctrl Pts',(-60.9025867168087,71.7490578343482,
78.4751395451311));
#213711=CARTESIAN_POINT('Ctrl Pts',(-60.9159159079656,72.1616733403399,
78.2278593814121));
#213712=CARTESIAN_POINT('Ctrl Pts',(-60.9483752296809,73.1088119638081,
77.5656261636239));
#213713=CARTESIAN_POINT('Ctrl Pts',(-60.9676476524271,73.6226153704897,
77.1249598270608));
#213714=CARTESIAN_POINT('Ctrl Pts',(-61.0069126057781,74.5810939893403,
76.1228360744059));
#213715=CARTESIAN_POINT('Ctrl Pts',(-61.026489504624,75.0179865180214,75.5588800128241));
#213716=CARTESIAN_POINT('Ctrl Pts',(-61.0621754880272,75.6872603427455,
74.4796447268075));
#213717=CARTESIAN_POINT('Ctrl Pts',(-61.0780551106555,75.9421911667023,
73.9819610882114));
#213718=CARTESIAN_POINT('Ctrl Pts',(-61.0939133588288,76.1552807409204,
73.4662010349383));
#213719=CARTESIAN_POINT('Ctrl Pts',(-60.6878802914039,76.1552807429917,
73.4662010299249));
#213720=CARTESIAN_POINT('Ctrl Pts',(-60.6549485341108,75.7132504877363,
74.5360870118048));
#213721=CARTESIAN_POINT('Ctrl Pts',(-60.6232629579733,75.0931226335129,
75.5234705721753));
#213722=CARTESIAN_POINT('Ctrl Pts',(-60.5753209784772,73.965374356376,76.7840831573706));
#213723=CARTESIAN_POINT('Ctrl Pts',(-60.5600539347455,73.5790171038901,
77.1534423333565));
#213724=CARTESIAN_POINT('Ctrl Pts',(-60.5260316711703,72.6417442432974,
77.9189216694829));
#213725=CARTESIAN_POINT('Ctrl Pts',(-60.5073738169853,72.0767549475306,
78.2938972018152));
#213726=CARTESIAN_POINT('Ctrl Pts',(-60.4735852252674,71.0172501247381,
78.8549804079524));
#213727=CARTESIAN_POINT('Ctrl Pts',(-60.4586939776463,70.537527052056,79.0638277026571));
#213728=CARTESIAN_POINT('Ctrl Pts',(-60.4262453781121,69.4576424072261,
79.43877344229));
#213729=CARTESIAN_POINT('Ctrl Pts',(-60.409058418936,68.8540231352694,79.5886775647626));
#213730=CARTESIAN_POINT('Ctrl Pts',(-60.3734714870408,67.5960713455299,
79.7822078911068));
#213731=CARTESIAN_POINT('Ctrl Pts',(-60.355017215576,66.9435951390965,79.8196325924058));
#213732=CARTESIAN_POINT('Ctrl Pts',(-60.3055240992358,65.2047612307084,
79.7534292233736));
#213733=CARTESIAN_POINT('Ctrl Pts',(-60.2757486247089,64.1310079803187,
79.5391809452647));
#213734=CARTESIAN_POINT('Ctrl Pts',(-60.2286892275576,62.5735019927232,
78.9603211407063));
#213735=CARTESIAN_POINT('Ctrl Pts',(-60.2122723783564,62.0535931967266,
78.7157340010946));
#213736=CARTESIAN_POINT('Ctrl Pts',(-60.181791493639,61.1137897171559,78.1731239029127));
#213737=CARTESIAN_POINT('Ctrl Pts',(-60.1676315602797,60.6904769236396,
77.8844831172379));
#213738=CARTESIAN_POINT('Ctrl Pts',(-60.1329740426831,59.7237980888031,
77.1134404341653));
#213739=CARTESIAN_POINT('Ctrl Pts',(-60.1123084476268,59.2066537291693,
76.6025959714561));
#213740=CARTESIAN_POINT('Ctrl Pts',(-60.082295326596,58.5358905214297,75.7824723433042));
#213741=CARTESIAN_POINT('Ctrl Pts',(-60.0729376397816,58.3368489241872,
75.5132260455352));
#213742=CARTESIAN_POINT('Ctrl Pts',(-60.0454258533623,57.7900555909077,
74.6923694873538));
#213743=CARTESIAN_POINT('Ctrl Pts',(-60.0272520902436,57.4813255399839,
74.1167986352783));
#213744=CARTESIAN_POINT('Ctrl Pts',(-59.9952901842338,57.0456129228912,
73.0776794715103));
#213745=CARTESIAN_POINT('Ctrl Pts',(-59.9817127483809,56.892578447159,72.6272857226267));
#213746=CARTESIAN_POINT('Ctrl Pts',(-59.9549264327128,56.6499902430636,
71.708128035941));
#213747=CARTESIAN_POINT('Ctrl Pts',(-59.9417584347214,56.5607852278596,
71.2404603787749));
#213748=CARTESIAN_POINT('Ctrl Pts',(-59.9191599910854,56.4648900413591,
70.4378726483234));
#213749=CARTESIAN_POINT('Ctrl Pts',(-59.9098138709983,56.441525080417,70.1057288119717));
#213750=CARTESIAN_POINT('Ctrl Pts',(-59.8862018942639,56.4235443216733,
69.2711961468919));
#213751=CARTESIAN_POINT('Ctrl Pts',(-59.8718628566535,56.4496103948148,
68.7692382534012));
#213752=CARTESIAN_POINT('Ctrl Pts',(-59.839516880951,56.5925153240701,67.6347664157159));
#213753=CARTESIAN_POINT('Ctrl Pts',(-59.8218335602107,56.7322556075732,
67.007248505875));
#213754=CARTESIAN_POINT('Ctrl Pts',(-59.7773523524945,57.220434708535,65.4984210150842));
#213755=CARTESIAN_POINT('Ctrl Pts',(-59.7502626452442,57.633921297722,64.6443974106474));
#213756=CARTESIAN_POINT('Ctrl Pts',(-59.7089452485514,58.4549724285869,
63.4151545489328));
#213757=CARTESIAN_POINT('Ctrl Pts',(-59.6941331228875,58.7857298103031,
62.9950532064511));
#213758=CARTESIAN_POINT('Ctrl Pts',(-59.6600401087609,59.6066435074168,
62.1050767582944));
#213759=CARTESIAN_POINT('Ctrl Pts',(-59.6406626778559,60.1137418848491,
61.6542114447438));
#213760=CARTESIAN_POINT('Ctrl Pts',(-59.6075214539254,61.0649230001214,
60.963906100831));
#213761=CARTESIAN_POINT('Ctrl Pts',(-59.5937295363409,61.4890949026599,
60.700982854176));
#213762=CARTESIAN_POINT('Ctrl Pts',(-59.5619836481202,62.4948812706617,
60.1748196345405));
#213763=CARTESIAN_POINT('Ctrl Pts',(-59.5439632172434,63.0853266098694,
59.9328910318027));
#213764=CARTESIAN_POINT('Ctrl Pts',(-59.5163445957165,64.0141391665109,
59.6498785787787));
#213765=CARTESIAN_POINT('Ctrl Pts',(-59.5068630287181,64.3384759567163,
59.5681462490696));
#213766=CARTESIAN_POINT('Ctrl Pts',(-59.4781411725836,65.3433315880202,
59.366596917901));
#213767=CARTESIAN_POINT('Ctrl Pts',(-59.4590485401284,66.0324285189169,
59.299562823386));
#213768=CARTESIAN_POINT('Ctrl Pts',(-59.4259185778911,67.2049256704212,
59.3042570477717));
#213769=CARTESIAN_POINT('Ctrl Pts',(-59.4121692654834,67.6860998487761,
59.3401703957783));
#213770=CARTESIAN_POINT('Ctrl Pts',(-59.3737534033847,69.0266224411124,
59.5359101890221));
#213771=CARTESIAN_POINT('Ctrl Pts',(-59.3498274925003,69.8706508586717,
59.7718212381078));
#213772=CARTESIAN_POINT('Ctrl Pts',(-59.299281691461,71.5193218358627,60.4690792530385));
#213773=CARTESIAN_POINT('Ctrl Pts',(-59.2731736187973,72.3123426922754,
60.9381397042643));
#213774=CARTESIAN_POINT('Ctrl Pts',(-59.2099049123124,74.0932680633157,
62.3437747327888));
#213775=CARTESIAN_POINT('Ctrl Pts',(-59.1714264730219,74.9781754503829,
63.3827736498539));
#213776=CARTESIAN_POINT('Ctrl Pts',(-59.1153877058776,75.9562112306616,
65.1381831109986));
#213777=CARTESIAN_POINT('Ctrl Pts',(-59.0969999679401,76.2203414750931,
65.7423948469949));
#213778=CARTESIAN_POINT('Ctrl Pts',(-59.0603571616319,76.6212706720565,
66.9690058615184));
#213779=CARTESIAN_POINT('Ctrl Pts',(-59.0423634308292,76.7617220829095,
67.5871901044692));
#213780=CARTESIAN_POINT('Ctrl Pts',(-59.0155634669358,76.8870309466762,
68.5390172346081));
#213781=CARTESIAN_POINT('Ctrl Pts',(-59.0064538859771,76.9141896502028,
68.865527374132));
#213782=CARTESIAN_POINT('Ctrl Pts',(-58.966135792939,76.9646919211623,70.304674835983));
#213783=CARTESIAN_POINT('Ctrl Pts',(-58.9343155956169,76.8224161565893,
71.4155415775799));
#213784=CARTESIAN_POINT('Ctrl Pts',(-58.8935634996675,76.4048021503051,
72.8157919687679));
#213785=CARTESIAN_POINT('Ctrl Pts',(-58.8838562479809,76.2882462665789,
73.1443724947634));
#213786=CARTESIAN_POINT('Ctrl Pts',(-58.8740778711611,76.1552807409204,
73.4662010349383));
#213787=CARTESIAN_POINT('Origin',(-45.8894114130409,66.6819786653733,69.5522455184007));
#213788=CARTESIAN_POINT('',(-62.9075068658247,76.1552807409205,73.4662010349382));
#213789=CARTESIAN_POINT('',(-62.5017927896903,76.155280734099,73.4662010514488));
#213790=CARTESIAN_POINT('',(-45.8894114130409,76.1552807409204,73.4662010349383));
#213791=CARTESIAN_POINT('',(-62.1255457361908,56.4404739457998,69.970346603214));
#213792=CARTESIAN_POINT('Ctrl Pts',(-62.9075068658247,76.1552807409205,
73.4662010349381));
#213793=CARTESIAN_POINT('Ctrl Pts',(-62.8890297137549,75.9058901354936,
74.0698237715866));
#213794=CARTESIAN_POINT('Ctrl Pts',(-62.8709501951456,75.5993777230872,
74.6482296293145));
#213795=CARTESIAN_POINT('Ctrl Pts',(-62.8346556323582,74.8824994691326,
75.7357486846771));
#213796=CARTESIAN_POINT('Ctrl Pts',(-62.816127299745,74.4743566483045,76.2427667065411));
#213797=CARTESIAN_POINT('Ctrl Pts',(-62.7595831183316,73.087620491147,77.6650712602951));
#213798=CARTESIAN_POINT('Ctrl Pts',(-62.7232980830353,71.975875999061,78.4305795136537));
#213799=CARTESIAN_POINT('Ctrl Pts',(-62.6471481891127,69.5250490757961,
79.4898561694311));
#213800=CARTESIAN_POINT('Ctrl Pts',(-62.6109576119547,68.2100385426075,
79.7749756124774));
#213801=CARTESIAN_POINT('Ctrl Pts',(-62.5541063933798,66.212220750335,79.8130641293939));
#213802=CARTESIAN_POINT('Ctrl Pts',(-62.535111901963,65.5474139902432,79.760960059608));
#213803=CARTESIAN_POINT('Ctrl Pts',(-62.4978581696945,64.2397658569823,
79.5290869291397));
#213804=CARTESIAN_POINT('Ctrl Pts',(-62.4796746883654,63.5999399229083,
79.3503470402618));
#213805=CARTESIAN_POINT('Ctrl Pts',(-62.4424295539205,62.3682979709726,
78.8735937106281));
#213806=CARTESIAN_POINT('Ctrl Pts',(-62.4235188596298,61.7790196920629,
78.5775642584995));
#213807=CARTESIAN_POINT('Ctrl Pts',(-62.3861515017278,60.6593754335759,
77.8728813615583));
#213808=CARTESIAN_POINT('Ctrl Pts',(-62.367792036736,60.1323725892804,77.4647286706259));
#213809=CARTESIAN_POINT('Ctrl Pts',(-62.3306363167817,59.1642311111784,
76.5514880424947));
#213810=CARTESIAN_POINT('Ctrl Pts',(-62.3115449033513,58.7255184123369,
76.0484475302655));
#213811=CARTESIAN_POINT('Ctrl Pts',(-62.2644735866284,57.763231000053,74.7000482335411));
#213812=CARTESIAN_POINT('Ctrl Pts',(-62.237467135121,57.3076947730774,73.8144878831635));
#213813=CARTESIAN_POINT('Ctrl Pts',(-62.1815044190819,56.6647956602292,
71.9398912558015));
#213814=CARTESIAN_POINT('Ctrl Pts',(-62.1531555603416,56.4809386499188,
70.9606701984124));
#213815=CARTESIAN_POINT('Ctrl Pts',(-62.1255316836823,56.4405094161815,
69.9703455277974));
#213816=CARTESIAN_POINT('Ctrl Pts',(-61.0939133588288,76.1552807409204,
73.4662010349383));
#213817=CARTESIAN_POINT('Ctrl Pts',(-61.0972367439251,76.1999375471068,
73.3581141103563));
#213818=CARTESIAN_POINT('Ctrl Pts',(-61.1005568733328,76.2427567690946,
73.2492332337271));
#213819=CARTESIAN_POINT('Ctrl Pts',(-61.1224307548111,76.5133223357398,
72.5250515977391));
#213820=CARTESIAN_POINT('Ctrl Pts',(-61.1405086451475,76.6833975931833,
71.8898758938489));
#213821=CARTESIAN_POINT('Ctrl Pts',(-61.1778581615379,76.9029391447842,
70.5770148905306));
#213822=CARTESIAN_POINT('Ctrl Pts',(-61.1970990172255,76.9482316221127,
69.9018442930587));
#213823=CARTESIAN_POINT('Ctrl Pts',(-61.2400395265103,76.9001918497218,
68.3879451290524));
#213824=CARTESIAN_POINT('Ctrl Pts',(-61.2630717386202,76.7705483014273,
67.5551875938367));
#213825=CARTESIAN_POINT('Ctrl Pts',(-61.312198681151,76.2940135131976,65.880082552741));
#213826=CARTESIAN_POINT('Ctrl Pts',(-61.3379412428464,75.9337910039552,
65.0489153455686));
#213827=CARTESIAN_POINT('Ctrl Pts',(-61.3813544223569,75.1324778699189,
63.7144282365011));
#213828=CARTESIAN_POINT('Ctrl Pts',(-61.3996290326739,74.742489401471,63.186775714214));
#213829=CARTESIAN_POINT('Ctrl Pts',(-61.4361064185458,73.8832261135128,
62.2308855240864));
#213830=CARTESIAN_POINT('Ctrl Pts',(-61.4540782302245,73.4191962866505,
61.8017492157138));
#213831=CARTESIAN_POINT('Ctrl Pts',(-61.4894335104073,72.4146824655236,
61.0315685733077));
#213832=CARTESIAN_POINT('Ctrl Pts',(-61.5070703523648,71.8758691137458,
60.6928252217055));
#213833=CARTESIAN_POINT('Ctrl Pts',(-61.5392428845874,70.8610138634007,
60.1793893499888));
#213834=CARTESIAN_POINT('Ctrl Pts',(-61.5535907935117,70.39678499443,59.9858993636265));
#213835=CARTESIAN_POINT('Ctrl Pts',(-61.585876373904,69.3138961483048,59.6253154434844));
#213836=CARTESIAN_POINT('Ctrl Pts',(-61.603494777744,68.6899897691559,59.4805612565544));
#213837=CARTESIAN_POINT('Ctrl Pts',(-61.6480441332805,67.1159772358438,
59.2675350741756));
#213838=CARTESIAN_POINT('Ctrl Pts',(-61.6752737373193,66.1621390075234,
59.271516041684));
#213839=CARTESIAN_POINT('Ctrl Pts',(-61.7207714169046,64.5507744930857,
59.5033120523018));
#213840=CARTESIAN_POINT('Ctrl Pts',(-61.7396021229131,63.8902760825381,
59.6664228414106));
#213841=CARTESIAN_POINT('Ctrl Pts',(-61.7736284575458,62.7577122202194,
60.0687646542903));
#213842=CARTESIAN_POINT('Ctrl Pts',(-61.7885898979955,62.2788005150607,
60.2814151338566));
#213843=CARTESIAN_POINT('Ctrl Pts',(-61.8177696215568,61.3682737972457,
60.7722496029264));
#213844=CARTESIAN_POINT('Ctrl Pts',(-61.8319097085121,60.9370959355713,
61.0481221638876));
#213845=CARTESIAN_POINT('Ctrl Pts',(-61.8635657927953,60.0320550465909,
61.7275375424783));
#213846=CARTESIAN_POINT('Ctrl Pts',(-61.8811261608956,59.5706660897355,
62.1443605664694));
#213847=CARTESIAN_POINT('Ctrl Pts',(-61.9371865882037,58.2340501941442,
63.5925388739433));
#213848=CARTESIAN_POINT('Ctrl Pts',(-61.9740772309726,57.5232964863006,
64.7559831093433));
#213849=CARTESIAN_POINT('Ctrl Pts',(-62.0507304415328,56.595657382813,67.2859393327457));
#213850=CARTESIAN_POINT('Ctrl Pts',(-62.0874436008208,56.385669728745,68.6270190094509));
#213851=CARTESIAN_POINT('Ctrl Pts',(-62.1256936736044,56.4405092384687,
69.970341174655));
#213852=CARTESIAN_POINT('Ctrl Pts',(-62.5017927901887,76.1552807340937,
73.4662010514616));
#213853=CARTESIAN_POINT('Ctrl Pts',(-62.4841922972289,75.9145711506133,
74.0488123192402));
#213854=CARTESIAN_POINT('Ctrl Pts',(-62.4666695608352,75.6205925594882,
74.6080634458034));
#213855=CARTESIAN_POINT('Ctrl Pts',(-62.4394943477806,75.0973719085795,
75.4133374247731));
#213856=CARTESIAN_POINT('Ctrl Pts',(-62.4301092507227,74.9044674712425,
75.6810234098114));
#213857=CARTESIAN_POINT('Ctrl Pts',(-62.3906691516004,74.0402843286251,
76.7658050470616));
#213858=CARTESIAN_POINT('Ctrl Pts',(-62.3617368215435,73.2575992204254,
77.4858024457807));
#213859=CARTESIAN_POINT('Ctrl Pts',(-62.3224962160946,72.1053173772563,
78.25615692612));
#213860=CARTESIAN_POINT('Ctrl Pts',(-62.3131328650323,71.823252316642,78.4256879595615));
#213861=CARTESIAN_POINT('Ctrl Pts',(-62.2743688109905,70.6222510105518,
79.0710130229089));
#213862=CARTESIAN_POINT('Ctrl Pts',(-62.2460538557988,69.6420793705324,
79.4198942368236));
#213863=CARTESIAN_POINT('Ctrl Pts',(-62.2074497315998,68.3027992898412,
79.6786487708405));
#213864=CARTESIAN_POINT('Ctrl Pts',(-62.1980699502291,67.9764083234649,
79.7255219348873));
#213865=CARTESIAN_POINT('Ctrl Pts',(-62.1587963366469,66.6014304642697,
79.8557322082481));
#213866=CARTESIAN_POINT('Ctrl Pts',(-62.1300162389156,65.5454851851599,
79.793178877457));
#213867=CARTESIAN_POINT('Ctrl Pts',(-62.0855242684048,64.0092360112201,
79.461304617849));
#213868=CARTESIAN_POINT('Ctrl Pts',(-62.070654090811,63.5099597587049,79.3129472836041));
#213869=CARTESIAN_POINT('Ctrl Pts',(-62.0466204641156,62.7143708676141,
79.0090169142959));
#213870=CARTESIAN_POINT('Ctrl Pts',(-62.0373875858622,62.4105596550341,
78.8757329341445));
#213871=CARTESIAN_POINT('Ctrl Pts',(-61.9904501189389,60.9038137257355,
78.1255817594361));
#213872=CARTESIAN_POINT('Ctrl Pts',(-61.9519710838904,59.8248949818888,
77.2897960181841));
#213873=CARTESIAN_POINT('Ctrl Pts',(-61.8792589333449,58.1163135090342,
75.3201748664833));
#213874=CARTESIAN_POINT('Ctrl Pts',(-61.8434477977863,57.4747010030091,
74.228320341494));
#213875=CARTESIAN_POINT('Ctrl Pts',(-61.7895071829267,56.8162421860416,
72.413248143466));
#213876=CARTESIAN_POINT('Ctrl Pts',(-61.7707657618205,56.6492959879891,
71.7575500086725));
#213877=CARTESIAN_POINT('Ctrl Pts',(-61.7325192602644,56.4466488491963,
70.42227352131));
#213878=CARTESIAN_POINT('Ctrl Pts',(-61.7132062075065,56.411563542068,69.7459346692063));
#213879=CARTESIAN_POINT('Ctrl Pts',(-61.6754559768368,56.4749534317402,
68.3970798056311));
#213880=CARTESIAN_POINT('Ctrl Pts',(-61.6567441080256,56.5731019559975,
67.7278599535121));
#213881=CARTESIAN_POINT('Ctrl Pts',(-61.6283190342541,56.8160501993116,
66.7531936361492));
#213882=CARTESIAN_POINT('Ctrl Pts',(-61.6189341589787,56.9111982087794,
66.4372681446033));
#213883=CARTESIAN_POINT('Ctrl Pts',(-61.5795010328776,57.37465676238,65.1303265128581));
#213884=CARTESIAN_POINT('Ctrl Pts',(-61.5505750818935,57.8798668347393,
64.1947793356987));
#213885=CARTESIAN_POINT('Ctrl Pts',(-61.5113410431149,58.7180248529935,
63.0911217362924));
#213886=CARTESIAN_POINT('Ctrl Pts',(-61.5019775256112,58.9294404974505,
62.8389131309679));
#213887=CARTESIAN_POINT('Ctrl Pts',(-61.4632083193789,59.8546679717751,
61.8372687115672));
#213888=CARTESIAN_POINT('Ctrl Pts',(-61.4348886658117,60.6677702807964,
61.1878960272877));
#213889=CARTESIAN_POINT('Ctrl Pts',(-61.3907375002071,62.0194455357514,
60.4089801986216));
#213890=CARTESIAN_POINT('Ctrl Pts',(-61.3757162824535,62.4941382459002,
60.1820531209446));
#213891=CARTESIAN_POINT('Ctrl Pts',(-61.3515272726771,63.2934640245289,
59.8728614805776));
#213892=CARTESIAN_POINT('Ctrl Pts',(-61.3422905752263,63.6084255106306,
59.7682903446434));
#213893=CARTESIAN_POINT('Ctrl Pts',(-61.2953515245365,65.2297471767491,
59.3160256255313));
#213894=CARTESIAN_POINT('Ctrl Pts',(-61.2568736358841,66.5906529660278,
59.2139267751174));
#213895=CARTESIAN_POINT('Ctrl Pts',(-61.1815476488329,69.2716270960578,
59.5433682057727));
#213896=CARTESIAN_POINT('Ctrl Pts',(-61.1431284236275,70.5655415412455,
59.970917131753));
#213897=CARTESIAN_POINT('Ctrl Pts',(-61.0879192858583,72.2872921442577,
60.9476120127659));
#213898=CARTESIAN_POINT('Ctrl Pts',(-61.0703450852994,72.80534901744,61.3082425228484));
#213899=CARTESIAN_POINT('Ctrl Pts',(-61.0381959693188,73.672257774307,62.0387710039529));
#213900=CARTESIAN_POINT('Ctrl Pts',(-61.0237913443329,74.033043166991,62.3913688874729));
#213901=CARTESIAN_POINT('Ctrl Pts',(-60.9948506921104,74.7136963947578,
63.1624598137185));
#213902=CARTESIAN_POINT('Ctrl Pts',(-60.9803381643744,75.0302345998815,
63.5819457145789));
#213903=CARTESIAN_POINT('Ctrl Pts',(-60.9477026318596,75.6585442783944,
64.5628973954093));
#213904=CARTESIAN_POINT('Ctrl Pts',(-60.929523342466,75.9525650523743,65.133134905363));
#213905=CARTESIAN_POINT('Ctrl Pts',(-60.8933588951831,76.4274396498665,
66.3136799793408));
#213906=CARTESIAN_POINT('Ctrl Pts',(-60.8757973779874,76.6086228929761,
66.9208855829549));
#213907=CARTESIAN_POINT('Ctrl Pts',(-60.8397638334601,76.8617260615403,
68.1856495294659));
#213908=CARTESIAN_POINT('Ctrl Pts',(-60.8211917604325,76.9284120227369,
68.8413094635645));
#213909=CARTESIAN_POINT('Ctrl Pts',(-60.7640366603233,76.9388849077235,
70.8504171533983));
#213910=CARTESIAN_POINT('Ctrl Pts',(-60.7271143861794,76.6785175472096,
72.1901584257861));
#213911=CARTESIAN_POINT('Ctrl Pts',(-60.6884024604886,76.1622782263207,
73.4492321076023));
#213912=CARTESIAN_POINT('Ctrl Pts',(-60.6881413685773,76.1587850810255,
73.4577191622393));
#213913=CARTESIAN_POINT('Ctrl Pts',(-60.6878802914039,76.1552807429917,
73.4662010299249));
#213914=CARTESIAN_POINT('Origin',(-21.6548258024609,75.,72.9888893865801));
#213915=CARTESIAN_POINT('',(-23.7494631149408,87.0149197165679,77.9529305028912));
#213916=CARTESIAN_POINT('',(-23.5675316904177,87.0149197054641,77.9529305294612));
#213917=CARTESIAN_POINT('',(-21.6548258024609,87.0149197055719,77.9529305295058));
#213918=CARTESIAN_POINT('',(-23.5675316903009,81.8060517138039,84.0648841531475));
#213919=CARTESIAN_POINT('Ctrl Pts',(-23.7494631142982,87.0149197165734,
77.9529305028779));
#213920=CARTESIAN_POINT('Ctrl Pts',(-23.7335469728164,86.7427187400688,
78.6117632568488));
#213921=CARTESIAN_POINT('Ctrl Pts',(-23.7173356484354,86.4167322474098,
79.2472274990606));
#213922=CARTESIAN_POINT('Ctrl Pts',(-23.6789660693055,85.5103834448235,
80.7050232771271));
#213923=CARTESIAN_POINT('Ctrl Pts',(-23.6573462260829,84.8836923221021,
81.4929757686694));
#213924=CARTESIAN_POINT('Ctrl Pts',(-23.6129675706424,83.4586738982171,
82.9118922602039));
#213925=CARTESIAN_POINT('Ctrl Pts',(-23.5899173818351,82.6644777038016,
83.5373927807216));
#213926=CARTESIAN_POINT('Ctrl Pts',(-23.5675316903009,81.8060517138039,
84.0648841531474));
#213927=CARTESIAN_POINT('Origin',(-23.5675316903009,75.,72.9888893865801));
#213928=CARTESIAN_POINT('Origin',(-21.6548258024609,75.,72.9888893865801));
#213929=CARTESIAN_POINT('',(-25.5628518781596,87.0149197055719,77.9529305295058));
#213930=CARTESIAN_POINT('',(-25.2581222247367,87.0149197055719,77.9529305295058));
#213931=CARTESIAN_POINT('',(-21.6548258024609,87.0149197055719,77.9529305295058));
#213932=CARTESIAN_POINT('Ctrl Pts',(-25.5628518781596,87.0149197055719,
77.9529305295058));
#213933=CARTESIAN_POINT('Ctrl Pts',(-25.5342348853662,86.524408980039,79.1401581958999));
#213934=CARTESIAN_POINT('Ctrl Pts',(-25.506780222184,85.859722271091,80.250298001449));
#213935=CARTESIAN_POINT('Ctrl Pts',(-25.4598723099545,84.537509974558,81.858175099878));
#213936=CARTESIAN_POINT('Ctrl Pts',(-25.4420110595247,83.9790909030928,
82.4230970114736));
#213937=CARTESIAN_POINT('Ctrl Pts',(-25.4061623457357,82.7368144036211,
83.46899814892));
#213938=CARTESIAN_POINT('Ctrl Pts',(-25.3882919641257,82.0510448433343,
83.9421414655669));
#213939=CARTESIAN_POINT('Ctrl Pts',(-25.3604186304516,80.9574848293449,
84.551118847472));
#213940=CARTESIAN_POINT('Ctrl Pts',(-25.350916041777,80.580447467698,84.7377352997618));
#213941=CARTESIAN_POINT('Ctrl Pts',(-25.3031624035225,78.63948693439,85.5838769037982));
#213942=CARTESIAN_POINT('Ctrl Pts',(-25.2671492367615,76.9661123482892,
85.9509106010206));
#213943=CARTESIAN_POINT('Ctrl Pts',(-25.2110937833321,74.4788017793984,
86.0024934260275));
#213944=CARTESIAN_POINT('Ctrl Pts',(-25.1932702125315,73.6882045327406,
85.9466959719249));
#213945=CARTESIAN_POINT('Ctrl Pts',(-25.1573545097553,72.0826904798649,
85.6848678052996));
#213946=CARTESIAN_POINT('Ctrl Pts',(-25.1393881007222,71.272686857849,85.4711042328599));
#213947=CARTESIAN_POINT('Ctrl Pts',(-25.1114105692349,70.0945458901189,
85.0351860135718));
#213948=CARTESIAN_POINT('Ctrl Pts',(-25.1019084706643,69.7075720149055,
84.8702591362608));
#213949=CARTESIAN_POINT('Ctrl Pts',(-25.0541466985092,67.8019242994457,
83.9464752146266));
#213950=CARTESIAN_POINT('Ctrl Pts',(-25.0181261672443,66.4342651665973,
82.9140686343922));
#213951=CARTESIAN_POINT('Ctrl Pts',(-24.9617637202306,64.7681195006503,
81.0483612746353));
#213952=CARTESIAN_POINT('Ctrl Pts',(-24.9436507628794,64.2893456262384,
80.4002570731414));
#213953=CARTESIAN_POINT('Ctrl Pts',(-24.9079838183038,63.4533687006,79.0167666311959));
#213954=CARTESIAN_POINT('Ctrl Pts',(-24.8905073373037,63.0993246365807,
78.2835953282246));
#213955=CARTESIAN_POINT('Ctrl Pts',(-24.8630645895267,62.6693559715836,
77.1279872899257));
#213956=CARTESIAN_POINT('Ctrl Pts',(-24.8535596220526,62.5419006961698,
76.7268933833944));
#213957=CARTESIAN_POINT('Ctrl Pts',(-24.8058503480044,61.9998300936705,
74.6822528929047));
#213958=CARTESIAN_POINT('Ctrl Pts',(-24.7698813216614,61.8900144000392,
72.9749547962966));
#213959=CARTESIAN_POINT('Ctrl Pts',(-24.7143843430214,62.2110645219798,
70.5324051813204));
#213960=CARTESIAN_POINT('Ctrl Pts',(-24.6970419222636,62.3787014145589,
69.7804588734101));
#213961=CARTESIAN_POINT('Ctrl Pts',(-24.6632901642082,62.8415470111348,
68.3255961552879));
#213962=CARTESIAN_POINT('Ctrl Pts',(-24.6469281069572,63.1339929094341,
67.6249218798871));
#213963=CARTESIAN_POINT('Ctrl Pts',(-24.6085627568924,63.9405482866857,
66.0861333089842));
#213964=CARTESIAN_POINT('Ctrl Pts',(-24.5861603841818,64.4918984265292,
65.2727174091015));
#213965=CARTESIAN_POINT('Ctrl Pts',(-24.5478929218032,65.6118513645777,
63.9660075581907));
#213966=CARTESIAN_POINT('Ctrl Pts',(-24.5317890202232,66.1416283591875,
63.4453584440137));
#213967=CARTESIAN_POINT('Ctrl Pts',(-24.478678041785,68.0084483911288,61.9008022575695));
#213968=CARTESIAN_POINT('Ctrl Pts',(-24.4404197776328,69.4997497811424,
61.0903726254267));
#213969=CARTESIAN_POINT('Ctrl Pts',(-24.3944539989604,71.5059127553458,
60.4601679353283));
#213970=CARTESIAN_POINT('Ctrl Pts',(-24.3852625240197,71.9137615352939,
60.3535169796907));
#213971=CARTESIAN_POINT('Ctrl Pts',(-24.3589735379831,73.0715263622877,
60.1101762674291));
#213972=CARTESIAN_POINT('Ctrl Pts',(-24.3416198348962,73.829319278862,60.0193181026902));
#213973=CARTESIAN_POINT('Ctrl Pts',(-24.3153476699086,75.0034597100019,
59.9823322175879));
#213974=CARTESIAN_POINT('Ctrl Pts',(-24.3062012240956,75.4166079409204,
59.9890054637244));
#213975=CARTESIAN_POINT('Ctrl Pts',(-24.2791962632356,76.6425985097674,
60.0673205172565));
#213976=CARTESIAN_POINT('Ctrl Pts',(-24.2616122208314,77.4497550355971,
60.1957750471302));
#213977=CARTESIAN_POINT('Ctrl Pts',(-24.2174452577425,79.358630216496,60.6869544139071));
#213978=CARTESIAN_POINT('Ctrl Pts',(-24.1913574606352,80.4343690257702,
61.1228465529736));
#213979=CARTESIAN_POINT('Ctrl Pts',(-24.1481030157837,82.1490683603878,
62.1003517955465));
#213980=CARTESIAN_POINT('Ctrl Pts',(-24.1303270077378,82.8200217247972,
62.5717550113872));
#213981=CARTESIAN_POINT('Ctrl Pts',(-24.0934607218744,84.0657367716937,
63.6355618776563));
#213982=CARTESIAN_POINT('Ctrl Pts',(-24.0749439293719,84.6374991871952,
64.2258447186507));
#213983=CARTESIAN_POINT('Ctrl Pts',(-24.0399256256361,85.6278339792556,
65.4633093765027));
#213984=CARTESIAN_POINT('Ctrl Pts',(-24.0234209550587,86.052170387339,66.1016021099573));
#213985=CARTESIAN_POINT('Ctrl Pts',(-23.986480861679,86.8507665052518,67.5686511770748));
#213986=CARTESIAN_POINT('Ctrl Pts',(-23.9657965863791,87.1993699844182,
68.4068572517046));
#213987=CARTESIAN_POINT('Ctrl Pts',(-23.9286751730297,87.6752780539253,
70.0030333534241));
#213988=CARTESIAN_POINT('Ctrl Pts',(-23.9121337744981,87.8281748594039,
70.7492595749639));
#213989=CARTESIAN_POINT('Ctrl Pts',(-23.8584168754291,88.1082626488629,
73.18626923684));
#213990=CARTESIAN_POINT('Ctrl Pts',(-23.8198811582619,87.9712232475782,
74.8896421088131));
#213991=CARTESIAN_POINT('Ctrl Pts',(-23.7736771942424,87.3973357905358,
76.9237439180041));
#213992=CARTESIAN_POINT('Ctrl Pts',(-23.7645045072649,87.2635037493548,
77.3228814710253));
#213993=CARTESIAN_POINT('Ctrl Pts',(-23.7532764802347,87.0794545224418,
77.7945212352546));
#213994=CARTESIAN_POINT('Ctrl Pts',(-23.7513724844872,87.0475741404218,
77.8738940340539));
#213995=CARTESIAN_POINT('Ctrl Pts',(-23.7494631142981,87.0149197165734,
77.952930502878));
#213996=CARTESIAN_POINT('',(-23.5675316904177,87.9904527821819,72.490756361305));
#213997=CARTESIAN_POINT('Origin',(-23.5675316903009,75.,72.9888893865801));
#213998=CARTESIAN_POINT('',(-23.5676924422401,87.9901782351292,72.4836474449556));
#213999=CARTESIAN_POINT('Ctrl Pts',(-23.5675316904177,87.9904527821819,
72.490756361305));
#214000=CARTESIAN_POINT('Ctrl Pts',(-23.5675873235413,87.9904177973111,
72.4883921330275));
#214001=CARTESIAN_POINT('Ctrl Pts',(-23.5676429566649,87.9903821670158,
72.4860278991294));
#214002=CARTESIAN_POINT('Ctrl Pts',(-23.5676985897885,87.9903458912847,
72.483663659963));
#214003=CARTESIAN_POINT('',(-24.3504740810588,62.9850814687467,68.0248454013454));
#214004=CARTESIAN_POINT('Ctrl Pts',(-23.5676924422401,87.9901782351292,
72.4836474449556));
#214005=CARTESIAN_POINT('Ctrl Pts',(-23.579866516381,87.9692398735109,71.9453052627941));
#214006=CARTESIAN_POINT('Ctrl Pts',(-23.5921363130451,87.9148563762113,
71.4087819670215));
#214007=CARTESIAN_POINT('Ctrl Pts',(-23.6163677338714,87.7397953767718,
70.3453912998746));
#214008=CARTESIAN_POINT('Ctrl Pts',(-23.6283050919863,87.6192627227127,
69.8195543991763));
#214009=CARTESIAN_POINT('Ctrl Pts',(-23.6548809171444,87.274925491956,68.6550241764215));
#214010=CARTESIAN_POINT('Ctrl Pts',(-23.6693811451346,87.0332275773113,
68.023246912331));
#214011=CARTESIAN_POINT('Ctrl Pts',(-23.7137157498716,86.1721125160913,
66.2095881368177));
#214012=CARTESIAN_POINT('Ctrl Pts',(-23.7444931511871,85.4190515220121,
65.1010209222251));
#214013=CARTESIAN_POINT('Ctrl Pts',(-23.7829206451029,84.224537357421,63.8191474354379));
#214014=CARTESIAN_POINT('Ctrl Pts',(-23.792027110996,83.9236127931091,63.5260466635811));
#214015=CARTESIAN_POINT('Ctrl Pts',(-23.8386873210016,82.3161449889425,
62.10535751495));
#214016=CARTESIAN_POINT('Ctrl Pts',(-23.8784725722724,80.8086174661391,
61.231457189744));
#214017=CARTESIAN_POINT('Ctrl Pts',(-23.9304375078449,78.5567988600886,
60.467921189179));
#214018=CARTESIAN_POINT('Ctrl Pts',(-23.944451268879,77.9241855151621,60.3052546592794));
#214019=CARTESIAN_POINT('Ctrl Pts',(-23.9734151603134,76.6342131999977,
60.0752384248521));
#214020=CARTESIAN_POINT('Ctrl Pts',(-23.9884516930088,75.9785489184828,
60.0090797283746));
#214021=CARTESIAN_POINT('Ctrl Pts',(-24.0419614354671,73.6141729955495,
59.9507329783205));
#214022=CARTESIAN_POINT('Ctrl Pts',(-24.077636442192,71.9159497188868,60.2451583872028));
#214023=CARTESIAN_POINT('Ctrl Pts',(-24.133518316589,69.6097364794835,61.1343653793949));
#214024=CARTESIAN_POINT('Ctrl Pts',(-24.1509196237138,68.9219381508364,
61.4718643510489));
#214025=CARTESIAN_POINT('Ctrl Pts',(-24.1919754352576,67.3408833122785,
62.4289671184786));
#214026=CARTESIAN_POINT('Ctrl Pts',(-24.2148896691121,66.4877584805762,
63.1037622587486));
#214027=CARTESIAN_POINT('Ctrl Pts',(-24.2533759923444,65.2787446307964,
64.3339212689603));
#214028=CARTESIAN_POINT('Ctrl Pts',(-24.2680418990405,64.8636792060789,
64.8239471120891));
#214029=CARTESIAN_POINT('Ctrl Pts',(-24.2940935767858,64.1847342464081,
65.7574852536576));
#214030=CARTESIAN_POINT('Ctrl Pts',(-24.3055351499497,63.9078155261211,
66.1898725772495));
#214031=CARTESIAN_POINT('Ctrl Pts',(-24.3281398473403,63.4058937918095,
67.0862442270404));
#214032=CARTESIAN_POINT('Ctrl Pts',(-24.3392828333262,63.1814723764496,
67.5495029661559));
#214033=CARTESIAN_POINT('Ctrl Pts',(-24.3504740810588,62.9850814687467,
68.0248454013453));
#214034=CARTESIAN_POINT('Ctrl Pts',(-25.2581222247367,87.0149197055719,
77.9529305295058));
#214035=CARTESIAN_POINT('Ctrl Pts',(-25.2371139398987,86.6552691734239,
78.8234253826726));
#214036=CARTESIAN_POINT('Ctrl Pts',(-25.21540963982,86.2018081844466,79.6529161935503));
#214037=CARTESIAN_POINT('Ctrl Pts',(-25.1819196289472,85.3392991491601,
80.8893513410912));
#214038=CARTESIAN_POINT('Ctrl Pts',(-25.169745613827,84.9866696364086,81.3306425359654));
#214039=CARTESIAN_POINT('Ctrl Pts',(-25.1201329901855,83.4509550568779,
83.0149971163702));
#214040=CARTESIAN_POINT('Ctrl Pts',(-25.0805800079591,82.0559752886199,
84.0412504737423));
#214041=CARTESIAN_POINT('Ctrl Pts',(-25.0292609529725,79.9279759288953,
85.0353238638776));
#214042=CARTESIAN_POINT('Ctrl Pts',(-25.0156013108458,79.3350240530373,
85.2611792863697));
#214043=CARTESIAN_POINT('Ctrl Pts',(-24.9750095399314,77.5673393760012,
85.7903165773942));
#214044=CARTESIAN_POINT('Ctrl Pts',(-24.9470863164354,76.3638564276923,
85.9737863082347));
#214045=CARTESIAN_POINT('Ctrl Pts',(-24.9074472810324,74.5784121188101,
85.9947286348465));
#214046=CARTESIAN_POINT('Ctrl Pts',(-24.8950686465802,74.0045315539647,
85.9634276728041));
#214047=CARTESIAN_POINT('Ctrl Pts',(-24.8452804596057,71.7345459005824,
85.6880829545065));
#214048=CARTESIAN_POINT('Ctrl Pts',(-24.8057674949643,70.0918887737977,
85.1479662710231));
#214049=CARTESIAN_POINT('Ctrl Pts',(-24.7535182297264,68.0089873638452,
83.9701726821653));
#214050=CARTESIAN_POINT('Ctrl Pts',(-24.7388535665513,67.4439846541188,
83.5893363030982));
#214051=CARTESIAN_POINT('Ctrl Pts',(-24.698671883696,66.0184478844832,82.4563454180001));
#214052=CARTESIAN_POINT('Ctrl Pts',(-24.6723892453867,65.2228080106428,
81.6322347885949));
#214053=CARTESIAN_POINT('Ctrl Pts',(-24.6343728549527,64.2061403484082,
80.256461050092));
#214054=CARTESIAN_POINT('Ctrl Pts',(-24.6220757074902,63.8978517413121,
79.7761802700339));
#214055=CARTESIAN_POINT('Ctrl Pts',(-24.5723410170108,62.7926248175406,
77.7764145957868));
#214056=CARTESIAN_POINT('Ctrl Pts',(-24.5327923771568,62.2682504897212,
76.1262380636946));
#214057=CARTESIAN_POINT('Ctrl Pts',(-24.4727154955514,61.9651282535958,
73.3931830852563));
#214058=CARTESIAN_POINT('Ctrl Pts',(-24.450423176884,61.9742992358757,72.3544900136934));
#214059=CARTESIAN_POINT('Ctrl Pts',(-24.4014705356543,62.2527429291364,
70.1930457335824));
#214060=CARTESIAN_POINT('Ctrl Pts',(-24.3753730910726,62.5481383061654,
69.0824179202065));
#214061=CARTESIAN_POINT('Ctrl Pts',(-24.3504740810588,62.9850814687467,
68.0248454013453));
#214062=CARTESIAN_POINT('Origin',(-21.6548258024609,75.,72.9888893865801));
#214063=CARTESIAN_POINT('',(-27.3772428998516,87.0149197057112,77.9529305291688));
#214064=CARTESIAN_POINT('',(-27.071820154481,87.0149197055719,77.9529305295058));
#214065=CARTESIAN_POINT('',(-21.6548258024609,87.0149197055719,77.9529305295058));
#214066=CARTESIAN_POINT('',(-25.7929126252424,86.9560726709681,67.8848479330955));
#214067=CARTESIAN_POINT('Ctrl Pts',(-27.3772428998516,87.0149197058504,
77.9529305288318));
#214068=CARTESIAN_POINT('Ctrl Pts',(-27.3585026366247,86.6920930370044,
78.7342972407386));
#214069=CARTESIAN_POINT('Ctrl Pts',(-27.3400433155629,86.2938005397031,
79.4823430155439));
#214070=CARTESIAN_POINT('Ctrl Pts',(-27.3118499074165,85.5953734961236,
80.5328339483534));
#214071=CARTESIAN_POINT('Ctrl Pts',(-27.3025307943751,85.348569085002,80.8679856481114));
#214072=CARTESIAN_POINT('Ctrl Pts',(-27.274613720519,84.5582100824996,81.839921252302));
#214073=CARTESIAN_POINT('Ctrl Pts',(-27.2563294776812,83.9688536705665,
82.4366299088375));
#214074=CARTESIAN_POINT('Ctrl Pts',(-27.2185818420799,82.66146632564,83.5269761458286));
#214075=CARTESIAN_POINT('Ctrl Pts',(-27.1990975050948,81.9429570105276,
84.01362043297));
#214076=CARTESIAN_POINT('Ctrl Pts',(-27.1608686233789,80.4246186178578,
84.8342939279908));
#214077=CARTESIAN_POINT('Ctrl Pts',(-27.1420577344777,79.629070187145,85.1672227095795));
#214078=CARTESIAN_POINT('Ctrl Pts',(-27.1134541677068,78.4061460599412,
85.5417166702577));
#214079=CARTESIAN_POINT('Ctrl Pts',(-27.1040817102919,78.0001138129745,
85.6449006902839));
#214080=CARTESIAN_POINT('Ctrl Pts',(-27.0756316214871,76.7475906674452,
85.899527575069));
#214081=CARTESIAN_POINT('Ctrl Pts',(-27.0568990797288,75.8904665626252,
85.9868013423841));
#214082=CARTESIAN_POINT('Ctrl Pts',(-27.0176781623146,74.127690109845,85.9910081379894));
#214083=CARTESIAN_POINT('Ctrl Pts',(-26.9974077424435,73.2265835598246,
85.8990029018832));
#214084=CARTESIAN_POINT('Ctrl Pts',(-26.968250549752,71.9348259340739,85.6292215760866));
#214085=CARTESIAN_POINT('Ctrl Pts',(-26.9591046860196,71.5316602483832,
85.5245947390282));
#214086=CARTESIAN_POINT('Ctrl Pts',(-26.9349401815241,70.488075109287,85.199561969259));
#214087=CARTESIAN_POINT('Ctrl Pts',(-26.9197323165762,69.8586419172962,
84.9481711651819));
#214088=CARTESIAN_POINT('Ctrl Pts',(-26.8859122844744,68.498424915887,84.2775901023272));
#214089=CARTESIAN_POINT('Ctrl Pts',(-26.8675404929102,67.7829525778628,
83.834140109348));
#214090=CARTESIAN_POINT('Ctrl Pts',(-26.8299101986688,66.4320387623489,
82.8035971260288));
#214091=CARTESIAN_POINT('Ctrl Pts',(-26.8105585703119,65.8021719605181,
82.2159370712263));
#214092=CARTESIAN_POINT('Ctrl Pts',(-26.7724324749667,64.6668976818974,
80.9240898258221));
#214093=CARTESIAN_POINT('Ctrl Pts',(-26.7536453108212,64.1644601915041,
80.2229397836913));
#214094=CARTESIAN_POINT('Ctrl Pts',(-26.7250956737158,63.5270109069143,
79.1162186341038));
#214095=CARTESIAN_POINT('Ctrl Pts',(-26.715761955723,63.3365114880958,78.7453361357191));
#214096=CARTESIAN_POINT('Ctrl Pts',(-26.6878646566231,62.8185801602425,
77.605278466486));
#214097=CARTESIAN_POINT('Ctrl Pts',(-26.6696154374097,62.5471417669723,
76.8130691020841));
#214098=CARTESIAN_POINT('Ctrl Pts',(-26.6329190489758,62.1639564653197,
75.2038925083435));
#214099=CARTESIAN_POINT('Ctrl Pts',(-26.6144941074024,62.049964964534,74.3913345736975));
#214100=CARTESIAN_POINT('Ctrl Pts',(-26.5772663572282,61.9744567925888,
72.7138662237188));
#214101=CARTESIAN_POINT('Ctrl Pts',(-26.5584809883254,62.0212044236113,
71.852545420024));
#214102=CARTESIAN_POINT('Ctrl Pts',(-26.5299362395003,62.2163619130141,
70.5905354922137));
#214103=CARTESIAN_POINT('Ctrl Pts',(-26.5206058473888,62.2997667635459,
70.1821865398606));
#214104=CARTESIAN_POINT('Ctrl Pts',(-26.4927037374686,62.6090275943298,
68.9686480648817));
#214105=CARTESIAN_POINT('Ctrl Pts',(-26.4744462598849,62.8930467479042,
68.1805412489976));
#214106=CARTESIAN_POINT('Ctrl Pts',(-26.4375071524084,63.6057605027665,
66.6754580572646));
#214107=CARTESIAN_POINT('Ctrl Pts',(-26.4188376326829,64.0317228180229,
65.9614423333998));
#214108=CARTESIAN_POINT('Ctrl Pts',(-26.3813781293124,65.0321953444006,
64.5994160557959));
#214109=CARTESIAN_POINT('Ctrl Pts',(-26.3625868347542,65.6091804053644,
63.9582250617695));
#214110=CARTESIAN_POINT('Ctrl Pts',(-26.3340264446216,66.553586253858,63.0978810349136));
#214111=CARTESIAN_POINT('Ctrl Pts',(-26.3246853485288,66.8752439694295,
62.8320054219483));
#214112=CARTESIAN_POINT('Ctrl Pts',(-26.2967994471399,67.8773984430049,
62.0817619822098));
#214113=CARTESIAN_POINT('Ctrl Pts',(-26.2785692142129,68.5923066241011,
61.6470051727518));
#214114=CARTESIAN_POINT('Ctrl Pts',(-26.2424224009397,70.0590097150615,
60.9382741883589));
#214115=CARTESIAN_POINT('Ctrl Pts',(-26.2245511524584,70.8042374504039,
60.6589950005373));
#214116=CARTESIAN_POINT('Ctrl Pts',(-26.1897733046434,72.3165714552708,
60.2453486461837));
#214117=CARTESIAN_POINT('Ctrl Pts',(-26.1728928390523,73.0795965666424,
60.1082578434061));
#214118=CARTESIAN_POINT('Ctrl Pts',(-26.1429023266542,74.4197179295013,
59.9892701169044));
#214119=CARTESIAN_POINT('Ctrl Pts',(-26.1300716403104,74.9918828037437,
59.9763275579365));
#214120=CARTESIAN_POINT('Ctrl Pts',(-26.0982220008237,76.4218187852646,
60.0383171234002));
#214121=CARTESIAN_POINT('Ctrl Pts',(-26.0794903366003,77.2747899921236,
60.1606308648086));
#214122=CARTESIAN_POINT('Ctrl Pts',(-26.0392642115874,79.0293957409234,
60.5928547252689));
#214123=CARTESIAN_POINT('Ctrl Pts',(-26.0180298275783,79.9218450641421,
60.9193753076888));
#214124=CARTESIAN_POINT('Ctrl Pts',(-25.9887478158431,81.1105915754084,
61.5082789939621));
#214125=CARTESIAN_POINT('Ctrl Pts',(-25.980414557455,81.4427986662038,61.6913635913145));
#214126=CARTESIAN_POINT('Ctrl Pts',(-25.9453511555322,82.7962653180951,
62.5164191486459));
#214127=CARTESIAN_POINT('Ctrl Pts',(-25.9182823831953,83.7336670457999,
63.2843824439299));
#214128=CARTESIAN_POINT('Ctrl Pts',(-25.8835582823454,84.802145820081,64.4417136345005));
#214129=CARTESIAN_POINT('Ctrl Pts',(-25.8754354658025,85.0408914382205,
64.7234931914111));
#214130=CARTESIAN_POINT('Ctrl Pts',(-25.8424562339689,85.9509334591754,
65.8952865936117));
#214131=CARTESIAN_POINT('Ctrl Pts',(-25.8175223603503,86.518524818664,66.859797753857));
#214132=CARTESIAN_POINT('Ctrl Pts',(-25.7929565710457,86.9561115222891,
67.8848324446381));
#214133=CARTESIAN_POINT('Ctrl Pts',(-25.7925315892805,86.9561078343949,
67.8848238058573));
#214134=CARTESIAN_POINT('Ctrl Pts',(-25.7738172320668,87.2899529717186,
68.6668451961985));
#214135=CARTESIAN_POINT('Ctrl Pts',(-25.7554910654485,87.5462664477491,
69.479728285654));
#214136=CARTESIAN_POINT('Ctrl Pts',(-25.7174585685915,87.89551651574,71.1393471814782));
#214137=CARTESIAN_POINT('Ctrl Pts',(-25.6982654760428,87.9885017447245,
71.9819134464591));
#214138=CARTESIAN_POINT('Ctrl Pts',(-25.6580815311063,88.0110086692369,
73.7950592766131));
#214139=CARTESIAN_POINT('Ctrl Pts',(-25.6373707278172,87.9149608356701,
74.760904048186));
#214140=CARTESIAN_POINT('Ctrl Pts',(-25.6073298168375,87.6337185281454,
76.0762223461118));
#214141=CARTESIAN_POINT('Ctrl Pts',(-25.5988027409164,87.5387580880639,
76.4417162546927));
#214142=CARTESIAN_POINT('Ctrl Pts',(-25.5810816491095,87.3082309444352,
77.1929608534129));
#214143=CARTESIAN_POINT('Ctrl Pts',(-25.5719178118877,87.1703147103061,
77.576813883658));
#214144=CARTESIAN_POINT('Ctrl Pts',(-25.5628518781596,87.0149197055719,
77.9529305295058));
#214145=CARTESIAN_POINT('Ctrl Pts',(-27.071820154481,87.0149197055719,77.9529305295058));
#214146=CARTESIAN_POINT('Ctrl Pts',(-27.0605085365974,86.8166613733047,
78.4327931806334));
#214147=CARTESIAN_POINT('Ctrl Pts',(-27.049101654611,86.5896253620448,78.9008516142056));
#214148=CARTESIAN_POINT('Ctrl Pts',(-27.0197225666822,85.9448502140688,
80.0489617246627));
#214149=CARTESIAN_POINT('Ctrl Pts',(-27.0015063043549,85.4918565712577,
80.70609693059));
#214150=CARTESIAN_POINT('Ctrl Pts',(-26.9591716635365,84.2850054963717,
82.1524488952687));
#214151=CARTESIAN_POINT('Ctrl Pts',(-26.9361717726357,83.4864499048139,
82.8965790426729));
#214152=CARTESIAN_POINT('Ctrl Pts',(-26.8941455410223,81.9446283737061,
84.0086132753054));
#214153=CARTESIAN_POINT('Ctrl Pts',(-26.8756807836608,81.2414038974203,
84.421606780749));
#214154=CARTESIAN_POINT('Ctrl Pts',(-26.8189728420717,78.9721657266138,
85.4821578977096));
#214155=CARTESIAN_POINT('Ctrl Pts',(-26.7836305989519,77.3150352142353,
85.8923958059138));
#214156=CARTESIAN_POINT('Ctrl Pts',(-26.7312779156254,74.9997905288434,
86.0039922207733));
#214157=CARTESIAN_POINT('Ctrl Pts',(-26.7169492121584,74.372336987336,85.9888485981267));
#214158=CARTESIAN_POINT('Ctrl Pts',(-26.6742994714576,72.4684258750948,
85.8046950112485));
#214159=CARTESIAN_POINT('Ctrl Pts',(-26.6471833125259,71.2138486459522,
85.4916438799536));
#214160=CARTESIAN_POINT('Ctrl Pts',(-26.6020301406656,69.3559903103541,
84.7222014240607));
#214161=CARTESIAN_POINT('Ctrl Pts',(-26.5854317064412,68.7106481624918,
84.3893060366484));
#214162=CARTESIAN_POINT('Ctrl Pts',(-26.5450219175929,67.181239395849,83.4308014465017));
#214163=CARTESIAN_POINT('Ctrl Pts',(-26.5221896305854,66.3410918902448,
82.7454188415464));
#214164=CARTESIAN_POINT('Ctrl Pts',(-26.4780446581086,64.9659409652747,
81.3044741245955));
#214165=CARTESIAN_POINT('Ctrl Pts',(-26.4572014080688,64.4076145893941,
80.5805045840409));
#214166=CARTESIAN_POINT('Ctrl Pts',(-26.4036318027753,63.1590546347934,
78.5523955573464));
#214167=CARTESIAN_POINT('Ctrl Pts',(-26.3728346457708,62.6063171379071,
77.17902371207));
#214168=CARTESIAN_POINT('Ctrl Pts',(-26.3244976064021,62.1517516696246,
75.0816632598761));
#214169=CARTESIAN_POINT('Ctrl Pts',(-26.3090236792136,62.0603060695958,
74.410685161115));
#214170=CARTESIAN_POINT('Ctrl Pts',(-26.2641235956774,61.9448936273482,
72.4048400651594));
#214171=CARTESIAN_POINT('Ctrl Pts',(-26.2360680888913,62.0734620859508,
71.0701429440428));
#214172=CARTESIAN_POINT('Ctrl Pts',(-26.1966699289764,62.5063482147525,
69.3715812671164));
#214173=CARTESIAN_POINT('Ctrl Pts',(-26.1871415785778,62.629674256928,68.9700224075527));
#214174=CARTESIAN_POINT('Ctrl Pts',(-26.1506331525675,63.1764235758087,
67.4553166575137));
#214175=CARTESIAN_POINT('Ctrl Pts',(-26.1251170344048,63.7325528158873,
66.3963153232645));
#214176=CARTESIAN_POINT('Ctrl Pts',(-26.0806649581723,64.9095364125484,
64.7501647278864));
#214177=CARTESIAN_POINT('Ctrl Pts',(-26.061906909934,65.4580950871485,64.1206280522381));
#214178=CARTESIAN_POINT('Ctrl Pts',(-26.015547404288,66.9426901021429,62.7152958770042));
#214179=CARTESIAN_POINT('Ctrl Pts',(-25.9895183092078,67.9343472290684,
62.0096573409437));
#214180=CARTESIAN_POINT('Ctrl Pts',(-25.9446017362212,69.7502091534502,
61.0667794261834));
#214181=CARTESIAN_POINT('Ctrl Pts',(-25.9258205977896,70.5264831300893,
60.7543225527409));
#214182=CARTESIAN_POINT('Ctrl Pts',(-25.8792531495497,72.4961488897322,
60.1742348887389));
#214183=CARTESIAN_POINT('Ctrl Pts',(-25.8530429820679,73.7075859543001,
59.9960325963783));
#214184=CARTESIAN_POINT('Ctrl Pts',(-25.7978641992108,76.221579111487,59.9817283532551));
#214185=CARTESIAN_POINT('Ctrl Pts',(-25.7679576827334,77.5109436766013,
60.1680641200787));
#214186=CARTESIAN_POINT('Ctrl Pts',(-25.7252345790019,79.3600452531562,
60.7253599424855));
#214187=CARTESIAN_POINT('Ctrl Pts',(-25.7115677709115,79.9544559836962,
60.9532121514447));
#214188=CARTESIAN_POINT('Ctrl Pts',(-25.6608585552852,82.0562660521998,
61.941087947732));
#214189=CARTESIAN_POINT('Ctrl Pts',(-25.6219008261527,83.4285950314223,
62.9487898664131));
#214190=CARTESIAN_POINT('Ctrl Pts',(-25.5674029111453,85.122148925319,64.790880633502));
#214191=CARTESIAN_POINT('Ctrl Pts',(-25.5497603779432,85.6164336888591,
65.4419311246971));
#214192=CARTESIAN_POINT('Ctrl Pts',(-25.5071780938393,86.6226461392791,
67.0636464884068));
#214193=CARTESIAN_POINT('Ctrl Pts',(-25.4819488655756,87.0794462568247,
68.06127024736));
#214194=CARTESIAN_POINT('Ctrl Pts',(-25.4375428607714,87.6846242953266,
69.9939712119277));
#214195=CARTESIAN_POINT('Ctrl Pts',(-25.4175628093938,87.866700763943,70.911088538553));
#214196=CARTESIAN_POINT('Ctrl Pts',(-25.3726675196419,88.0448682000109,
72.9188124382479));
#214197=CARTESIAN_POINT('Ctrl Pts',(-25.3476385525466,88.0053767103916,
74.005599745462));
#214198=CARTESIAN_POINT('Ctrl Pts',(-25.3071797422961,87.710143730812,75.821687234242));
#214199=CARTESIAN_POINT('Ctrl Pts',(-25.2909561985655,87.5237651081034,
76.5564960547168));
#214200=CARTESIAN_POINT('Ctrl Pts',(-25.2689347587987,87.1943353664899,
77.5008148016953));
#214201=CARTESIAN_POINT('Ctrl Pts',(-25.2635448812528,87.1077526672685,
77.7282384794804));
#214202=CARTESIAN_POINT('Ctrl Pts',(-25.2581222247367,87.0149197055719,
77.9529305295058));
#214203=CARTESIAN_POINT('Origin',(-21.6548258024609,75.,72.9888893865801));
#214204=CARTESIAN_POINT('',(-29.191473624437,87.0149197052612,77.9529305302578));
#214205=CARTESIAN_POINT('',(-28.8854250924613,87.0149197055719,77.9529305295058));
#214206=CARTESIAN_POINT('',(-21.6548258024609,87.0149197055719,77.9529305295058));
#214207=CARTESIAN_POINT('Ctrl Pts',(-29.191473624437,87.0149197049505,77.9529305310098));
#214208=CARTESIAN_POINT('Ctrl Pts',(-29.1748720876648,86.7289553381427,
78.6450760643983));
#214209=CARTESIAN_POINT('Ctrl Pts',(-29.1580149809245,86.3837020063489,
79.3112532791676));
#214210=CARTESIAN_POINT('Ctrl Pts',(-29.124299147414,85.571916627344,80.5931613503198));
#214211=CARTESIAN_POINT('Ctrl Pts',(-29.1075265747482,85.1040975117078,
81.2045804644005));
#214212=CARTESIAN_POINT('Ctrl Pts',(-29.0719165439695,84.0216019566031,
82.3860326371831));
#214213=CARTESIAN_POINT('Ctrl Pts',(-29.0531686040573,83.400296735343,82.9453261314133));
#214214=CARTESIAN_POINT('Ctrl Pts',(-29.0254578252239,82.3940610068601,
83.6894563361449));
#214215=CARTESIAN_POINT('Ctrl Pts',(-29.0162756596396,82.0466521866939,
83.9213623179776));
#214216=CARTESIAN_POINT('Ctrl Pts',(-28.9880846702559,80.9508731496388,
84.5788624319063));
#214217=CARTESIAN_POINT('Ctrl Pts',(-28.968753497635,80.1709259228678,84.9472287683825));
#214218=CARTESIAN_POINT('Ctrl Pts',(-28.9321198753148,78.6199709504613,
85.4994218773942));
#214219=CARTESIAN_POINT('Ctrl Pts',(-28.9149486411076,77.8572365707559,
85.6953367527481));
#214220=CARTESIAN_POINT('Ctrl Pts',(-28.8804006429214,76.319908017302,85.9447035848871));
#214221=CARTESIAN_POINT('Ctrl Pts',(-28.8630365366872,75.5488317126422,
86.000194742609));
#214222=CARTESIAN_POINT('Ctrl Pts',(-28.8299316869188,74.0577519012817,
85.974658983903));
#214223=CARTESIAN_POINT('Ctrl Pts',(-28.8142064869176,73.3403740924139,
85.9025905663761));
#214224=CARTESIAN_POINT('Ctrl Pts',(-28.7822406653669,71.9251851481273,
85.640498115977));
#214225=CARTESIAN_POINT('Ctrl Pts',(-28.7660578641987,71.229805419051,85.450965044082));
#214226=CARTESIAN_POINT('Ctrl Pts',(-28.7329339171202,69.8286644159398,
84.9409847514264));
#214227=CARTESIAN_POINT('Ctrl Pts',(-28.7160965468475,69.1285756681097,
84.6130739307271));
#214228=CARTESIAN_POINT('Ctrl Pts',(-28.6814663693343,67.7825461534335,
83.8298215910126));
#214229=CARTESIAN_POINT('Ctrl Pts',(-28.6638066304726,67.1406086921955,
83.3738511520525));
#214230=CARTESIAN_POINT('Ctrl Pts',(-28.6273228458363,65.8902559677678,
82.3030143783936));
#214231=CARTESIAN_POINT('Ctrl Pts',(-28.6085271767135,65.2939104292582,
81.679814776386));
#214232=CARTESIAN_POINT('Ctrl Pts',(-28.5799560800039,64.5061977061064,
80.6735741452155));
#214233=CARTESIAN_POINT('Ctrl Pts',(-28.5706075320066,64.2648558037467,
80.3326586225553));
#214234=CARTESIAN_POINT('Ctrl Pts',(-28.5427341981161,63.5917536584481,
79.2775744658596));
#214235=CARTESIAN_POINT('Ctrl Pts',(-28.5245241146975,63.2118827786116,
78.5328886001411));
#214236=CARTESIAN_POINT('Ctrl Pts',(-28.4889453592806,62.6239769793031,
77.0416904741416));
#214237=CARTESIAN_POINT('Ctrl Pts',(-28.4716462600002,62.4059890416338,
76.3028051357496));
#214238=CARTESIAN_POINT('Ctrl Pts',(-28.4374968922271,62.1029596373628,
74.79418291339));
#214239=CARTESIAN_POINT('Ctrl Pts',(-28.4207003956739,62.0186962073909,
74.0273904754124));
#214240=CARTESIAN_POINT('Ctrl Pts',(-28.3812460335961,61.9820704138856,
72.2562631386752));
#214241=CARTESIAN_POINT('Ctrl Pts',(-28.3588390415407,62.0771648609283,
71.2558023076267));
#214242=CARTESIAN_POINT('Ctrl Pts',(-28.3275291901714,62.3734187427387,
69.8673081502499));
#214243=CARTESIAN_POINT('Ctrl Pts',(-28.3183412063837,62.4803432102327,
69.4628411396055));
#214244=CARTESIAN_POINT('Ctrl Pts',(-28.2923755504632,62.8330635637699,
68.3490075777341));
#214245=CARTESIAN_POINT('Ctrl Pts',(-28.2755070075871,63.1210447020856,
67.6547282024298));
#214246=CARTESIAN_POINT('Ctrl Pts',(-28.2417582543861,63.8229839058438,
66.3054550517388));
#214247=CARTESIAN_POINT('Ctrl Pts',(-28.2249441368782,64.2387725268455,
65.6547251696));
#214248=CARTESIAN_POINT('Ctrl Pts',(-28.1960445766112,65.0315160668254,
64.6278736278802));
#214249=CARTESIAN_POINT('Ctrl Pts',(-28.1842258494247,65.3783142874616,
64.231011675039));
#214250=CARTESIAN_POINT('Ctrl Pts',(-28.1538344070745,66.3362913012858,
63.2605346562643));
#214251=CARTESIAN_POINT('Ctrl Pts',(-28.1355402688503,66.9805262409467,
62.7229862544525));
#214252=CARTESIAN_POINT('Ctrl Pts',(-28.0974818801123,68.3984355273252,
61.7553264165708));
#214253=CARTESIAN_POINT('Ctrl Pts',(-28.077684353741,69.1733633480648,61.3345381023075));
#214254=CARTESIAN_POINT('Ctrl Pts',(-28.0391615851677,70.7783713925089,
60.6634003441353));
#214255=CARTESIAN_POINT('Ctrl Pts',(-28.0203440667548,71.6028949814444,
60.4111510069592));
#214256=CARTESIAN_POINT('Ctrl Pts',(-27.9917283516021,72.8573435161289,
60.1598290194321));
#214257=CARTESIAN_POINT('Ctrl Pts',(-27.9823455955259,73.2721645197844,
60.0974056651172));
#214258=CARTESIAN_POINT('Ctrl Pts',(-27.9538883157487,74.5444829827186,
59.9684671118984));
#214259=CARTESIAN_POINT('Ctrl Pts',(-27.9351567136414,75.4061785530909,
59.9668347644462));
#214260=CARTESIAN_POINT('Ctrl Pts',(-27.8949029168007,77.2059437756855,
60.1423383019933));
#214261=CARTESIAN_POINT('Ctrl Pts',(-27.8736417249549,78.1372751239506,
60.3375024609604));
#214262=CARTESIAN_POINT('Ctrl Pts',(-27.8435000938951,79.4352842125235,
60.761787114919));
#214263=CARTESIAN_POINT('Ctrl Pts',(-27.8343431385889,79.8250579186713,
60.9102888508809));
#214264=CARTESIAN_POINT('Ctrl Pts',(-27.806068651421,80.9944788766643,61.4214866700108));
#214265=CARTESIAN_POINT('Ctrl Pts',(-27.7867170866246,81.7458640588492,
61.8429527291791));
#214266=CARTESIAN_POINT('Ctrl Pts',(-27.7485971918739,83.1552834822207,
62.8285874493229));
#214267=CARTESIAN_POINT('Ctrl Pts',(-27.7298045572284,83.8097219140442,
63.3904946116153));
#214268=CARTESIAN_POINT('Ctrl Pts',(-27.7012408120807,84.691884529798,64.314707962388));
#214269=CARTESIAN_POINT('Ctrl Pts',(-27.6918973945536,84.9652449281237,
64.6301847203721));
#214270=CARTESIAN_POINT('Ctrl Pts',(-27.6640152773653,85.7385092525964,
65.6145471493112));
#214271=CARTESIAN_POINT('Ctrl Pts',(-27.6457912017925,86.1896591627655,
66.3189551409814));
#214272=CARTESIAN_POINT('Ctrl Pts',(-27.6098192685302,86.9287037331747,
67.7616130856516));
#214273=CARTESIAN_POINT('Ctrl Pts',(-27.5921241879336,87.2229985640537,
68.4925905055258));
#214274=CARTESIAN_POINT('Ctrl Pts',(-27.5575468408499,87.6717811724289,
69.9851787610371));
#214275=CARTESIAN_POINT('Ctrl Pts',(-27.5406994570977,87.8277990288113,
70.7430295666117));
#214276=CARTESIAN_POINT('Ctrl Pts',(-27.5112209523472,87.9782559482579,
72.0572259881749));
#214277=CARTESIAN_POINT('Ctrl Pts',(-27.4988633979556,88.0060670538526,
72.6076465536683));
#214278=CARTESIAN_POINT('Ctrl Pts',(-27.4674693610454,87.9877096261058,
74.0173047691573));
#214279=CARTESIAN_POINT('Ctrl Pts',(-27.4487334796038,87.8913750969979,
74.8732140521648));
#214280=CARTESIAN_POINT('Ctrl Pts',(-27.4125506948449,87.5502774816522,
76.4646545510302));
#214281=CARTESIAN_POINT('Ctrl Pts',(-27.3952778289842,87.3229510848624,
77.2002187729921));
#214282=CARTESIAN_POINT('Ctrl Pts',(-27.3779066749826,87.0263291301507,
77.9252475393518));
#214283=CARTESIAN_POINT('Ctrl Pts',(-27.3775747483253,87.020636249744,77.9390942583602));
#214284=CARTESIAN_POINT('Ctrl Pts',(-27.3772428998516,87.0149197058504,
77.9529305288318));
#214285=CARTESIAN_POINT('',(-27.3009674773552,86.9560726238069,67.8848561928421));
#214286=CARTESIAN_POINT('Ctrl Pts',(-27.3016104665866,86.9561198926212,
67.8848520519528));
#214287=CARTESIAN_POINT('Ctrl Pts',(-27.2822043885439,87.2951893562206,
68.6791164534333));
#214288=CARTESIAN_POINT('Ctrl Pts',(-27.2623604058397,87.5542721652542,
69.5051986871067));
#214289=CARTESIAN_POINT('Ctrl Pts',(-27.2247684056633,87.9002962357792,
71.1748980595603));
#214290=CARTESIAN_POINT('Ctrl Pts',(-27.2067907055177,87.9906504840547,
72.0135794964742));
#214291=CARTESIAN_POINT('Ctrl Pts',(-27.1756917368117,88.0051539398962,
73.4227565893461));
#214292=CARTESIAN_POINT('Ctrl Pts',(-27.1629591016859,87.9738071072631,
73.99018325198));
#214293=CARTESIAN_POINT('Ctrl Pts',(-27.1372090798418,87.8369700906062,
75.1186947614233));
#214294=CARTESIAN_POINT('Ctrl Pts',(-27.1242209102934,87.7314420438741,
75.6785468397757));
#214295=CARTESIAN_POINT('Ctrl Pts',(-27.0980726513746,87.4382792427217,
76.8174033129033));
#214296=CARTESIAN_POINT('Ctrl Pts',(-27.0850145273716,87.2461770192046,
77.3931974461928));
#214297=CARTESIAN_POINT('Ctrl Pts',(-27.071820154481,87.0149197055719,77.9529305295058));
#214298=CARTESIAN_POINT('Ctrl Pts',(-28.8854250924613,87.0149197055719,
77.9529305295058));
#214299=CARTESIAN_POINT('Ctrl Pts',(-28.8824657061371,86.9641248974214,
78.07587381781));
#214300=CARTESIAN_POINT('Ctrl Pts',(-28.8795002899751,86.9114288111352,
78.1980719467812));
#214301=CARTESIAN_POINT('Ctrl Pts',(-28.8672396720504,86.6861614970234,
78.6991345686103));
#214302=CARTESIAN_POINT('Ctrl Pts',(-28.85790713716,86.4973408615809,79.0703713766788));
#214303=CARTESIAN_POINT('Ctrl Pts',(-28.8331154639791,85.9467030888406,
80.0353338803234));
#214304=CARTESIAN_POINT('Ctrl Pts',(-28.8179195844283,85.5545514401051,
80.610184072988));
#214305=CARTESIAN_POINT('Ctrl Pts',(-28.7840038631501,84.5919001765483,
81.8035658259997));
#214306=CARTESIAN_POINT('Ctrl Pts',(-28.7651844263082,84.0035487921546,
82.4037267980327));
#214307=CARTESIAN_POINT('Ctrl Pts',(-28.7276150004718,82.7113055402472,
83.4892160188048));
#214308=CARTESIAN_POINT('Ctrl Pts',(-28.7091084160755,82.0091389010379,
83.9703769223539));
#214309=CARTESIAN_POINT('Ctrl Pts',(-28.6710757148091,80.5111363836892,
84.7943023480581));
#214310=CARTESIAN_POINT('Ctrl Pts',(-28.6517365479907,79.7178740929953,
85.1331091609983));
#214311=CARTESIAN_POINT('Ctrl Pts',(-28.6235540749995,78.4993036765176,
85.5160051569611));
#214312=CARTESIAN_POINT('Ctrl Pts',(-28.6143870150687,78.0958534094773,
85.6217610820052));
#214313=CARTESIAN_POINT('Ctrl Pts',(-28.5866706223603,76.8708386070266,
85.8806532998752));
#214314=CARTESIAN_POINT('Ctrl Pts',(-28.567902739722,76.038917234555,85.9741983900568));
#214315=CARTESIAN_POINT('Ctrl Pts',(-28.5313313335661,74.3942339589746,
85.9999846244162));
#214316=CARTESIAN_POINT('Ctrl Pts',(-28.5136689781962,73.5852537378235,
85.9370186488788));
#214317=CARTESIAN_POINT('Ctrl Pts',(-28.4765264015262,71.9394859923286,
85.6527617372223));
#214318=CARTESIAN_POINT('Ctrl Pts',(-28.4571790904682,71.1081997231846,
85.4224853881641));
#214319=CARTESIAN_POINT('Ctrl Pts',(-28.4290075316119,69.9177814281301,
84.9615319511398));
#214320=CARTESIAN_POINT('Ctrl Pts',(-28.4198590143517,69.5372190569592,
84.7927506157629));
#214321=CARTESIAN_POINT('Ctrl Pts',(-28.3921379113707,68.4178096980704,
84.2305375552029));
#214322=CARTESIAN_POINT('Ctrl Pts',(-28.3733480092101,67.7082051386715,
83.7837768461554));
#214323=CARTESIAN_POINT('Ctrl Pts',(-28.3356160482187,66.3665029863644,
82.746023955881));
#214324=CARTESIAN_POINT('Ctrl Pts',(-28.3168778777699,65.7403786425432,
82.1539515382366));
#214325=CARTESIAN_POINT('Ctrl Pts',(-28.2785889933486,64.6137354201889,
80.8543635225977));
#214326=CARTESIAN_POINT('Ctrl Pts',(-28.2592740996115,64.1160992638615,
80.1499571314905));
#214327=CARTESIAN_POINT('Ctrl Pts',(-28.2310705762345,63.485298007818,79.0375859269632));
#214328=CARTESIAN_POINT('Ctrl Pts',(-28.2218640006324,63.2965830577881,
78.6638451860493));
#214329=CARTESIAN_POINT('Ctrl Pts',(-28.1935575655176,62.7763359508144,
77.4967242676392));
#214330=CARTESIAN_POINT('Ctrl Pts',(-28.1742147305241,62.5051462879013,
76.6790331332835));
#214331=CARTESIAN_POINT('Ctrl Pts',(-28.13553707715,62.1225407789516,74.9773354996262));
#214332=CARTESIAN_POINT('Ctrl Pts',(-28.1162057659808,62.0170866958016,
74.0965199011238));
#214333=CARTESIAN_POINT('Ctrl Pts',(-28.078268587886,61.987921446801,72.3962011304826));
#214334=CARTESIAN_POINT('Ctrl Pts',(-28.0600134566556,62.0507353882327,
71.5810452228492));
#214335=CARTESIAN_POINT('Ctrl Pts',(-28.0236265245261,62.3315440089111,
69.9545773365316));
#214336=CARTESIAN_POINT('Ctrl Pts',(-28.0051829628842,62.5524646578503,
69.1475767222341));
#214337=CARTESIAN_POINT('Ctrl Pts',(-27.9771298133304,62.9982787259586,
67.9754591654159));
#214338=CARTESIAN_POINT('Ctrl Pts',(-27.9677390142899,63.1662066934128,
67.5910069257234));
#214339=CARTESIAN_POINT('Ctrl Pts',(-27.9370287574911,63.7818224627086,
66.349060825342));
#214340=CARTESIAN_POINT('Ctrl Pts',(-27.9158767653462,64.3065324424989,
65.533381975057));
#214341=CARTESIAN_POINT('Ctrl Pts',(-27.8849412670348,65.1801585010924,
64.4598336454975));
#214342=CARTESIAN_POINT('Ctrl Pts',(-27.8755848279818,65.4589341724681,
64.1490849776268));
#214343=CARTESIAN_POINT('Ctrl Pts',(-27.8473308132092,66.3516610491003,
63.2454906496998));
#214344=CARTESIAN_POINT('Ctrl Pts',(-27.8287354763865,67.0094212758992,
62.699173963006));
#214345=CARTESIAN_POINT('Ctrl Pts',(-27.790598345434,68.4285698429715,61.7391537518352));
#214346=CARTESIAN_POINT('Ctrl Pts',(-27.7712781789703,69.1873064754114,
61.3290072595462));
#214347=CARTESIAN_POINT('Ctrl Pts',(-27.7430781552989,70.3667123452662,
60.8353920205676));
#214348=CARTESIAN_POINT('Ctrl Pts',(-27.7338787555852,70.7600093741734,
60.6926569597947));
#214349=CARTESIAN_POINT('Ctrl Pts',(-27.7055841569337,71.9804540657243,
60.3152650493847));
#214350=CARTESIAN_POINT('Ctrl Pts',(-27.6862456860974,72.824555129948,60.1434294170083));
#214351=CARTESIAN_POINT('Ctrl Pts',(-27.6496231645155,74.4670898531631,
59.9757072121913));
#214352=CARTESIAN_POINT('Ctrl Pts',(-27.6323226821408,75.2604702770383,
59.9674045950463));
#214353=CARTESIAN_POINT('Ctrl Pts',(-27.5955515295513,76.9072526729874,
60.1008067118721));
#214354=CARTESIAN_POINT('Ctrl Pts',(-27.5762273817978,77.7558348782639,
60.2552460394781));
#214355=CARTESIAN_POINT('Ctrl Pts',(-27.5480309082657,78.9846379265348,
60.6075604536139));
#214356=CARTESIAN_POINT('Ctrl Pts',(-27.5388377802742,79.380570584004,60.7420429913732));
#214357=CARTESIAN_POINT('Ctrl Pts',(-27.5105536384159,80.5686610096575,
61.2105913528594));
#214358=CARTESIAN_POINT('Ctrl Pts',(-27.4912191807338,81.3347621600151,
61.6042915492844));
#214359=CARTESIAN_POINT('Ctrl Pts',(-27.4548946107977,82.7098171497384,
62.4929847277351));
#214360=CARTESIAN_POINT('Ctrl Pts',(-27.437895175373,83.3240090917863,62.9730931068896));
#214361=CARTESIAN_POINT('Ctrl Pts',(-27.4008866114246,84.5376412426188,
64.1109558996629));
#214362=CARTESIAN_POINT('Ctrl Pts',(-27.3809948754877,85.1201218069142,
64.7811217819716));
#214363=CARTESIAN_POINT('Ctrl Pts',(-27.3514639952375,85.8909626243882,
65.8760463333275));
#214364=CARTESIAN_POINT('Ctrl Pts',(-27.3414897687577,86.1324106356795,
66.2602166990751));
#214365=CARTESIAN_POINT('Ctrl Pts',(-27.3213168088313,86.5756651997547,
67.0548885316681));
#214366=CARTESIAN_POINT('Ctrl Pts',(-27.3111305725315,86.7768845333005,
67.4649977218528));
#214367=CARTESIAN_POINT('Ctrl Pts',(-27.3009162452284,86.9561136407892,
67.8848374071686));
#214368=CARTESIAN_POINT('Origin',(-21.6548258024609,75.,72.9888893865801));
#214369=CARTESIAN_POINT('',(-31.0052564152503,87.0149197055719,77.9529305295058));
#214370=CARTESIAN_POINT('',(-30.6991941617974,87.0149197055719,77.9529305295058));
#214371=CARTESIAN_POINT('',(-21.6548258024609,87.0149197055719,77.9529305295058));
#214372=CARTESIAN_POINT('Ctrl Pts',(-31.0052564152503,87.0149197055719,
77.9529305295058));
#214373=CARTESIAN_POINT('Ctrl Pts',(-30.9917690488268,86.7838685708455,
78.5121645792832));
#214374=CARTESIAN_POINT('Ctrl Pts',(-30.978424675615,86.5139457893124,79.0548487104576));
#214375=CARTESIAN_POINT('Ctrl Pts',(-30.947081719252,85.7934089254036,80.2805586134048));
#214376=CARTESIAN_POINT('Ctrl Pts',(-30.9288274919334,85.3144592787945,
80.9436385734192));
#214377=CARTESIAN_POINT('Ctrl Pts',(-30.8907219891804,84.1888208488232,
82.2279694179499));
#214378=CARTESIAN_POINT('Ctrl Pts',(-30.8712396609758,83.5336950227652,
82.8362782998089));
#214379=CARTESIAN_POINT('Ctrl Pts',(-30.8324131676161,82.1350383383838,
83.8897976090933));
#214380=CARTESIAN_POINT('Ctrl Pts',(-30.8130689348788,81.3990007294873,
84.337517908959));
#214381=CARTESIAN_POINT('Ctrl Pts',(-30.7847585542864,80.2468455373728,
84.8903927636798));
#214382=CARTESIAN_POINT('Ctrl Pts',(-30.7755495903525,79.86098288616,85.0531347620494));
#214383=CARTESIAN_POINT('Ctrl Pts',(-30.7473449652769,78.6600270726954,
85.4926632164057));
#214384=CARTESIAN_POINT('Ctrl Pts',(-30.7280319465382,77.8247529729081,
85.7074159361789));
#214385=CARTESIAN_POINT('Ctrl Pts',(-30.6910603912866,76.1833097779639,
85.9596412280131));
#214386=CARTESIAN_POINT('Ctrl Pts',(-30.6735710441109,75.3826698359065,
86.0078825015437));
#214387=CARTESIAN_POINT('Ctrl Pts',(-30.6367612694799,73.723799707552,85.9546048289067));
#214388=CARTESIAN_POINT('Ctrl Pts',(-30.6174206737797,72.8697508673038,
85.8419244905332));
#214389=CARTESIAN_POINT('Ctrl Pts',(-30.5891203967703,71.625834320556,85.5503372772465));
#214390=CARTESIAN_POINT('Ctrl Pts',(-30.5799175548124,71.2234276662779,
85.4352731540193));
#214391=CARTESIAN_POINT('Ctrl Pts',(-30.5517158090505,70.0124310690293,
85.0248514265013));
#214392=CARTESIAN_POINT('Ctrl Pts',(-30.5323980990866,69.2270193158836,
84.6684830853844));
#214393=CARTESIAN_POINT('Ctrl Pts',(-30.4941887309648,67.7418127631924,
83.8079329876412));
#214394=CARTESIAN_POINT('Ctrl Pts',(-30.4755254322597,67.0452443059709,
83.3065849621175));
#214395=CARTESIAN_POINT('Ctrl Pts',(-30.4378741503665,65.7755713791571,
82.1872388125171));
#214396=CARTESIAN_POINT('Ctrl Pts',(-30.4190857000926,65.2029574684524,
81.5747899403001));
#214397=CARTESIAN_POINT('Ctrl Pts',(-30.3913648517823,64.4395602890922,
80.5816671073266));
#214398=CARTESIAN_POINT('Ctrl Pts',(-30.3822150418368,64.2019447331048,
80.2397626378297));
#214399=CARTESIAN_POINT('Ctrl Pts',(-30.3540427097426,63.5245441071243,
79.1577086904222));
#214400=CARTESIAN_POINT('Ctrl Pts',(-30.3346959136119,63.1414925942369,
78.384833382503));
#214401=CARTESIAN_POINT('Ctrl Pts',(-30.2969818153582,62.5426256359343,
76.7982985002516));
#214402=CARTESIAN_POINT('Ctrl Pts',(-30.2787732689618,62.3236428415581,
75.9901789180012));
#214403=CARTESIAN_POINT('Ctrl Pts',(-30.2508987994316,62.1138560264226,
74.7555711816159));
#214404=CARTESIAN_POINT('Ctrl Pts',(-30.241547686786,62.0638225373116,74.3413625467781));
#214405=CARTESIAN_POINT('Ctrl Pts',(-30.2108955544545,61.9649968470735,
72.9731955847784));
#214406=CARTESIAN_POINT('Ctrl Pts',(-30.1900135419002,62.0013269251022,
72.0162419579962));
#214407=CARTESIAN_POINT('Ctrl Pts',(-30.149811678117,62.2688678602672,70.2217270883568));
#214408=CARTESIAN_POINT('Ctrl Pts',(-30.1304569567233,62.4796377824916,
69.3861894619105));
#214409=CARTESIAN_POINT('Ctrl Pts',(-30.0987099752017,62.9657266805747,
68.0386905203795));
#214410=CARTESIAN_POINT('Ctrl Pts',(-30.0861499083022,63.1955356089743,
67.5132321762431));
#214411=CARTESIAN_POINT('Ctrl Pts',(-30.0641712084464,63.6527600071269,
66.6314639443198));
#214412=CARTESIAN_POINT('Ctrl Pts',(-30.0547676958645,63.8642552474804,
66.2678850765865));
#214413=CARTESIAN_POINT('Ctrl Pts',(-30.0178988288399,64.7609078072379,
64.8853263443044));
#214414=CARTESIAN_POINT('Ctrl Pts',(-29.9911962885626,65.5713348830826,
63.9552290855923));
#214415=CARTESIAN_POINT('Ctrl Pts',(-29.9545359336962,66.8151514200182,
62.880396375519));
#214416=CARTESIAN_POINT('Ctrl Pts',(-29.9451992868035,67.1431014367415,
62.6234408896241));
#214417=CARTESIAN_POINT('Ctrl Pts',(-29.9154777248646,68.2292233056485,
61.8536494978173));
#214418=CARTESIAN_POINT('Ctrl Pts',(-29.8954815089603,69.0293898410136,
61.4049008852747));
#214419=CARTESIAN_POINT('Ctrl Pts',(-29.8561491607125,70.6597401524625,
60.7047186172491));
#214420=CARTESIAN_POINT('Ctrl Pts',(-29.836800587082,71.4811624772142,60.4447076416566));
#214421=CARTESIAN_POINT('Ctrl Pts',(-29.8084773743039,72.7320732180116,
60.1813941330134));
#214422=CARTESIAN_POINT('Ctrl Pts',(-29.7992606631811,73.1458609453379,
60.1149779630723));
#214423=CARTESIAN_POINT('Ctrl Pts',(-29.7710526926903,74.4171129081448,
59.9735027293807));
#214424=CARTESIAN_POINT('Ctrl Pts',(-29.7517461979083,75.2794287901344,
59.9634544442968));
#214425=CARTESIAN_POINT('Ctrl Pts',(-29.7132365836367,77.0023514705184,
60.114641695641));
#214426=CARTESIAN_POINT('Ctrl Pts',(-29.6942902410553,77.8585081271593,
60.2772966406358));
#214427=CARTESIAN_POINT('Ctrl Pts',(-29.6656703653338,79.0919904728141,
60.642649394471));
#214428=CARTESIAN_POINT('Ctrl Pts',(-29.6563152116875,79.4860451648727,
60.7803093475951));
#214429=CARTESIAN_POINT('Ctrl Pts',(-29.6254462295597,80.7665405145654,
61.2980229125601));
#214430=CARTESIAN_POINT('Ctrl Pts',(-29.6043576289001,81.6173189050517,
61.7576637055568));
#214431=CARTESIAN_POINT('Ctrl Pts',(-29.565955471714,83.0415172632508,62.7455614485674));
#214432=CARTESIAN_POINT('Ctrl Pts',(-29.5486374992503,83.6334380938079,
63.2392476757865));
#214433=CARTESIAN_POINT('Ctrl Pts',(-29.5146922579461,84.715526424702,64.3180095817668));
#214434=CARTESIAN_POINT('Ctrl Pts',(-29.4981279757756,85.2049024155273,
64.8996638324907));
#214435=CARTESIAN_POINT('Ctrl Pts',(-29.4719894373469,85.880670516805,65.8625001577654));
#214436=CARTESIAN_POINT('Ctrl Pts',(-29.4626248789256,86.1039778442336,
66.2157003332167));
#214437=CARTESIAN_POINT('Ctrl Pts',(-29.4312913619077,86.7950129211955,
67.4350001219214));
#214438=CARTESIAN_POINT('Ctrl Pts',(-29.4097597523413,87.1813903963534,
68.3432747335166));
#214439=CARTESIAN_POINT('Ctrl Pts',(-29.3709189800937,87.6807751072625,
70.0240727435726));
#214440=CARTESIAN_POINT('Ctrl Pts',(-29.3535944272079,87.8340129956633,
70.7797482706167));
#214441=CARTESIAN_POINT('Ctrl Pts',(-29.3199808831717,88.0020982996774,
72.2832335622355));
#214442=CARTESIAN_POINT('Ctrl Pts',(-29.3037410645682,88.0211750548048,
73.0276616018292));
#214443=CARTESIAN_POINT('Ctrl Pts',(-29.2779607616765,87.9514273241659,
74.1869315593425));
#214444=CARTESIAN_POINT('Ctrl Pts',(-29.2685881002784,87.906204755505,74.6027829499671));
#214445=CARTESIAN_POINT('Ctrl Pts',(-29.2368855131641,87.6851712490229,
76.0031381799151));
#214446=CARTESIAN_POINT('Ctrl Pts',(-29.215001493764,87.4159475290683,76.9692793700861));
#214447=CARTESIAN_POINT('Ctrl Pts',(-29.1923989754345,87.0308162878128,
77.9143229035002));
#214448=CARTESIAN_POINT('Ctrl Pts',(-29.1919363963037,87.0228910310784,
77.933636806284));
#214449=CARTESIAN_POINT('Ctrl Pts',(-29.191473624437,87.0149197049505,77.9529305310098));
#214450=CARTESIAN_POINT('Ctrl Pts',(-30.6991941617974,87.0149197055719,
77.9529305295058));
#214451=CARTESIAN_POINT('Ctrl Pts',(-30.683487502314,86.7453849041422,78.6053100936136));
#214452=CARTESIAN_POINT('Ctrl Pts',(-30.6680646534442,86.423064275653,79.2348940782624));
#214453=CARTESIAN_POINT('Ctrl Pts',(-30.6351661800128,85.6414886819256,
80.496450934198));
#214454=CARTESIAN_POINT('Ctrl Pts',(-30.6176869597372,85.173438915591,81.119442347468));
#214455=CARTESIAN_POINT('Ctrl Pts',(-30.5812917504726,84.0769697870016,
82.3348469910265));
#214456=CARTESIAN_POINT('Ctrl Pts',(-30.5625565966655,83.4395720445536,
82.9142072901222));
#214457=CARTESIAN_POINT('Ctrl Pts',(-30.5341175409455,82.4141430219993,
83.675570097848));
#214458=CARTESIAN_POINT('Ctrl Pts',(-30.5247597961772,82.0667775703784,
83.9083818204726));
#214459=CARTESIAN_POINT('Ctrl Pts',(-30.4961757833556,80.9718250985024,
84.5680775450416));
#214460=CARTESIAN_POINT('Ctrl Pts',(-30.4773744419514,80.1925835798765,
84.9378379286018));
#214461=CARTESIAN_POINT('Ctrl Pts',(-30.4407631920138,78.63698675406,85.4948662864242));
#214462=CARTESIAN_POINT('Ctrl Pts',(-30.4229673875434,77.8685963057515,
85.6931514335049));
#214463=CARTESIAN_POINT('Ctrl Pts',(-30.3882077810994,76.3258553895781,
85.9440701974503));
#214464=CARTESIAN_POINT('Ctrl Pts',(-30.3713805720948,75.5552452569285,
85.9998966561579));
#214465=CARTESIAN_POINT('Ctrl Pts',(-30.3381954147479,74.0615379456218,
85.9751027001413));
#214466=CARTESIAN_POINT('Ctrl Pts',(-30.3219380215231,73.3410942776849,
85.9028536120454));
#214467=CARTESIAN_POINT('Ctrl Pts',(-30.2898766920788,71.9216513043095,
85.6397139236053));
#214468=CARTESIAN_POINT('Ctrl Pts',(-30.2741277391862,71.2250530960396,
85.4496026577302));
#214469=CARTESIAN_POINT('Ctrl Pts',(-30.2410058827312,69.8232952005922,
84.938634196457));
#214470=CARTESIAN_POINT('Ctrl Pts',(-30.2236501801234,69.1237157754223,
84.6105912010207));
#214471=CARTESIAN_POINT('Ctrl Pts',(-30.1889939369819,67.7735893450981,
83.8242530979093));
#214472=CARTESIAN_POINT('Ctrl Pts',(-30.1717043987259,67.1276141582225,
83.3644214827376));
#214473=CARTESIAN_POINT('Ctrl Pts',(-30.1349447442983,65.8748944413803,
82.2879618489353));
#214474=CARTESIAN_POINT('Ctrl Pts',(-30.1156198528478,65.2795974654932,
81.6638006618464));
#214475=CARTESIAN_POINT('Ctrl Pts',(-30.087423350035,64.4932999188011,80.6559535239909));
#214476=CARTESIAN_POINT('Ctrl Pts',(-30.0782309027133,64.2522932598192,
80.3142848457365));
#214477=CARTESIAN_POINT('Ctrl Pts',(-30.0499477074029,63.56729832787,79.2364185978482));
#214478=CARTESIAN_POINT('Ctrl Pts',(-30.030613679607,63.1794683809488,78.4673298951771));
#214479=CARTESIAN_POINT('Ctrl Pts',(-29.9943582613655,62.5915949928642,
76.9426142359236));
#214480=CARTESIAN_POINT('Ctrl Pts',(-29.9774277283934,62.3780308024885,
76.1961243240493));
#214481=CARTESIAN_POINT('Ctrl Pts',(-29.9410515613493,62.0703077754327,
74.5899724049097));
#214482=CARTESIAN_POINT('Ctrl Pts',(-29.9217091327139,61.992699412414,73.7308796678632));
#214483=CARTESIAN_POINT('Ctrl Pts',(-29.8935307167979,62.0043350551339,
72.4539048674676));
#214484=CARTESIAN_POINT('Ctrl Pts',(-29.8843706324115,62.0281484803234,
72.0377932588003));
#214485=CARTESIAN_POINT('Ctrl Pts',(-29.856652196523,62.1596741401908,70.7924099809308));
#214486=CARTESIAN_POINT('Ctrl Pts',(-29.8378757242906,62.3273948229381,
69.9716799211151));
#214487=CARTESIAN_POINT('Ctrl Pts',(-29.8008659262445,62.8159392159901,
68.3807326612484));
#214488=CARTESIAN_POINT('Ctrl Pts',(-29.7827974453274,63.1343099047363,
67.6137753764481));
#214489=CARTESIAN_POINT('Ctrl Pts',(-29.7452214016125,63.9276828070571,
66.1227272575466));
#214490=CARTESIAN_POINT('Ctrl Pts',(-29.725884467204,64.4062923013186,65.4051068112389));
#214491=CARTESIAN_POINT('Ctrl Pts',(-29.6976994255059,65.2168928217506,
64.4177329161527));
#214492=CARTESIAN_POINT('Ctrl Pts',(-29.6885278845024,65.4968615400463,
64.1083337423874));
#214493=CARTESIAN_POINT('Ctrl Pts',(-29.6608129838283,66.3805145173726,
63.2215199253372));
#214494=CARTESIAN_POINT('Ctrl Pts',(-29.6420508216541,67.0254128448869,
62.6882592610116));
#214495=CARTESIAN_POINT('Ctrl Pts',(-29.6057630221928,68.3775425608711,
61.773765084264));
#214496=CARTESIAN_POINT('Ctrl Pts',(-29.588363277267,69.0778239474529,61.388725890832));
#214497=CARTESIAN_POINT('Ctrl Pts',(-29.5534121047939,70.5190466965732,
60.7610142168751));
#214498=CARTESIAN_POINT('Ctrl Pts',(-29.5359768301,71.2553544349169,60.5158180731919));
#214499=CARTESIAN_POINT('Ctrl Pts',(-29.5059736898199,72.5750224054888,
60.2038333795925));
#214500=CARTESIAN_POINT('Ctrl Pts',(-29.4932246047683,73.1492892939941,
60.1081656105193));
#214501=CARTESIAN_POINT('Ctrl Pts',(-29.4612737528292,74.5836345257894,
59.967146809208));
#214502=CARTESIAN_POINT('Ctrl Pts',(-29.441913072983,75.4454771584534,59.968110292761));
#214503=CARTESIAN_POINT('Ctrl Pts',(-29.4005791665963,77.3024537657004,
60.1548729888451));
#214504=CARTESIAN_POINT('Ctrl Pts',(-29.3785386794421,78.2889343016288,
60.3715921653986));
#214505=CARTESIAN_POINT('Ctrl Pts',(-29.3466721202713,79.63589476985,60.8363819123887));
#214506=CARTESIAN_POINT('Ctrl Pts',(-29.337295744946,80.0244819828131,60.991825551247));
#214507=CARTESIAN_POINT('Ctrl Pts',(-29.3109609302171,81.1038978180587,
61.4852751765406));
#214508=CARTESIAN_POINT('Ctrl Pts',(-29.2941686238249,81.7731848908891,
61.8661791844435));
#214509=CARTESIAN_POINT('Ctrl Pts',(-29.2579408311842,83.1121287271607,
62.794097809553));
#214510=CARTESIAN_POINT('Ctrl Pts',(-29.2385928061241,83.7689585709696,
63.3532377044086));
#214511=CARTESIAN_POINT('Ctrl Pts',(-29.2104223409726,84.6542137681349,
64.27285767758));
#214512=CARTESIAN_POINT('Ctrl Pts',(-29.2012756477301,84.928162211407,64.5862322291635));
#214513=CARTESIAN_POINT('Ctrl Pts',(-29.1735542035811,85.7064522694633,
65.5678398967372));
#214514=CARTESIAN_POINT('Ctrl Pts',(-29.1547622732909,86.1617767551519,
66.2721327119445));
#214515=CARTESIAN_POINT('Ctrl Pts',(-29.116916366813,86.9435113337627,67.7831280194739));
#214516=CARTESIAN_POINT('Ctrl Pts',(-29.098072423964,87.2631860069253,68.5886973960785));
#214517=CARTESIAN_POINT('Ctrl Pts',(-29.0596713147632,87.7367018161264,
70.2472590047661));
#214518=CARTESIAN_POINT('Ctrl Pts',(-29.0403605782177,87.8901804322048,
71.0959102590723));
#214519=CARTESIAN_POINT('Ctrl Pts',(-29.0121546979943,87.9920446606397,
72.3707958832831));
#214520=CARTESIAN_POINT('Ctrl Pts',(-29.0029429272309,88.0052104471586,
72.7894780506037));
#214521=CARTESIAN_POINT('Ctrl Pts',(-28.9746279035492,87.983662591991,74.0673762813916));
#214522=CARTESIAN_POINT('Ctrl Pts',(-28.9552820635389,87.8839947534392,
74.9231335477672));
#214523=CARTESIAN_POINT('Ctrl Pts',(-28.9192277563573,87.5370075915119,
76.5118633438581));
#214524=CARTESIAN_POINT('Ctrl Pts',(-28.9024715747196,87.3075049584308,
77.2447598639295));
#214525=CARTESIAN_POINT('Ctrl Pts',(-28.8854250924613,87.0149197055719,
77.9529305295058));
#214526=CARTESIAN_POINT('Origin',(-21.6548258024609,75.,72.9888893865801));
#214527=CARTESIAN_POINT('',(-32.819270903196,87.0149197055719,77.9529305295058));
#214528=CARTESIAN_POINT('',(-32.5134098057851,87.0149197055719,77.9529305295058));
#214529=CARTESIAN_POINT('',(-21.6548258024609,87.0149197055719,77.9529305295058));
#214530=CARTESIAN_POINT('',(-31.8032572668915,65.6642719369909,63.9421119750625));
#214531=CARTESIAN_POINT('Ctrl Pts',(-31.8032572668915,65.6642719369909,
63.9421119750625));
#214532=CARTESIAN_POINT('Ctrl Pts',(-31.8135733380367,65.3385656683114,
64.2782211788701));
#214533=CARTESIAN_POINT('Ctrl Pts',(-31.8239028665893,65.0312489587717,
64.6316736406528));
#214534=CARTESIAN_POINT('Ctrl Pts',(-31.8446497618166,64.458312651216,65.3673088614644));
#214535=CARTESIAN_POINT('Ctrl Pts',(-31.8550507549726,64.1927991754078,
65.7487187740987));
#214536=CARTESIAN_POINT('Ctrl Pts',(-31.8857791041659,63.469068259206,66.9171692590297));
#214537=CARTESIAN_POINT('Ctrl Pts',(-31.9056269465411,63.0724313378894,
67.7390056154748));
#214538=CARTESIAN_POINT('Ctrl Pts',(-31.9423166756006,62.513779546848,69.294791851719));
#214539=CARTESIAN_POINT('Ctrl Pts',(-31.9590233980021,62.3230926914423,
70.0143187716436));
#214540=CARTESIAN_POINT('Ctrl Pts',(-31.9836814319382,62.1316498998252,
71.1073896767436));
#214541=CARTESIAN_POINT('Ctrl Pts',(-31.9917495291653,62.0836986306711,
71.4711162185924));
#214542=CARTESIAN_POINT('Ctrl Pts',(-32.0263623363712,61.9444997996125,
73.0350631533012));
#214543=CARTESIAN_POINT('Ctrl Pts',(-32.0533773329147,62.0047705901487,
74.2427715948304));
#214544=CARTESIAN_POINT('Ctrl Pts',(-32.0892096891712,62.3082996330555,
75.8339102814937));
#214545=CARTESIAN_POINT('Ctrl Pts',(-32.0983575985955,62.405937461001,76.2389650225414));
#214546=CARTESIAN_POINT('Ctrl Pts',(-32.1278230373569,62.780470583843,77.5193580315241));
#214547=CARTESIAN_POINT('Ctrl Pts',(-32.1484059703415,63.1306211086671,
78.3703268030057));
#214548=CARTESIAN_POINT('Ctrl Pts',(-32.1879520538945,63.9765823916936,
79.9331668466769));
#214549=CARTESIAN_POINT('Ctrl Pts',(-32.2066841825695,64.4596806333664,
80.6465912662357));
#214550=CARTESIAN_POINT('Ctrl Pts',(-32.2384146572364,65.3718995347885,
81.742186566815));
#214551=CARTESIAN_POINT('Ctrl Pts',(-32.2511214127918,65.7621942789836,
82.1531391066049));
#214552=CARTESIAN_POINT('Ctrl Pts',(-32.2731089279731,66.4867285575212,
82.8225484010837));
#214553=CARTESIAN_POINT('Ctrl Pts',(-32.2823645111182,66.8090751745151,
83.0926209277359));
#214554=CARTESIAN_POINT('Ctrl Pts',(-32.3186284223173,68.1198341268779,
84.0867981090575));
#214555=CARTESIAN_POINT('Ctrl Pts',(-32.3461123736615,69.1954616791803,
84.6853669253804));
#214556=CARTESIAN_POINT('Ctrl Pts',(-32.3824141307471,70.7275723256521,
85.2738289342571));
#214557=CARTESIAN_POINT('Ctrl Pts',(-32.3915615106238,71.1232226654734,
85.4043626424828));
#214558=CARTESIAN_POINT('Ctrl Pts',(-32.4209738567902,72.4063196478546,
85.7603565975389));
#214559=CARTESIAN_POINT('Ctrl Pts',(-32.441503262611,73.3115543342576,85.9112220916367));
#214560=CARTESIAN_POINT('Ctrl Pts',(-32.4789869647881,74.9930306227604,
86.0116302776272));
#214561=CARTESIAN_POINT('Ctrl Pts',(-32.4957723959841,75.7635232247348,
85.9892303391343));
#214562=CARTESIAN_POINT('Ctrl Pts',(-32.529097733169,77.2539602171473,85.8128823263586));
#214563=CARTESIAN_POINT('Ctrl Pts',(-32.5455487687377,77.9718656649989,
85.6657635364555));
#214564=CARTESIAN_POINT('Ctrl Pts',(-32.579135811788,79.4220603514326,85.2385520285343));
#214565=CARTESIAN_POINT('Ctrl Pts',(-32.5961693648489,80.1491790912049,
84.9511139013838));
#214566=CARTESIAN_POINT('Ctrl Pts',(-32.6268443157916,81.3816067348078,
84.3306056441482));
#214567=CARTESIAN_POINT('Ctrl Pts',(-32.6402975044144,81.8977977270893,
84.0242785943624));
#214568=CARTESIAN_POINT('Ctrl Pts',(-32.6630465611979,82.7370776852665,
83.4442518058244));
#214569=CARTESIAN_POINT('Ctrl Pts',(-32.6723157786034,83.0713407117878,
83.1884204480479));
#214570=CARTESIAN_POINT('Ctrl Pts',(-32.7088655896348,84.3376510901744,
82.1179418422261));
#214571=CARTESIAN_POINT('Ctrl Pts',(-32.7366253494161,85.1637971527023,
81.1881909555477));
#214572=CARTESIAN_POINT('Ctrl Pts',(-32.773203608357,86.0755540950393,79.8083810977813));
#214573=CARTESIAN_POINT('Ctrl Pts',(-32.782350752454,86.2882775758034,79.4501706690866));
#214574=CARTESIAN_POINT('Ctrl Pts',(-32.8007507006903,86.6787198769651,
78.7143643607418));
#214575=CARTESIAN_POINT('Ctrl Pts',(-32.8099869769191,86.8560578530742,
78.3374383019199));
#214576=CARTESIAN_POINT('Ctrl Pts',(-32.819270903196,87.0149197055719,77.9529305295058));
#214577=CARTESIAN_POINT('Ctrl Pts',(-31.8032546359729,65.6642718921576,
63.9421120213278));
#214578=CARTESIAN_POINT('Ctrl Pts',(-31.7842284681536,66.2560091425745,
63.3314749007115));
#214579=CARTESIAN_POINT('Ctrl Pts',(-31.7654238551895,66.9062344712278,
62.7803635629509));
#214580=CARTESIAN_POINT('Ctrl Pts',(-31.728504118784,68.2838663363805,61.8276341158955));
#214581=CARTESIAN_POINT('Ctrl Pts',(-31.7100617480658,69.0052280770819,
61.4241685258146));
#214582=CARTESIAN_POINT('Ctrl Pts',(-31.6718429273203,70.5729452195354,
60.7336692325463));
#214583=CARTESIAN_POINT('Ctrl Pts',(-31.6524317557486,71.4205314357544,
60.4598578773549));
#214584=CARTESIAN_POINT('Ctrl Pts',(-31.6136746885707,73.1298798352618,
60.095434315327));
#214585=CARTESIAN_POINT('Ctrl Pts',(-31.5943314241114,73.986071048588,60.000029197985));
#214586=CARTESIAN_POINT('Ctrl Pts',(-31.562881818816,75.4056682551647,59.9831450953161));
#214587=CARTESIAN_POINT('Ctrl Pts',(-31.5505969704306,75.9657858978662,
60.0127109359883));
#214588=CARTESIAN_POINT('Ctrl Pts',(-31.5210871038211,77.2900265256507,
60.1688478647222));
#214589=CARTESIAN_POINT('Ctrl Pts',(-31.5036829091261,78.0482033068846,
60.3276833323172));
#214590=CARTESIAN_POINT('Ctrl Pts',(-31.4673980769323,79.6096046724077,
60.8032570735867));
#214591=CARTESIAN_POINT('Ctrl Pts',(-31.4486815423165,80.404613767649,61.1344286833351));
#214592=CARTESIAN_POINT('Ctrl Pts',(-31.4202443593273,81.527856597147,61.7389763999586));
#214593=CARTESIAN_POINT('Ctrl Pts',(-31.410905144574,81.8848939385131,61.953868331928));
#214594=CARTESIAN_POINT('Ctrl Pts',(-31.3809917514735,82.9981248456975,
62.6989855387059));
#214595=CARTESIAN_POINT('Ctrl Pts',(-31.3608129843137,83.708379801769,63.2926924838235));
#214596=CARTESIAN_POINT('Ctrl Pts',(-31.3310663415844,84.6408211138014,
64.2579053239863));
#214597=CARTESIAN_POINT('Ctrl Pts',(-31.3216800837528,84.9171638610513,
64.573108212071));
#214598=CARTESIAN_POINT('Ctrl Pts',(-31.2936664521116,85.6963073046544,
65.5535948162585));
#214599=CARTESIAN_POINT('Ctrl Pts',(-31.2752613335763,86.1508664949386,
66.2544421967027));
#214600=CARTESIAN_POINT('Ctrl Pts',(-31.2389086390138,86.9112415809572,
67.7175257133276));
#214601=CARTESIAN_POINT('Ctrl Pts',(-31.2206515149041,87.2183687057085,
68.4748661687591));
#214602=CARTESIAN_POINT('Ctrl Pts',(-31.1828793143346,87.7046520773152,
70.0970395384582));
#214603=CARTESIAN_POINT('Ctrl Pts',(-31.1636970411606,87.8709224718629,
70.9614956475302));
#214604=CARTESIAN_POINT('Ctrl Pts',(-31.1349413547196,87.9859043416946,
72.2530214836414));
#214605=CARTESIAN_POINT('Ctrl Pts',(-31.1255602693797,88.0028642364736,
72.6715053387859));
#214606=CARTESIAN_POINT('Ctrl Pts',(-31.0934877823317,87.9917030279652,
74.10542105164));
#214607=CARTESIAN_POINT('Ctrl Pts',(-31.0712508455816,87.8648704341448,
75.1163507153663));
#214608=CARTESIAN_POINT('Ctrl Pts',(-31.03947192201,87.5212073175799,76.5096092073126));
#214609=CARTESIAN_POINT('Ctrl Pts',(-31.0300766281358,87.4010408798071,
76.9119344551807));
#214610=CARTESIAN_POINT('Ctrl Pts',(-31.0155341825007,87.1850859522539,
77.5250511349386));
#214611=CARTESIAN_POINT('Ctrl Pts',(-31.0103872385355,87.1028154818789,
77.7401883977667));
#214612=CARTESIAN_POINT('Ctrl Pts',(-31.0052564152503,87.0149197055719,
77.9529305295058));
#214613=CARTESIAN_POINT('Ctrl Pts',(-32.5134098057851,87.0149197055719,
77.9529305295058));
#214614=CARTESIAN_POINT('Ctrl Pts',(-32.5075997933644,86.9146418918773,
78.1956420311034));
#214615=CARTESIAN_POINT('Ctrl Pts',(-32.5017690584973,86.8069826178028,
78.4353803885588));
#214616=CARTESIAN_POINT('Ctrl Pts',(-32.4838109340488,86.4545420879065,
79.1604936379299));
#214617=CARTESIAN_POINT('Ctrl Pts',(-32.4716151683794,86.1866124201152,
79.6338073004822));
#214618=CARTESIAN_POINT('Ctrl Pts',(-32.4423112173233,85.4683690181421,
80.7354249903596));
#214619=CARTESIAN_POINT('Ctrl Pts',(-32.4254745688282,84.9901551749687,
81.3430718605348));
#214620=CARTESIAN_POINT('Ctrl Pts',(-32.3909691756996,83.9235056915968,
82.4749303419633));
#214621=CARTESIAN_POINT('Ctrl Pts',(-32.3733384476991,83.3356814762439,
82.9954039613138));
#214622=CARTESIAN_POINT('Ctrl Pts',(-32.337430403783,82.0324512357819,83.9543344917921));
#214623=CARTESIAN_POINT('Ctrl Pts',(-32.3192085828059,81.3142562951554,
84.3830340939489));
#214624=CARTESIAN_POINT('Ctrl Pts',(-32.2913278650799,80.1827923149245,
84.9183801317905));
#214625=CARTESIAN_POINT('Ctrl Pts',(-32.2819836082309,79.797270011951,85.0785661809406));
#214626=CARTESIAN_POINT('Ctrl Pts',(-32.2534186544639,78.5951583303169,
85.5114776060869));
#214627=CARTESIAN_POINT('Ctrl Pts',(-32.2346255300043,77.758655028736,85.721925287822));
#214628=CARTESIAN_POINT('Ctrl Pts',(-32.1970950751662,76.0836806853654,
85.9703866976567));
#214629=CARTESIAN_POINT('Ctrl Pts',(-32.1783506117603,75.2500110699179,
86.0131407334634));
#214630=CARTESIAN_POINT('Ctrl Pts',(-32.1413371328631,73.5829692638462,
85.9384339552752));
#214631=CARTESIAN_POINT('Ctrl Pts',(-32.1230771433696,72.7534880564385,
85.8205639948546));
#214632=CARTESIAN_POINT('Ctrl Pts',(-32.0951735876016,71.5362867104418,
85.5258807657098));
#214633=CARTESIAN_POINT('Ctrl Pts',(-32.0858442209667,71.1364359369947,
85.4084841601795));
#214634=CARTESIAN_POINT('Ctrl Pts',(-32.0573009838373,69.9298848928574,
84.9903203794736));
#214635=CARTESIAN_POINT('Ctrl Pts',(-32.0385161603638,69.1468406483531,
84.6285173885043));
#214636=CARTESIAN_POINT('Ctrl Pts',(-32.0003874137635,67.6647780431255,
83.7561040859797));
#214637=CARTESIAN_POINT('Ctrl Pts',(-31.9810358762197,66.9692967255576,
83.2478463122074));
#214638=CARTESIAN_POINT('Ctrl Pts',(-31.9434039408314,65.7031284230795,
82.1143467604991));
#214639=CARTESIAN_POINT('Ctrl Pts',(-31.9250222758533,65.1329804070874,
81.4946358664839));
#214640=CARTESIAN_POINT('Ctrl Pts',(-31.8913006292345,64.2216681034031,
80.288134727132));
#214641=CARTESIAN_POINT('Ctrl Pts',(-31.8762028233835,63.858882935033,79.7214178144745));
#214642=CARTESIAN_POINT('Ctrl Pts',(-31.8521448114598,63.3449044615873,
78.7622803770684));
#214643=CARTESIAN_POINT('Ctrl Pts',(-31.8429988603328,63.1660163439334,
78.3861226572369));
#214644=CARTESIAN_POINT('Ctrl Pts',(-31.8138208557924,62.6567570514172,
77.1676617000098));
#214645=CARTESIAN_POINT('Ctrl Pts',(-31.7935292548616,62.396043768211,76.2991841604238));
#214646=CARTESIAN_POINT('Ctrl Pts',(-31.7542863072485,62.0674673988842,
74.5663088062888));
#214647=CARTESIAN_POINT('Ctrl Pts',(-31.7355537963974,61.9914880216104,
73.7081064929883));
#214648=CARTESIAN_POINT('Ctrl Pts',(-31.7071035349279,62.0052709553146,
72.4300220550393));
#214649=CARTESIAN_POINT('Ctrl Pts',(-31.6977308382133,62.0300109726611,
72.0118023620038));
#214650=CARTESIAN_POINT('Ctrl Pts',(-31.6691269703002,62.1670970869241,
70.7401805414656));
#214651=CARTESIAN_POINT('Ctrl Pts',(-31.6503159240616,62.3439801615891,
69.8961150526805));
#214652=CARTESIAN_POINT('Ctrl Pts',(-31.6120805004828,62.8636003199811,
68.2499355214424));
#214653=CARTESIAN_POINT('Ctrl Pts',(-31.5925892083222,63.2061228202923,
67.4522537560806));
#214654=CARTESIAN_POINT('Ctrl Pts',(-31.5548346716221,64.030534095666,65.9624416214482));
#214655=CARTESIAN_POINT('Ctrl Pts',(-31.5365502063061,64.5054110851407,
65.2711331158504));
#214656=CARTESIAN_POINT('Ctrl Pts',(-31.5086330122316,65.3108801702628,
64.3116782590005));
#214657=CARTESIAN_POINT('Ctrl Pts',(-31.4993139962588,65.5934778173574,
64.006107216035));
#214658=CARTESIAN_POINT('Ctrl Pts',(-31.4707861181307,66.5041026698939,
63.1116356769772));
#214659=CARTESIAN_POINT('Ctrl Pts',(-31.4520065855794,67.1763190514444,
62.5710954819328));
#214660=CARTESIAN_POINT('Ctrl Pts',(-31.4150123669398,68.5735484664381,
61.6595800493482));
#214661=CARTESIAN_POINT('Ctrl Pts',(-31.3968335965468,69.2897667003974,
61.2822349691715));
#214662=CARTESIAN_POINT('Ctrl Pts',(-31.3603815292869,70.8082550101268,
60.6549203508464));
#214663=CARTESIAN_POINT('Ctrl Pts',(-31.3421407074077,71.6090923015082,
60.4111601719133));
#214664=CARTESIAN_POINT('Ctrl Pts',(-31.3142483905366,72.8363906628502,
60.163423457877));
#214665=CARTESIAN_POINT('Ctrl Pts',(-31.3049113628243,73.2487508542692,
60.1006425291059));
#214666=CARTESIAN_POINT('Ctrl Pts',(-31.2763568850329,74.5193177389937,
59.9693138810174));
#214667=CARTESIAN_POINT('Ctrl Pts',(-31.2575678935881,75.3818940328471,
59.966041762369));
#214668=CARTESIAN_POINT('Ctrl Pts',(-31.2212335515245,77.0135281432915,
60.1221898690667));
#214669=CARTESIAN_POINT('Ctrl Pts',(-31.2037330433807,77.7803744388936,
60.2658489075672));
#214670=CARTESIAN_POINT('Ctrl Pts',(-31.1673159196836,79.3567104591316,
60.7105594778463));
#214671=CARTESIAN_POINT('Ctrl Pts',(-31.1485808358536,80.1585174025768,
61.0252771705167));
#214672=CARTESIAN_POINT('Ctrl Pts',(-31.1201415347332,81.2954281594925,
61.6072260922669));
#214673=CARTESIAN_POINT('Ctrl Pts',(-31.1107834729899,81.6580632094587,
61.8154893569849));
#214674=CARTESIAN_POINT('Ctrl Pts',(-31.0821990223593,82.734626612722,62.5048137631266));
#214675=CARTESIAN_POINT('Ctrl Pts',(-31.0633974804975,83.4113707080935,
63.0395609964287));
#214676=CARTESIAN_POINT('Ctrl Pts',(-31.0255413687474,84.6404053738881,
64.2263624082217));
#214677=CARTESIAN_POINT('Ctrl Pts',(-31.0064524825665,85.191385486151,64.8737831658655));
#214678=CARTESIAN_POINT('Ctrl Pts',(-30.9690972308968,86.1526095639457,
66.2569751945058));
#214679=CARTESIAN_POINT('Ctrl Pts',(-30.9508258171705,86.5624697843879,
66.9881669713929));
#214680=CARTESIAN_POINT('Ctrl Pts',(-30.9229157932786,87.0668817808325,
68.13465099886));
#214681=CARTESIAN_POINT('Ctrl Pts',(-30.9135911763968,87.2161150735975,
68.5234893164158));
#214682=CARTESIAN_POINT('Ctrl Pts',(-30.8850549657918,87.6158356070293,
69.7360280810617));
#214683=CARTESIAN_POINT('Ctrl Pts',(-30.8662726181079,87.8034327564835,
70.5779713807514));
#214684=CARTESIAN_POINT('Ctrl Pts',(-30.8291649364347,88.0038269288232,
72.2394920522822));
#214685=CARTESIAN_POINT('Ctrl Pts',(-30.8108665953109,88.0252391035558,
73.0540816277721));
#214686=CARTESIAN_POINT('Ctrl Pts',(-30.7742958530402,87.9141078888471,
74.6987386374438));
#214687=CARTESIAN_POINT('Ctrl Pts',(-30.7560509419293,87.7775952862349,
75.5247984171261));
#214688=CARTESIAN_POINT('Ctrl Pts',(-30.7281561876402,87.4555936971577,
76.7348072049893));
#214689=CARTESIAN_POINT('Ctrl Pts',(-30.7188207626934,87.3291018834203,
77.1321924632432));
#214690=CARTESIAN_POINT('Ctrl Pts',(-30.7060591949955,87.1300003055977,
77.6672262756005));
#214691=CARTESIAN_POINT('Ctrl Pts',(-30.7026204048056,87.073715895164,77.8106207708631));
#214692=CARTESIAN_POINT('Ctrl Pts',(-30.6991941617974,87.0149197055719,
77.9529305295058));
#214693=CARTESIAN_POINT('Origin',(-21.6548258024609,75.,72.9888893865801));
#214694=CARTESIAN_POINT('',(-34.6333744106366,87.0149197055719,77.9529305295058));
#214695=CARTESIAN_POINT('',(-34.3273949797549,87.0149197055719,77.9529305295058));
#214696=CARTESIAN_POINT('',(-21.6548258024609,87.0149197055719,77.9529305295058));
#214697=CARTESIAN_POINT('Ctrl Pts',(-32.819270903196,87.0149197055719,77.9529305295058));
#214698=CARTESIAN_POINT('Ctrl Pts',(-32.8303492893789,87.2044874487043,
77.4941025007035));
#214699=CARTESIAN_POINT('Ctrl Pts',(-32.8415001971829,87.3677464596969,
77.0244787448557));
#214700=CARTESIAN_POINT('Ctrl Pts',(-32.8618829569116,87.6184066977144,
76.1434512817156));
#214701=CARTESIAN_POINT('Ctrl Pts',(-32.8710927370109,87.7134904735021,
75.7352704421921));
#214702=CARTESIAN_POINT('Ctrl Pts',(-32.9028840772483,87.9724059114136,
74.3167894059358));
#214703=CARTESIAN_POINT('Ctrl Pts',(-32.925752002725,88.0366642288654,73.2921902487054));
#214704=CARTESIAN_POINT('Ctrl Pts',(-32.9578897961531,87.9569617157058,
71.8516619677294));
#214705=CARTESIAN_POINT('Ctrl Pts',(-32.9671257230642,87.9134966956485,
71.4339789389983));
#214706=CARTESIAN_POINT('Ctrl Pts',(-32.9948122310079,87.7231975056415,
70.1925447133568));
#214707=CARTESIAN_POINT('Ctrl Pts',(-33.0133770239326,87.5170292474647,
69.3801132161319));
#214708=CARTESIAN_POINT('Ctrl Pts',(-33.050347567485,86.9582785244051,67.8249971947681));
#214709=CARTESIAN_POINT('Ctrl Pts',(-33.0682711390013,86.6105575235084,
67.0845548514814));
#214710=CARTESIAN_POINT('Ctrl Pts',(-33.1060395069239,85.74201255568,65.6128453231014));
#214711=CARTESIAN_POINT('Ctrl Pts',(-33.1260757975856,85.2103360810908,
64.8928485371945));
#214712=CARTESIAN_POINT('Ctrl Pts',(-33.1650533361119,84.0302700332628,
63.5977869024856));
#214713=CARTESIAN_POINT('Ctrl Pts',(-33.1837862547422,83.3898671157429,
63.0215066535477));
#214714=CARTESIAN_POINT('Ctrl Pts',(-33.2122343752409,82.360001722789,62.2648248635988));
#214715=CARTESIAN_POINT('Ctrl Pts',(-33.2216041277003,82.0109346076854,
62.0334350381732));
#214716=CARTESIAN_POINT('Ctrl Pts',(-33.2502042439525,80.9121335321621,
61.3791168043054));
#214717=CARTESIAN_POINT('Ctrl Pts',(-33.2690133538773,80.1310797993482,
61.0134075639596));
#214718=CARTESIAN_POINT('Ctrl Pts',(-33.3071691420166,78.5064325375152,
60.4410479395259));
#214719=CARTESIAN_POINT('Ctrl Pts',(-33.326575808564,77.6667357252942,60.2361678403155));
#214720=CARTESIAN_POINT('Ctrl Pts',(-33.364246377408,75.9844855781902,59.999248268048));
#214721=CARTESIAN_POINT('Ctrl Pts',(-33.38252812792,75.1466759776841,59.9628200488981));
#214722=CARTESIAN_POINT('Ctrl Pts',(-33.4104438502265,73.895743675265,60.0291940811623));
#214723=CARTESIAN_POINT('Ctrl Pts',(-33.4197640468687,73.4815917907657,
60.0711682248313));
#214724=CARTESIAN_POINT('Ctrl Pts',(-33.4482936853185,72.2192296161529,
60.2606636956289));
#214725=CARTESIAN_POINT('Ctrl Pts',(-33.4670738020269,71.3830744700052,
60.4725694786873));
#214726=CARTESIAN_POINT('Ctrl Pts',(-33.5040917059498,69.8134338164243,
61.0409252526616));
#214727=CARTESIAN_POINT('Ctrl Pts',(-33.522295431567,69.0802262856134,61.3867090959163));
#214728=CARTESIAN_POINT('Ctrl Pts',(-33.5587722675796,67.664970945732,62.2234391375012));
#214729=CARTESIAN_POINT('Ctrl Pts',(-33.5770139445228,66.9886507511057,
62.7167979507159));
#214730=CARTESIAN_POINT('Ctrl Pts',(-33.6049067728145,66.0527525540762,
63.548522294637));
#214731=CARTESIAN_POINT('Ctrl Pts',(-33.6142434667843,65.7546604683032,
63.8402575975047));
#214732=CARTESIAN_POINT('Ctrl Pts',(-33.6427974576095,64.8857802564834,
64.7765230099947));
#214733=CARTESIAN_POINT('Ctrl Pts',(-33.6615862629468,64.3645242570598,
65.4637940548586));
#214734=CARTESIAN_POINT('Ctrl Pts',(-33.6989489141149,63.4840134475982,
66.9009771068278));
#214735=CARTESIAN_POINT('Ctrl Pts',(-33.7175161861705,63.1209666569287,
67.6438747452044));
#214736=CARTESIAN_POINT('Ctrl Pts',(-33.7543538258173,62.5368341013194,
69.1983991292577));
#214737=CARTESIAN_POINT('Ctrl Pts',(-33.7726078614505,62.3190020832833,
70.0071749283648));
#214738=CARTESIAN_POINT('Ctrl Pts',(-33.8005079772522,62.1111595771066,
71.2420763958167));
#214739=CARTESIAN_POINT('Ctrl Pts',(-33.8098397642832,62.0618026721878,
71.6559932981437));
#214740=CARTESIAN_POINT('Ctrl Pts',(-33.8383865660572,61.9716873813061,
72.9298889535711));
#214741=CARTESIAN_POINT('Ctrl Pts',(-33.8571726828789,61.9963379837603,
73.7921242859579));
#214742=CARTESIAN_POINT('Ctrl Pts',(-33.8952999633214,62.2155039798007,
75.4978903519339));
#214743=CARTESIAN_POINT('Ctrl Pts',(-33.9146515593895,62.4092514119537,
76.3372431241239));
#214744=CARTESIAN_POINT('Ctrl Pts',(-33.952282593488,62.9533283389689,77.9470330552479));
#214745=CARTESIAN_POINT('Ctrl Pts',(-33.9706588100548,63.2987482786594,
78.7148129343067));
#214746=CARTESIAN_POINT('Ctrl Pts',(-34.0044349703634,64.05076051187,80.0294294318639));
#214747=CARTESIAN_POINT('Ctrl Pts',(-34.0195937255112,64.4307815671972,
80.5880129367791));
#214748=CARTESIAN_POINT('Ctrl Pts',(-34.043710710607,65.1126285388131,81.4395211765081));
#214749=CARTESIAN_POINT('Ctrl Pts',(-34.0528566123954,65.3882857390685,
81.7517794139277));
#214750=CARTESIAN_POINT('Ctrl Pts',(-34.0820230583186,66.3084077888566,
82.6983197802078));
#214751=CARTESIAN_POINT('Ctrl Pts',(-34.1023028968185,67.0042272195077,
83.2789045014865));
#214752=CARTESIAN_POINT('Ctrl Pts',(-34.1415336101932,68.4681981288636,
84.2616092321369));
#214753=CARTESIAN_POINT('Ctrl Pts',(-34.1602661381447,69.2275293085514,
84.6686683300158));
#214754=CARTESIAN_POINT('Ctrl Pts',(-34.1887163038381,70.4082368105509,
85.1581547938577));
#214755=CARTESIAN_POINT('Ctrl Pts',(-34.1980888677721,70.802536777373,85.299722462373));
#214756=CARTESIAN_POINT('Ctrl Pts',(-34.2266925686778,72.0257499581929,
85.6732864135495));
#214757=CARTESIAN_POINT('Ctrl Pts',(-34.2455035276184,72.8714346049849,
85.8422664987384));
#214758=CARTESIAN_POINT('Ctrl Pts',(-34.2837353197547,74.5892192478275,
86.0112103592344));
#214759=CARTESIAN_POINT('Ctrl Pts',(-34.3032227509619,75.4571569903084,
86.0096644762231));
#214760=CARTESIAN_POINT('Ctrl Pts',(-34.3409734567283,77.1509044130273,
85.8369924861105));
#214761=CARTESIAN_POINT('Ctrl Pts',(-34.3592577985572,77.9732010418807,
85.6719578852339));
#214762=CARTESIAN_POINT('Ctrl Pts',(-34.387174925913,79.1719815355225,85.3082890595779));
#214763=CARTESIAN_POINT('Ctrl Pts',(-34.396493995771,79.5640204239145,85.1684934390129));
#214764=CARTESIAN_POINT('Ctrl Pts',(-34.4250219542817,80.7443686519268,
84.6825903029927));
#214765=CARTESIAN_POINT('Ctrl Pts',(-34.4438015133866,81.5055714903305,
84.2768454927081));
#214766=CARTESIAN_POINT('Ctrl Pts',(-34.4799213390596,82.8600103940223,
83.3720786412212));
#214767=CARTESIAN_POINT('Ctrl Pts',(-34.4971936814308,83.4598341179283,
82.8894741619705));
#214768=CARTESIAN_POINT('Ctrl Pts',(-34.533375927297,84.6326601303735,81.7610094245599));
#214769=CARTESIAN_POINT('Ctrl Pts',(-34.5521118107011,85.1912236252756,
81.1053664772444));
#214770=CARTESIAN_POINT('Ctrl Pts',(-34.5805483990319,85.9191496652819,
80.0561870100941));
#214771=CARTESIAN_POINT('Ctrl Pts',(-34.5899029774701,86.1406073486229,
79.7016676415927));
#214772=CARTESIAN_POINT('Ctrl Pts',(-34.6107233525499,86.5953149174206,
78.8890800648757));
#214773=CARTESIAN_POINT('Ctrl Pts',(-34.6220712822385,86.8191104022253,
78.4268655734703));
#214774=CARTESIAN_POINT('Ctrl Pts',(-34.6333744106366,87.0149197055719,
77.9529305295058));
#214775=CARTESIAN_POINT('',(-33.3112169404745,65.6642757110361,63.9421080804774));
#214776=CARTESIAN_POINT('Ctrl Pts',(-33.3112143094266,65.6642756705897,
63.9421081222156));
#214777=CARTESIAN_POINT('Ctrl Pts',(-33.3011530209772,65.9819378957081,
63.6143001563865));
#214778=CARTESIAN_POINT('Ctrl Pts',(-33.2910793698672,66.3166445043513,
63.3034516989295));
#214779=CARTESIAN_POINT('Ctrl Pts',(-33.2708446150653,67.0148633494904,
62.7203455116794));
#214780=CARTESIAN_POINT('Ctrl Pts',(-33.2606986075489,67.3776751568669,
62.4482270281143));
#214781=CARTESIAN_POINT('Ctrl Pts',(-33.2307671604748,68.488845839857,61.7022445712945));
#214782=CARTESIAN_POINT('Ctrl Pts',(-33.2114320471333,69.2722075581934,
61.2852200541596));
#214783=CARTESIAN_POINT('Ctrl Pts',(-33.1787503430636,70.6373979198212,
60.7285952391906));
#214784=CARTESIAN_POINT('Ctrl Pts',(-33.1655723528332,71.197443039727,60.54350207004));
#214785=CARTESIAN_POINT('Ctrl Pts',(-33.133160570118,72.6015034113583,60.1831278966833));
#214786=CARTESIAN_POINT('Ctrl Pts',(-33.114359740488,73.4540839038891,60.0524888559181));
#214787=CARTESIAN_POINT('Ctrl Pts',(-33.0777586365687,75.1036139273006,
59.9652335843315));
#214788=CARTESIAN_POINT('Ctrl Pts',(-33.0599736298245,75.8960926133116,
59.9956853011575));
#214789=CARTESIAN_POINT('Ctrl Pts',(-33.0252192077184,77.4457428445872,
60.197746707406));
#214790=CARTESIAN_POINT('Ctrl Pts',(-33.0083865484756,78.2002310484827,
60.3653591569273));
#214791=CARTESIAN_POINT('Ctrl Pts',(-32.9752391164359,79.6224206619558,
60.8170839334507));
#214792=CARTESIAN_POINT('Ctrl Pts',(-32.9590265762345,80.2901020089395,
61.092064837245));
#214793=CARTESIAN_POINT('Ctrl Pts',(-32.9255873095396,81.6297955898788,
61.7790023735103));
#214794=CARTESIAN_POINT('Ctrl Pts',(-32.9084557450833,82.2942060404131,
62.1995277917367));
#214795=CARTESIAN_POINT('Ctrl Pts',(-32.8778314769896,83.3865938986748,
63.0382061924307));
#214796=CARTESIAN_POINT('Ctrl Pts',(-32.8645353439765,83.8313399736833,
63.4307261721247));
#214797=CARTESIAN_POINT('Ctrl Pts',(-32.8340356118969,84.7927287577772,
64.4038026238821));
#214798=CARTESIAN_POINT('Ctrl Pts',(-32.8171172936067,85.2872556168821,
65.0030504225077));
#214799=CARTESIAN_POINT('Ctrl Pts',(-32.7829672966371,86.1573694942003,
66.2734299318871));
#214800=CARTESIAN_POINT('Ctrl Pts',(-32.7657834393555,86.5328486269691,
66.9409407885883));
#214801=CARTESIAN_POINT('Ctrl Pts',(-32.7296922896985,87.2011752105809,
68.4205721579918));
#214802=CARTESIAN_POINT('Ctrl Pts',(-32.7109560648433,87.4763561162233,
69.236723973125));
#214803=CARTESIAN_POINT('Ctrl Pts',(-32.6795826241964,87.7922379270936,
70.6096609682824));
#214804=CARTESIAN_POINT('Ctrl Pts',(-32.6672464094614,87.8813806697013,
71.1525590898731));
#214805=CARTESIAN_POINT('Ctrl Pts',(-32.6377909529484,88.0124818817826,
72.4678051521302));
#214806=CARTESIAN_POINT('Ctrl Pts',(-32.6209450117024,88.0204620489175,
73.2414421537243));
#214807=CARTESIAN_POINT('Ctrl Pts',(-32.5863770461848,87.8979292100688,
74.7947794161168));
#214808=CARTESIAN_POINT('Ctrl Pts',(-32.5686903127928,87.7651796837949,
75.5711359094499));
#214809=CARTESIAN_POINT('Ctrl Pts',(-32.5385603550143,87.4161659902799,
76.8831980345399));
#214810=CARTESIAN_POINT('Ctrl Pts',(-32.5260450915273,87.2329982117584,
77.4250953110014));
#214811=CARTESIAN_POINT('Ctrl Pts',(-32.5134098057851,87.0149197055719,
77.9529305295058));
#214812=CARTESIAN_POINT('Ctrl Pts',(-34.3273949797549,87.0149197055719,
77.9529305295058));
#214813=CARTESIAN_POINT('Ctrl Pts',(-34.3222659641844,86.9262956441725,
78.1674353958109));
#214814=CARTESIAN_POINT('Ctrl Pts',(-34.3171225529525,86.8319053648498,
78.3796197710729));
#214815=CARTESIAN_POINT('Ctrl Pts',(-34.2948046279984,86.3993570431063,
79.2857375148203));
#214816=CARTESIAN_POINT('Ctrl Pts',(-34.277429777375,86.0055155106241,79.9512358991139));
#214817=CARTESIAN_POINT('Ctrl Pts',(-34.2483014228856,85.2373570206595,
81.0196149185656));
#214818=CARTESIAN_POINT('Ctrl Pts',(-34.2363710132047,84.892316512885,81.4409960525426));
#214819=CARTESIAN_POINT('Ctrl Pts',(-34.2058500439899,83.9537884077597,
82.4507056320329));
#214820=CARTESIAN_POINT('Ctrl Pts',(-34.1870952982888,83.3281615847613,
83.0057752951113));
#214821=CARTESIAN_POINT('Ctrl Pts',(-34.1511658409779,82.0215106026655,
83.9574819248889));
#214822=CARTESIAN_POINT('Ctrl Pts',(-34.1340977716159,81.3490863657803,
84.3599378215143));
#214823=CARTESIAN_POINT('Ctrl Pts',(-34.099566968348,79.9496049205403,85.0344950070419));
#214824=CARTESIAN_POINT('Ctrl Pts',(-34.082198363434,79.2261880694725,85.306946908301));
#214825=CARTESIAN_POINT('Ctrl Pts',(-34.0531702411385,77.9628688572581,
85.6582519546531));
#214826=CARTESIAN_POINT('Ctrl Pts',(-34.0413343931215,77.4343400645138,
85.770334138519));
#214827=CARTESIAN_POINT('Ctrl Pts',(-34.0108988120774,76.0742343351886,
85.971317396461));
#214828=CARTESIAN_POINT('Ctrl Pts',(-33.9921328797055,75.2382530569122,
86.0135059638339));
#214829=CARTESIAN_POINT('Ctrl Pts',(-33.9556588893021,73.5993996063151,
85.9382949619383));
#214830=CARTESIAN_POINT('Ctrl Pts',(-33.9380867492596,72.7999443211295,
85.8266675374436));
#214831=CARTESIAN_POINT('Ctrl Pts',(-33.9010405308774,71.1784818734973,
85.444265901033));
#214832=CARTESIAN_POINT('Ctrl Pts',(-33.8816911855315,70.362662397949,85.1640901963068));
#214833=CARTESIAN_POINT('Ctrl Pts',(-33.8535228001869,69.2025344330137,
84.6320128779897));
#214834=CARTESIAN_POINT('Ctrl Pts',(-33.844379571971,68.8330790123165,84.4406148964829));
#214835=CARTESIAN_POINT('Ctrl Pts',(-33.8166575402668,67.7495989575,83.8116515107386));
#214836=CARTESIAN_POINT('Ctrl Pts',(-33.7978618271786,67.0680368267213,
83.3225450944089));
#214837=CARTESIAN_POINT('Ctrl Pts',(-33.7597997553321,65.7806670303727,
82.1958171576032));
#214838=CARTESIAN_POINT('Ctrl Pts',(-33.7407550949359,65.1827979707771,
81.555462203927));
#214839=CARTESIAN_POINT('Ctrl Pts',(-33.7021414094037,64.1328765984622,
80.175375567761));
#214840=CARTESIAN_POINT('Ctrl Pts',(-33.682839143146,63.6812806004565,79.4407540146172));
#214841=CARTESIAN_POINT('Ctrl Pts',(-33.6546292299432,63.1225457536784,
78.2899893501863));
#214842=CARTESIAN_POINT('Ctrl Pts',(-33.6454078184583,62.9578599763085,
77.9044202230711));
#214843=CARTESIAN_POINT('Ctrl Pts',(-33.6170767572343,62.5130524810403,
76.7057344151352));
#214844=CARTESIAN_POINT('Ctrl Pts',(-33.5977256972488,62.2946797467361,
75.8722255205868));
#214845=CARTESIAN_POINT('Ctrl Pts',(-33.5580794599566,62.0147439387142,
74.1054476306213));
#214846=CARTESIAN_POINT('Ctrl Pts',(-33.5377636242054,61.9681514221822,
73.1746553003406));
#214847=CARTESIAN_POINT('Ctrl Pts',(-33.508484753883,62.0429790849531,71.8658179188578));
#214848=CARTESIAN_POINT('Ctrl Pts',(-33.4999291116805,62.0815359334979,
71.485903537963));
#214849=CARTESIAN_POINT('Ctrl Pts',(-33.4761071074569,62.2359829592044,
70.4295195145831));
#214850=CARTESIAN_POINT('Ctrl Pts',(-33.4611010983193,62.3887756438287,
69.7597214309783));
#214851=CARTESIAN_POINT('Ctrl Pts',(-33.4236530676507,62.8946047984785,
68.1439051395504));
#214852=CARTESIAN_POINT('Ctrl Pts',(-33.4009695995417,63.3061994461789,
67.2209180035347));
#214853=CARTESIAN_POINT('Ctrl Pts',(-33.3675458891444,64.0778580688789,
65.9205273594993));
#214854=CARTESIAN_POINT('Ctrl Pts',(-33.3564646251883,64.3605967533275,
65.5016986277275));
#214855=CARTESIAN_POINT('Ctrl Pts',(-33.3339968452133,64.9764058514039,
64.6950610429881));
#214856=CARTESIAN_POINT('Ctrl Pts',(-33.3226268060556,65.3094146853376,
64.3083029275426));
#214857=CARTESIAN_POINT('Ctrl Pts',(-33.3112169404745,65.6642757110361,
63.9421080804774));
#214858=CARTESIAN_POINT('Origin',(-21.6548258024609,75.,72.9888893865801));
#214859=CARTESIAN_POINT('',(-36.4473639743914,87.0149197055719,77.9529305295058));
#214860=CARTESIAN_POINT('',(-36.1412950695185,87.0149197055719,77.9529305295058));
#214861=CARTESIAN_POINT('',(-21.6548258024609,87.0149197055719,77.9529305295058));
#214862=CARTESIAN_POINT('Ctrl Pts',(-34.6333744106366,87.0149197055719,
77.9529305295058));
#214863=CARTESIAN_POINT('Ctrl Pts',(-34.6410144983003,87.1472724658191,
77.6325851211187));
#214864=CARTESIAN_POINT('Ctrl Pts',(-34.6486583935817,87.2668387887337,
77.3068853606196));
#214865=CARTESIAN_POINT('Ctrl Pts',(-34.6738484033645,87.6155424360587,
76.2249071553366));
#214866=CARTESIAN_POINT('Ctrl Pts',(-34.6915963640561,87.7887956245091,
75.4527109380275));
#214867=CARTESIAN_POINT('Ctrl Pts',(-34.7263102933153,87.990609401202,73.9048043249291));
#214868=CARTESIAN_POINT('Ctrl Pts',(-34.7431409118189,88.0220646059666,
73.1326648094785));
#214869=CARTESIAN_POINT('Ctrl Pts',(-34.7762781355641,87.9501651988379,
71.6426752970501));
#214870=CARTESIAN_POINT('Ctrl Pts',(-34.7924822107326,87.855676750075,70.9271815437092));
#214871=CARTESIAN_POINT('Ctrl Pts',(-34.8245199274,87.5488040528677,69.5177537052255));
#214872=CARTESIAN_POINT('Ctrl Pts',(-34.8402934076479,87.3367026937042,
68.8263132726193));
#214873=CARTESIAN_POINT('Ctrl Pts',(-34.8734422301321,86.7815923625556,
67.4401181718058));
#214874=CARTESIAN_POINT('Ctrl Pts',(-34.8907994054764,86.4317462687593,
66.7511050424085));
#214875=CARTESIAN_POINT('Ctrl Pts',(-34.9254355268943,85.6039486300616,
65.4270899110364));
#214876=CARTESIAN_POINT('Ctrl Pts',(-34.9427031652308,85.1247666244966,
64.7965975177365));
#214877=CARTESIAN_POINT('Ctrl Pts',(-34.9794395177859,84.010501831775,63.5787263235851));
#214878=CARTESIAN_POINT('Ctrl Pts',(-34.9987656114896,83.3681062130668,
63.0031434726594));
#214879=CARTESIAN_POINT('Ctrl Pts',(-35.0269611300624,82.3363247293893,
62.2486428640155));
#214880=CARTESIAN_POINT('Ctrl Pts',(-35.0361517023222,81.9873840917416,
62.0184281753119));
#214881=CARTESIAN_POINT('Ctrl Pts',(-35.0644318262463,80.8888088134717,
61.3673496404138));
#214882=CARTESIAN_POINT('Ctrl Pts',(-35.0837646192032,80.1080443615473,
61.0036431587081));
#214883=CARTESIAN_POINT('Ctrl Pts',(-35.1199264595917,78.5698626863148,
60.4649172597747));
#214884=CARTESIAN_POINT('Ctrl Pts',(-35.1367626891527,77.8213855619841,
60.2753694849194));
#214885=CARTESIAN_POINT('Ctrl Pts',(-35.1730376670567,76.2109465644052,
60.0168418104364));
#214886=CARTESIAN_POINT('Ctrl Pts',(-35.1923839804659,75.3499051511802,
59.9651423693992));
#214887=CARTESIAN_POINT('Ctrl Pts',(-35.2205570259837,74.074235674986,60.0152174964822));
#214888=CARTESIAN_POINT('Ctrl Pts',(-35.2297080310198,73.6594045914688,
60.0515014820007));
#214889=CARTESIAN_POINT('Ctrl Pts',(-35.2574286343145,72.4182548404463,
60.2204054804586));
#214890=CARTESIAN_POINT('Ctrl Pts',(-35.2762157315111,71.6023019547656,
60.4129114049523));
#214891=CARTESIAN_POINT('Ctrl Pts',(-35.313792459455,70.0030946179789,60.9573297756987));
#214892=CARTESIAN_POINT('Ctrl Pts',(-35.3323865847917,69.2246777222068,
61.3109979269255));
#214893=CARTESIAN_POINT('Ctrl Pts',(-35.3705224383085,67.7419341476506,
62.1694287967758));
#214894=CARTESIAN_POINT('Ctrl Pts',(-35.3898426629352,67.0419700700413,
62.6733662263117));
#214895=CARTESIAN_POINT('Ctrl Pts',(-35.4180426922991,66.0834484591887,
63.5194670460732));
#214896=CARTESIAN_POINT('Ctrl Pts',(-35.4272420435321,65.7834928920688,
63.8111528869795));
#214897=CARTESIAN_POINT('Ctrl Pts',(-35.4555365738423,64.9116654239943,
64.7448662934268));
#214898=CARTESIAN_POINT('Ctrl Pts',(-35.4748750176126,64.3889339507664,
65.4295455466578));
#214899=CARTESIAN_POINT('Ctrl Pts',(-35.5114915870395,63.521864149559,66.8343076002342));
#214900=CARTESIAN_POINT('Ctrl Pts',(-35.5287861377058,63.1685136464488,
67.544404319794));
#214901=CARTESIAN_POINT('Ctrl Pts',(-35.5655511234903,62.5704350035212,
69.0842496789816));
#214902=CARTESIAN_POINT('Ctrl Pts',(-35.5848757371742,62.3393145831473,
69.915234724591));
#214903=CARTESIAN_POINT('Ctrl Pts',(-35.6130724628373,62.1204346444043,
71.174659599355));
#214904=CARTESIAN_POINT('Ctrl Pts',(-35.622265337517,62.0687744297023,71.5895901190422));
#214905=CARTESIAN_POINT('Ctrl Pts',(-35.6505492332774,61.9722424867744,
72.8630698276623));
#214906=CARTESIAN_POINT('Ctrl Pts',(-35.6698835404298,61.9924009342307,
73.7241800810811));
#214907=CARTESIAN_POINT('Ctrl Pts',(-35.7061605490294,62.1921485258402,
75.3470532185749));
#214908=CARTESIAN_POINT('Ctrl Pts',(-35.7231128405259,62.3556818101983,
76.1070973531199));
#214909=CARTESIAN_POINT('Ctrl Pts',(-35.7595123308866,62.8414434762071,
77.6696915924371));
#214910=CARTESIAN_POINT('Ctrl Pts',(-35.7788538220983,63.1778294579789,
78.4639875642219));
#214911=CARTESIAN_POINT('Ctrl Pts',(-35.8070334432503,63.7898918328367,
79.5848776875493));
#214912=CARTESIAN_POINT('Ctrl Pts',(-35.8161955881248,64.0070310580069,
79.9407395369645));
#214913=CARTESIAN_POINT('Ctrl Pts',(-35.8439134553117,64.709891921015,80.9771250993757));
#214914=CARTESIAN_POINT('Ctrl Pts',(-35.8626874295874,65.2444848391333,
81.6218577646133));
#214915=CARTESIAN_POINT('Ctrl Pts',(-35.8995680876586,66.4210303757784,
82.7908559751471));
#214916=CARTESIAN_POINT('Ctrl Pts',(-35.9175169075991,67.0585854030976,
83.3141598198811));
#214917=CARTESIAN_POINT('Ctrl Pts',(-35.9549652982439,68.4551599768391,
84.2541222654419));
#214918=CARTESIAN_POINT('Ctrl Pts',(-35.9743055043938,69.2149449454332,
84.6625156941114));
#214919=CARTESIAN_POINT('Ctrl Pts',(-36.0024867255381,70.3943086154943,
85.152823300772));
#214920=CARTESIAN_POINT('Ctrl Pts',(-36.0116516207469,70.7865987406913,
85.2942106379164));
#214921=CARTESIAN_POINT('Ctrl Pts',(-36.0393686835006,71.9836159836327,
85.6616679382997));
#214922=CARTESIAN_POINT('Ctrl Pts',(-36.0581392723562,72.8039998782774,
85.8292732298157));
#214923=CARTESIAN_POINT('Ctrl Pts',(-36.0948471064515,74.4457882050427,
86.0026489020353));
#214924=CARTESIAN_POINT('Ctrl Pts',(-36.1126358225816,75.2630700598925,
86.0117879939816));
#214925=CARTESIAN_POINT('Ctrl Pts',(-36.1499133284127,76.9333250757294,
85.8730915011334));
#214926=CARTESIAN_POINT('Ctrl Pts',(-36.169257629372,77.7816622711618,85.7169204670744));
#214927=CARTESIAN_POINT('Ctrl Pts',(-36.1974335359189,79.0083435510802,
85.3625125683815));
#214928=CARTESIAN_POINT('Ctrl Pts',(-36.2065893584936,79.4025750479469,
85.2277905438018));
#214929=CARTESIAN_POINT('Ctrl Pts',(-36.2343088797544,80.5669144822184,
84.7663455979332));
#214930=CARTESIAN_POINT('Ctrl Pts',(-36.2530904160522,81.3126370513456,
84.384046693144));
#214931=CARTESIAN_POINT('Ctrl Pts',(-36.2903666117951,82.7235994368813,
83.4794370187516));
#214932=CARTESIAN_POINT('Ctrl Pts',(-36.3086820169662,83.3851307160123,
82.9586018770635));
#214933=CARTESIAN_POINT('Ctrl Pts',(-36.3465212556786,84.6131905871474,
81.7824614731507));
#214934=CARTESIAN_POINT('Ctrl Pts',(-36.3658508378358,85.1739860388722,
81.1270932549301));
#214935=CARTESIAN_POINT('Ctrl Pts',(-36.3940433126084,85.9046378054383,
80.0785465049186));
#214936=CARTESIAN_POINT('Ctrl Pts',(-36.4032281993759,86.1267213877352,
79.7246472984632));
#214937=CARTESIAN_POINT('Ctrl Pts',(-36.4240420244147,86.5874331272118,
78.9053318148693));
#214938=CARTESIAN_POINT('Ctrl Pts',(-36.4356882939277,86.8156600708001,
78.4352167240423));
#214939=CARTESIAN_POINT('Ctrl Pts',(-36.4473639743914,87.0149197055719,
77.9529305295058));
#214940=CARTESIAN_POINT('Ctrl Pts',(-36.1412950695185,87.0149197055719,
77.9529305295058));
#214941=CARTESIAN_POINT('Ctrl Pts',(-36.1298525502738,86.8196408780571,
78.4255816146268));
#214942=CARTESIAN_POINT('Ctrl Pts',(-36.1184583697883,86.596525045201,78.8865806401068));
#214943=CARTESIAN_POINT('Ctrl Pts',(-36.0979502789332,86.1427955726876,
79.6980294853537));
#214944=CARTESIAN_POINT('Ctrl Pts',(-36.0887627234461,85.9214998403717,
80.0525495586229));
#214945=CARTESIAN_POINT('Ctrl Pts',(-36.0604875345434,85.1939912928237,
81.1018877762301));
#214946=CARTESIAN_POINT('Ctrl Pts',(-36.0411567591015,84.6356671185127,
81.7577039567634));
#214947=CARTESIAN_POINT('Ctrl Pts',(-36.005141592816,83.4665101443726,82.8834150940506));
#214948=CARTESIAN_POINT('Ctrl Pts',(-35.98845316749,82.8706522301808,83.3636796878424));
#214949=CARTESIAN_POINT('Ctrl Pts',(-35.9542340749897,81.5921201549929,
84.2203098349429));
#214950=CARTESIAN_POINT('Ctrl Pts',(-35.9367849374459,80.910852539125,84.593314433653));
#214951=CARTESIAN_POINT('Ctrl Pts',(-35.9065947946083,79.6601739007216,
85.1392086270328));
#214952=CARTESIAN_POINT('Ctrl Pts',(-35.8936717608624,79.1045078316714,
85.3379984858156));
#214953=CARTESIAN_POINT('Ctrl Pts',(-35.8631504302149,77.7800427230511,
85.7125134755317));
#214954=CARTESIAN_POINT('Ctrl Pts',(-35.845451574069,77.004936163505,85.857435042336));
#214955=CARTESIAN_POINT('Ctrl Pts',(-35.8119077179347,75.5013839149763,
85.9993391579588));
#214956=CARTESIAN_POINT('Ctrl Pts',(-35.7961055627523,74.7768473497895,
86.0070843132759));
#214957=CARTESIAN_POINT('Ctrl Pts',(-35.7629303782296,73.2864365511284,
85.898505926007));
#214958=CARTESIAN_POINT('Ctrl Pts',(-35.7455770786224,72.5239468151579,
85.7741799727015));
#214959=CARTESIAN_POINT('Ctrl Pts',(-35.7108868074003,71.0087798231814,
85.3864273950003));
#214960=CARTESIAN_POINT('Ctrl Pts',(-35.6935603236903,70.2601713027601,
85.1199577033177));
#214961=CARTESIAN_POINT('Ctrl Pts',(-35.6567613902556,68.7596768214792,
84.4256128919062));
#214962=CARTESIAN_POINT('Ctrl Pts',(-35.6374385692242,68.0166264949497,
83.9876521989185));
#214963=CARTESIAN_POINT('Ctrl Pts',(-35.6092404454297,66.9849945013812,
83.2326392530982));
#214964=CARTESIAN_POINT('Ctrl Pts',(-35.6000448638896,66.6597835518844,
82.9696465609767));
#214965=CARTESIAN_POINT('Ctrl Pts',(-35.5717565278372,65.706492535983,82.1195554927621));
#214966=CARTESIAN_POINT('Ctrl Pts',(-35.5524204694709,65.123457971628,81.4854917713839));
#214967=CARTESIAN_POINT('Ctrl Pts',(-35.5160044050387,64.1373087680155,
80.1731712204565));
#214968=CARTESIAN_POINT('Ctrl Pts',(-35.4989119659459,63.7247642495407,
79.506636882953));
#214969=CARTESIAN_POINT('Ctrl Pts',(-35.4623624821328,62.9895514411598,
78.0376027251217));
#214970=CARTESIAN_POINT('Ctrl Pts',(-35.443027406734,62.6817967463728,77.2317964309454));
#214971=CARTESIAN_POINT('Ctrl Pts',(-35.4148403435027,62.3464065441204,
75.9989730879931));
#214972=CARTESIAN_POINT('Ctrl Pts',(-35.4056652342491,62.2563351350567,
75.5913952682117));
#214973=CARTESIAN_POINT('Ctrl Pts',(-35.3779516248455,62.0453332897541,
74.3575303193435));
#214974=CARTESIAN_POINT('Ctrl Pts',(-35.3591941342385,61.9842008020369,
73.5232338078267));
#214975=CARTESIAN_POINT('Ctrl Pts',(-35.3231332769107,62.0216426046779,
71.9013533735228));
#214976=CARTESIAN_POINT('Ctrl Pts',(-35.3059436051296,62.1113612201544,
71.1171275422089));
#214977=CARTESIAN_POINT('Ctrl Pts',(-35.2712619618553,62.4285603751698,
69.5895374388546));
#214978=CARTESIAN_POINT('Ctrl Pts',(-35.2538720381301,62.6527066399022,
68.8487156849491));
#214979=CARTESIAN_POINT('Ctrl Pts',(-35.2245121001951,63.148280938239,67.6182535143398));
#214980=CARTESIAN_POINT('Ctrl Pts',(-35.212363927004,63.3879146739514,67.1180759417574));
#214981=CARTESIAN_POINT('Ctrl Pts',(-35.1810619263656,64.0787253779095,
65.8850795563455));
#214982=CARTESIAN_POINT('Ctrl Pts',(-35.1617255453019,64.5720124689809,
65.1789329448341));
#214983=CARTESIAN_POINT('Ctrl Pts',(-35.1252831314442,65.641357267583,63.9318661176365));
#214984=CARTESIAN_POINT('Ctrl Pts',(-35.1081641341423,66.2040941070758,
63.384415887291));
#214985=CARTESIAN_POINT('Ctrl Pts',(-35.0715862747248,67.4810526523204,
62.3490677629285));
#214986=CARTESIAN_POINT('Ctrl Pts',(-35.0522524904512,68.2015736270285,
61.874853984205));
#214987=CARTESIAN_POINT('Ctrl Pts',(-35.0240640822832,69.3332023665428,
61.2815618711429));
#214988=CARTESIAN_POINT('Ctrl Pts',(-35.0148865760114,69.7118740965361,
61.1057148441394));
#214989=CARTESIAN_POINT('Ctrl Pts',(-34.9871738864033,70.871174050503,60.6337671809289));
#214990=CARTESIAN_POINT('Ctrl Pts',(-34.9684195930582,71.6724955656291,
60.3942894384212));
#214991=CARTESIAN_POINT('Ctrl Pts',(-34.9325116520515,73.2576783180675,
60.0825148469752));
#214992=CARTESIAN_POINT('Ctrl Pts',(-34.9154634923922,74.0361699556754,
60.0011556725565));
#214993=CARTESIAN_POINT('Ctrl Pts',(-34.8809570298485,75.5885194412834,
59.979330204309));
#214994=CARTESIAN_POINT('Ctrl Pts',(-34.8635915756472,76.3592323104988,
60.0371529876881));
#214995=CARTESIAN_POINT('Ctrl Pts',(-34.8346151917973,77.6505818690484,
60.2506263943429));
#214996=CARTESIAN_POINT('Ctrl Pts',(-34.8228282368789,78.1749578050771,
60.3711014270372));
#214997=CARTESIAN_POINT('Ctrl Pts',(-34.7924368846693,79.491455892608,60.760855423949));
#214998=CARTESIAN_POINT('Ctrl Pts',(-34.7736652954155,80.2678135037159,
61.0746912797687));
#214999=CARTESIAN_POINT('Ctrl Pts',(-34.7369066461279,81.7337947492177,
61.8387922762775));
#215000=CARTESIAN_POINT('Ctrl Pts',(-34.7190708588111,82.4216467956235,
62.2843192095421));
#215001=CARTESIAN_POINT('Ctrl Pts',(-34.6817431027039,83.7380427758999,
63.3251935441175));
#215002=CARTESIAN_POINT('Ctrl Pts',(-34.6623999726677,84.35835774346,63.9245880071219));
#215003=CARTESIAN_POINT('Ctrl Pts',(-34.6342224804547,85.1842612527145,
64.8985071785536));
#215004=CARTESIAN_POINT('Ctrl Pts',(-34.6250639691175,85.4382125726879,
65.2289164659393));
#215005=CARTESIAN_POINT('Ctrl Pts',(-34.5973451184325,86.1528232112991,
66.2573800370101));
#215006=CARTESIAN_POINT('Ctrl Pts',(-34.5785667610308,86.5624635873858,
66.9882140541144));
#215007=CARTESIAN_POINT('Ctrl Pts',(-34.541458538371,87.2344805718937,68.5155273723569));
#215008=CARTESIAN_POINT('Ctrl Pts',(-34.5232988409555,87.4958477473876,
69.308226663165));
#215009=CARTESIAN_POINT('Ctrl Pts',(-34.4856255323828,87.869451885214,70.9597061078104));
#215010=CARTESIAN_POINT('Ctrl Pts',(-34.4662912175051,87.9755189309129,
71.8157330745989));
#215011=CARTESIAN_POINT('Ctrl Pts',(-34.4381033563664,88.0062765790443,
73.0930489463427));
#215012=CARTESIAN_POINT('Ctrl Pts',(-34.4289268273952,87.9962343871544,
73.5103979950093));
#215013=CARTESIAN_POINT('Ctrl Pts',(-34.4012137576439,87.9059515380183,
74.7588594088365));
#215014=CARTESIAN_POINT('Ctrl Pts',(-34.3824581549403,87.7657603498323,
75.5834465426814));
#215015=CARTESIAN_POINT('Ctrl Pts',(-34.3516509315271,87.4032629321684,
76.9212247748124));
#215016=CARTESIAN_POINT('Ctrl Pts',(-34.3395731065913,87.2253450875266,
77.4436188627799));
#215017=CARTESIAN_POINT('Ctrl Pts',(-34.3273949797549,87.0149197055719,
77.9529305295058));
#215018=CARTESIAN_POINT('Origin',(-21.6548258024609,75.,72.9888893865801));
#215019=CARTESIAN_POINT('',(-39.5675364832709,87.0149197055719,77.9529305295058));
#215020=CARTESIAN_POINT('',(-39.5675364832709,79.9640411429257,60.9739696810082));
#215021=CARTESIAN_POINT('Origin',(-39.5675364832709,75.,72.9888893865801));
#215022=CARTESIAN_POINT('Origin',(-39.5675364832709,75.,72.9888893865801));
#215023=CARTESIAN_POINT('',(-39.3655152556871,87.0149196672213,77.9529306223295));
#215024=CARTESIAN_POINT('',(-21.6548258024609,87.0149197055719,77.9529305295058));
#215025=CARTESIAN_POINT('',(-39.378281183842,87.9789324623827,72.2490839199061));
#215026=CARTESIAN_POINT('Ctrl Pts',(-39.3655152559408,87.014919667221,77.9529306223301));
#215027=CARTESIAN_POINT('Ctrl Pts',(-39.367974326097,87.3865627273345,77.0534091840337));
#215028=CARTESIAN_POINT('Ctrl Pts',(-39.3710406973607,87.6560163266104,
76.1149984769994));
#215029=CARTESIAN_POINT('Ctrl Pts',(-39.3753005433957,87.9804112067045,
74.1956296276193));
#215030=CARTESIAN_POINT('Ctrl Pts',(-39.376513824047,88.0343195956285,73.2207797100457));
#215031=CARTESIAN_POINT('Ctrl Pts',(-39.3782811843755,87.9789324627048,
72.2490839198887));
#215032=CARTESIAN_POINT('',(-38.9114901702032,87.9789324623618,72.2490839198538));
#215033=CARTESIAN_POINT('',(-38.9115960243709,87.9789324627076,72.2490839198856));
#215034=CARTESIAN_POINT('',(-38.6651607695591,87.0149202732382,77.9529291555314));
#215035=CARTESIAN_POINT('Ctrl Pts',(-38.9114901696398,87.9789324627004,
72.2490839198105));
#215036=CARTESIAN_POINT('Ctrl Pts',(-38.87002296087,88.0343175630345,73.2207440507034));
#215037=CARTESIAN_POINT('Ctrl Pts',(-38.8281416219942,87.9804138359084,
74.1955869480231));
#215038=CARTESIAN_POINT('Ctrl Pts',(-38.7459661857041,87.6560286922808,
76.1149524347907));
#215039=CARTESIAN_POINT('Ctrl Pts',(-38.7059499709518,87.3865732800262,
77.0533833312218));
#215040=CARTESIAN_POINT('Ctrl Pts',(-38.6651607695591,87.0149202732382,
77.9529291555314));
#215041=CARTESIAN_POINT('',(-37.9553013386749,87.0149197239183,77.9529304851004));
#215042=CARTESIAN_POINT('',(-21.6548258024609,87.0149197055719,77.9529305295058));
#215043=CARTESIAN_POINT('',(-39.3215010433097,70.2740072122874,85.0994220373138));
#215044=CARTESIAN_POINT('Ctrl Pts',(-39.321506023786,70.2738583024975,85.099363557938));
#215045=CARTESIAN_POINT('Ctrl Pts',(-39.3114020880209,69.8468174583147,
84.9327098405302));
#215046=CARTESIAN_POINT('Ctrl Pts',(-39.3012855729604,69.4288913059223,
84.7435856333423));
#215047=CARTESIAN_POINT('Ctrl Pts',(-39.280963349317,68.6176528904388,84.3234743085914));
#215048=CARTESIAN_POINT('Ctrl Pts',(-39.2707729228055,68.2247471115269,
84.0930830360041));
#215049=CARTESIAN_POINT('Ctrl Pts',(-39.2407041203334,67.1021730628955,
83.3530282551602));
#215050=CARTESIAN_POINT('Ctrl Pts',(-39.2212815979088,66.4118048498001,
82.7885807671965));
#215051=CARTESIAN_POINT('Ctrl Pts',(-39.1884559885027,65.3675884171679,
81.7390900665183));
#215052=CARTESIAN_POINT('Ctrl Pts',(-39.1752312649901,64.9797544211849,
81.2921440976121));
#215053=CARTESIAN_POINT('Ctrl Pts',(-39.1427805644905,64.1053250437752,
80.1335688480066));
#215054=CARTESIAN_POINT('Ctrl Pts',(-39.1239870143577,63.6564342372199,
79.3970017841523));
#215055=CARTESIAN_POINT('Ctrl Pts',(-39.0864295461419,62.9222219147695,
77.8697693025234));
#215056=CARTESIAN_POINT('Ctrl Pts',(-39.0676566045221,62.63401471161,77.0849988222401));
#215057=CARTESIAN_POINT('Ctrl Pts',(-39.030614924758,62.2114826142195,75.4693290884284));
#215058=CARTESIAN_POINT('Ctrl Pts',(-39.012353616074,62.0784797054115,74.6420922817204));
#215059=CARTESIAN_POINT('Ctrl Pts',(-38.9844493981105,61.9995852932347,
73.3921966966507));
#215060=CARTESIAN_POINT('Ctrl Pts',(-38.9751206225394,61.9933378521099,
72.9755430471695));
#215061=CARTESIAN_POINT('Ctrl Pts',(-38.946578292483,62.0355334386009,71.6993073294617));
#215062=CARTESIAN_POINT('Ctrl Pts',(-38.9277937808025,62.1492825577064,
70.8442501044364));
#215063=CARTESIAN_POINT('Ctrl Pts',(-38.8915606746817,62.5241755004248,
69.2535805458345));
#215064=CARTESIAN_POINT('Ctrl Pts',(-38.8741679040607,62.7685641781066,
68.5177937551494));
#215065=CARTESIAN_POINT('Ctrl Pts',(-38.8378616598784,63.4193471623844,
67.0200742385238));
#215066=CARTESIAN_POINT('Ctrl Pts',(-38.8191262125368,63.8390537658709,
66.2679101802637));
#215067=CARTESIAN_POINT('Ctrl Pts',(-38.790688162261,64.568589507438,65.2197014772622));
#215068=CARTESIAN_POINT('Ctrl Pts',(-38.7813317124692,64.823687144539,64.888441178162));
#215069=CARTESIAN_POINT('Ctrl Pts',(-38.7527494948693,65.6514972276645,
63.9144306783834));
#215070=CARTESIAN_POINT('Ctrl Pts',(-38.7339489678599,66.272414068001,63.3157538675906));
#215071=CARTESIAN_POINT('Ctrl Pts',(-38.6961323116346,67.6122913153949,
62.258655584523));
#215072=CARTESIAN_POINT('Ctrl Pts',(-38.6770852008029,68.32626924716,61.8006157399202));
#215073=CARTESIAN_POINT('Ctrl Pts',(-38.649063492353,69.4511464508941,61.2252027944466));
#215074=CARTESIAN_POINT('Ctrl Pts',(-38.6398975354063,69.8315507630826,
61.0531769281282));
#215075=CARTESIAN_POINT('Ctrl Pts',(-38.609331741426,71.1197986245397,60.5437628631491));
#215076=CARTESIAN_POINT('Ctrl Pts',(-38.5876505567486,72.0569819038552,
60.2894501687834));
#215077=CARTESIAN_POINT('Ctrl Pts',(-38.5489686896933,73.7739355034221,
60.023990570254));
#215078=CARTESIAN_POINT('Ctrl Pts',(-38.5321845447893,74.5431454813509,
59.9741622638402));
#215079=CARTESIAN_POINT('Ctrl Pts',(-38.5008117355056,75.9561224552041,
60.0081089072099));
#215080=CARTESIAN_POINT('Ctrl Pts',(-38.4863650581999,76.5979715007598,
60.0714084547044));
#215081=CARTESIAN_POINT('Ctrl Pts',(-38.4626017641503,77.6473753072034,
60.2543388149753));
#215082=CARTESIAN_POINT('Ctrl Pts',(-38.4533157484133,78.0585156925993,
60.3467828974843));
#215083=CARTESIAN_POINT('Ctrl Pts',(-38.4164245293697,79.6716516533196,
60.7928065998949));
#215084=CARTESIAN_POINT('Ctrl Pts',(-38.3883367518857,80.8243084251877,
61.2993133040721));
#215085=CARTESIAN_POINT('Ctrl Pts',(-38.3514289180863,82.2397648680118,
62.1833742844974));
#215086=CARTESIAN_POINT('Ctrl Pts',(-38.3422820314882,82.5821013107596,
62.4207726013387));
#215087=CARTESIAN_POINT('Ctrl Pts',(-38.3129369998464,83.636119886382,63.2293150724732));
#215088=CARTESIAN_POINT('Ctrl Pts',(-38.2924757734087,84.2993534094154,
63.8590557240803));
#215089=CARTESIAN_POINT('Ctrl Pts',(-38.2530563239258,85.4489216617826,
65.2069402920131));
#215090=CARTESIAN_POINT('Ctrl Pts',(-38.2343240422644,85.9404230632382,
65.9145806437461));
#215091=CARTESIAN_POINT('Ctrl Pts',(-38.2058724294769,86.5621961834555,
67.0314554614813));
#215092=CARTESIAN_POINT('Ctrl Pts',(-38.1964978479394,86.7481070142651,
67.4070097828176));
#215093=CARTESIAN_POINT('Ctrl Pts',(-38.1678916339641,87.2595380844619,
68.5793797065549));
#215094=CARTESIAN_POINT('Ctrl Pts',(-38.1490793502634,87.5243955576249,
69.4000778515985));
#215095=CARTESIAN_POINT('Ctrl Pts',(-38.1107919550294,87.8898085558847,
71.0896871066573));
#215096=CARTESIAN_POINT('Ctrl Pts',(-38.0912453846014,87.987865078529,71.9547294911018));
#215097=CARTESIAN_POINT('Ctrl Pts',(-38.0534359995219,88.0096166010421,
73.6598078459812));
#215098=CARTESIAN_POINT('Ctrl Pts',(-38.03514977022,87.9394741214373,74.4956319081321));
#215099=CARTESIAN_POINT('Ctrl Pts',(-38.0072316254609,87.7149408798079,
75.72810147097));
#215100=CARTESIAN_POINT('Ctrl Pts',(-37.9979133811153,87.6207958687613,
76.1334903360733));
#215101=CARTESIAN_POINT('Ctrl Pts',(-37.9774099080487,87.3706399895231,
77.0161397197716));
#215102=CARTESIAN_POINT('Ctrl Pts',(-37.966341833165,87.2061795722548,77.4900068955137));
#215103=CARTESIAN_POINT('Ctrl Pts',(-37.9553013376164,87.0149197239272,
77.9529304850788));
#215104=CARTESIAN_POINT('Ctrl Pts',(-39.3215011869246,70.2741248823959,
85.0994675880043));
#215105=CARTESIAN_POINT('Ctrl Pts',(-39.3236712637677,71.0632752616707,
85.4074154067983));
#215106=CARTESIAN_POINT('Ctrl Pts',(-39.3262569458996,71.880640057225,85.6374944349641));
#215107=CARTESIAN_POINT('Ctrl Pts',(-39.3301175566085,73.5347367964358,
85.9328892466978));
#215108=CARTESIAN_POINT('Ctrl Pts',(-39.3314200360407,74.3670796427984,
86.0001740554811));
#215109=CARTESIAN_POINT('Ctrl Pts',(-39.3355204404005,76.8868812019081,
85.9613804639162));
#215110=CARTESIAN_POINT('Ctrl Pts',(-39.3415199539802,78.5525524484387,
85.6073365102985));
#215111=CARTESIAN_POINT('Ctrl Pts',(-39.3463525919956,80.8711551225581,
84.617527519692));
#215112=CARTESIAN_POINT('Ctrl Pts',(-39.3473555822715,81.6049539354431,
84.2169902570333));
#215113=CARTESIAN_POINT('Ctrl Pts',(-39.3513429793926,83.3501269679487,
83.0337632759548));
#215114=CARTESIAN_POINT('Ctrl Pts',(-39.3558794304814,84.2940584038291,
82.1673740340381));
#215115=CARTESIAN_POINT('Ctrl Pts',(-39.3612997924158,85.8887379039215,
80.2011041664733));
#215116=CARTESIAN_POINT('Ctrl Pts',(-39.3623386985112,86.5348437171632,
79.1149045610223));
#215117=CARTESIAN_POINT('Ctrl Pts',(-39.3655152812068,87.0149234856985,
77.9529213801122));
#215118=CARTESIAN_POINT('Origin',(-23.4378585958609,75.,72.9888893865801));
#215119=CARTESIAN_POINT('',(-23.3083467243891,86.7753674719618,77.8539778944305));
#215120=CARTESIAN_POINT('',(-23.4378585958609,86.8950725984871,77.9034149284857));
#215121=CARTESIAN_POINT('',(-23.5671968062386,81.7816282713719,84.0797707272729));
#215122=CARTESIAN_POINT('Ctrl Pts',(-23.5672140314447,81.7816648771554,
84.07983260589));
#215123=CARTESIAN_POINT('Ctrl Pts',(-23.5673199177301,81.7897993012429,
84.0748587333312));
#215124=CARTESIAN_POINT('Ctrl Pts',(-23.5674258040155,81.7979282533515,
84.0698759117298));
#215125=CARTESIAN_POINT('Ctrl Pts',(-23.5675316903009,81.8060517138039,
84.0648841531474));
#215126=CARTESIAN_POINT('',(-22.5675364824894,86.9998979375059,73.039443228467));
#215127=CARTESIAN_POINT('Ctrl Pts',(-23.5671139309304,81.7814521506577,
84.0794730118532));
#215128=CARTESIAN_POINT('Ctrl Pts',(-23.5554441969661,81.093704963152,84.4863247226582));
#215129=CARTESIAN_POINT('Ctrl Pts',(-23.5440549453205,80.3694906051007,
84.8293747514794));
#215130=CARTESIAN_POINT('Ctrl Pts',(-23.5205294743054,78.8459785012502,
85.3850651834404));
#215131=CARTESIAN_POINT('Ctrl Pts',(-23.5081796031132,78.0485116703269,
85.5920974487081));
#215132=CARTESIAN_POINT('Ctrl Pts',(-23.4721296505078,75.648480810247,85.9772996965804));
#215133=CARTESIAN_POINT('Ctrl Pts',(-23.4493257715469,74.0212183490508,
85.9346245406178));
#215134=CARTESIAN_POINT('Ctrl Pts',(-23.400751606844,70.8562592203477,85.2427926589502));
#215135=CARTESIAN_POINT('Ctrl Pts',(-23.3776454762802,69.3427417189109,
84.5970625631213));
#215136=CARTESIAN_POINT('Ctrl Pts',(-23.3403526762987,67.289062705934,83.2069683034419));
#215137=CARTESIAN_POINT('Ctrl Pts',(-23.3274897439033,66.633733857187,82.6607486085187));
#215138=CARTESIAN_POINT('Ctrl Pts',(-23.3030014708832,65.4741786697172,
81.4799624604395));
#215139=CARTESIAN_POINT('Ctrl Pts',(-23.2913605641576,64.9652158093804,
80.8531966773066));
#215140=CARTESIAN_POINT('Ctrl Pts',(-23.273148804062,64.2923408780737,79.8406857186491));
#215141=CARTESIAN_POINT('Ctrl Pts',(-23.266907699706,64.0819260352267,79.4879801447772));
#215142=CARTESIAN_POINT('Ctrl Pts',(-23.2363418036894,63.135444316788,77.7111294603452));
#215143=CARTESIAN_POINT('Ctrl Pts',(-23.2132436084909,62.6532773507385,
76.1605022589756));
#215144=CARTESIAN_POINT('Ctrl Pts',(-23.1759412452441,62.3852856750543,
73.7273574819093));
#215145=CARTESIAN_POINT('Ctrl Pts',(-23.1630923328798,62.376935370315,72.8851889496607));
#215146=CARTESIAN_POINT('Ctrl Pts',(-23.1386272326454,62.5232656519847,
71.2588084415987));
#215147=CARTESIAN_POINT('Ctrl Pts',(-23.1269905153999,62.6689014872749,
70.4759290443836));
#215148=CARTESIAN_POINT('Ctrl Pts',(-23.1023462125105,63.1162283208151,
68.9167373502686));
#215149=CARTESIAN_POINT('Ctrl Pts',(-23.0894884991716,63.4231978635774,
68.1451374417189));
#215150=CARTESIAN_POINT('Ctrl Pts',(-23.064779964354,64.1707164063792,66.7003125165312));
#215151=CARTESIAN_POINT('Ctrl Pts',(-23.0529403525713,64.6051802209593,
66.0267421448527));
#215152=CARTESIAN_POINT('Ctrl Pts',(-23.0283692983427,65.6150627386631,
64.7498100788519));
#215153=CARTESIAN_POINT('Ctrl Pts',(-23.0154222549054,66.1928994922378,
64.1532084285951));
#215154=CARTESIAN_POINT('Ctrl Pts',(-22.9905384216501,67.4277670869574,
63.108792457982));
#215155=CARTESIAN_POINT('Ctrl Pts',(-22.9786497998762,68.0785768235615,
62.6567224664561));
#215156=CARTESIAN_POINT('Ctrl Pts',(-22.9417990983282,70.2075954434887,
61.4614169297251));
#215157=CARTESIAN_POINT('Ctrl Pts',(-22.9159564408367,71.7892810380742,
60.9523140322329));
#215158=CARTESIAN_POINT('Ctrl Pts',(-22.8848941253732,73.8228050179139,
60.7213246443219));
#215159=CARTESIAN_POINT('Ctrl Pts',(-22.8788053233582,74.2242359646979,
60.6955106593124));
#215160=CARTESIAN_POINT('Ctrl Pts',(-22.8601629334116,75.4343458629007,
60.6773776226708));
#215161=CARTESIAN_POINT('Ctrl Pts',(-22.8473408710597,76.2422172252888,
60.7453967284844));
#215162=CARTESIAN_POINT('Ctrl Pts',(-22.822646349902,77.8052043610332,61.0335899700925));
#215163=CARTESIAN_POINT('Ctrl Pts',(-22.8107879232795,78.559075510394,61.2483269085615));
#215164=CARTESIAN_POINT('Ctrl Pts',(-22.7739585650263,80.7943332456824,
62.1240879218893));
#215165=CARTESIAN_POINT('Ctrl Pts',(-22.7483049277878,82.1656766468166,
63.0075631318245));
#215166=CARTESIAN_POINT('Ctrl Pts',(-22.6985290046578,84.4883882135417,
65.2585150327436));
#215167=CARTESIAN_POINT('Ctrl Pts',(-22.6726909441824,85.4096795911242,
66.6031378681074));
#215168=CARTESIAN_POINT('Ctrl Pts',(-22.6412225596302,86.2045837909721,
68.4717174240305));
#215169=CARTESIAN_POINT('Ctrl Pts',(-22.6347891537383,86.3477834654584,
68.8633544227412));
#215170=CARTESIAN_POINT('Ctrl Pts',(-22.6081787237398,86.8465827549896,
70.4844388954695));
#215171=CARTESIAN_POINT('Ctrl Pts',(-22.5874829697694,87.0252275441048,
71.7617031373274));
#215172=CARTESIAN_POINT('Ctrl Pts',(-22.5675364824894,86.9998979375059,
73.039443228467));
#215173=CARTESIAN_POINT('',(-22.5675364829333,74.3890640007607,84.9729941181989));
#215174=CARTESIAN_POINT('Origin',(-22.5675364832709,75.,72.98888938658));
#215175=CARTESIAN_POINT('Ctrl Pts',(-22.5675364828275,74.3890709851988,
84.9733322994732));
#215176=CARTESIAN_POINT('Ctrl Pts',(-22.582124664134,74.6718425512144,85.0023542290884));
#215177=CARTESIAN_POINT('Ctrl Pts',(-22.5966303455749,74.9561571119262,
85.0212811334547));
#215178=CARTESIAN_POINT('Ctrl Pts',(-22.6110726647668,75.2412883501049,
85.0300127005125));
#215179=CARTESIAN_POINT('Ctrl Pts',(-22.6255527714039,75.5271656167355,
85.0387671131816));
#215180=CARTESIAN_POINT('Ctrl Pts',(-22.6399691837915,75.813863596684,85.0372727556581));
#215181=CARTESIAN_POINT('Ctrl Pts',(-22.6543411901568,76.1006465657745,
85.0254808020078));
#215182=CARTESIAN_POINT('Ctrl Pts',(-22.6687338767191,76.3878421932063,
85.0136718806553));
#215183=CARTESIAN_POINT('Ctrl Pts',(-22.6830820293737,76.6751228126908,
84.9915357218146));
#215184=CARTESIAN_POINT('Ctrl Pts',(-22.6974050197304,76.9617494722563,
84.9590756102513));
#215185=CARTESIAN_POINT('Ctrl Pts',(-22.711758435899,77.248985002497,84.9265465448437));
#215186=CARTESIAN_POINT('Ctrl Pts',(-22.7260865827534,77.5355635524261,
84.8836496437204));
#215187=CARTESIAN_POINT('Ctrl Pts',(-22.7404089556175,77.8207450199491,
84.8304404268258));
#215188=CARTESIAN_POINT('Ctrl Pts',(-22.744959834007,77.9113603244082,84.8135334046732));
#215189=CARTESIAN_POINT('Ctrl Pts',(-22.7495101294395,78.001834617382,84.7955856168893));
#215190=CARTESIAN_POINT('Ctrl Pts',(-22.7540604673341,78.0921442910401,
84.7765999369994));
#215191=CARTESIAN_POINT('Ctrl Pts',(-22.7682603128447,78.3739658708317,
84.7173529695009));
#215192=CARTESIAN_POINT('Ctrl Pts',(-22.7824601583552,78.6541757753439,
84.6479966081922));
#215193=CARTESIAN_POINT('Ctrl Pts',(-22.7966600038657,78.9320516198127,
84.568636466251));
#215194=CARTESIAN_POINT('Ctrl Pts',(-22.810844131221,79.2096198767334,84.489364169986));
#215195=CARTESIAN_POINT('Ctrl Pts',(-22.8250282585763,79.4848589921676,
84.4001102585485));
#215196=CARTESIAN_POINT('Ctrl Pts',(-22.8392123859315,79.7570558754403,
84.301031531765));
#215197=CARTESIAN_POINT('Ctrl Pts',(-22.8533857637286,80.0290464720533,
84.2020278926142));
#215198=CARTESIAN_POINT('Ctrl Pts',(-22.8675591415256,80.2979992025523,
84.0932143694567));
#215199=CARTESIAN_POINT('Ctrl Pts',(-22.8817325193226,80.5632131543211,
83.9747983265767));
#215200=CARTESIAN_POINT('Ctrl Pts',(-22.8958952491306,80.8282278596376,
83.8564712457451));
#215201=CARTESIAN_POINT('Ctrl Pts',(-22.9100579789387,81.0895091623533,
83.7285561304107));
#215202=CARTESIAN_POINT('Ctrl Pts',(-22.9242207087467,81.3463718930863,
83.5913099327499));
#215203=CARTESIAN_POINT('Ctrl Pts',(-22.9383728914716,81.6030433363624,
83.4541659432843));
#215204=CARTESIAN_POINT('Ctrl Pts',(-22.9525250741965,81.8553025520532,
83.3077048435267));
#215205=CARTESIAN_POINT('Ctrl Pts',(-22.9666772569214,82.1024835994402,
83.1522319476038));
#215206=CARTESIAN_POINT('Ctrl Pts',(-22.9808147545179,82.3494081573861,
82.9969203794065));
#215207=CARTESIAN_POINT('Ctrl Pts',(-22.9949522521143,82.5912648537644,
82.8326158057161));
#215208=CARTESIAN_POINT('Ctrl Pts',(-23.0090897497107,82.8274109397139,
82.6596701102719));
#215209=CARTESIAN_POINT('Ctrl Pts',(-23.0232178305836,83.0633997331586,
82.4868396107309));
#215210=CARTESIAN_POINT('Ctrl Pts',(-23.0373459114565,83.2936853006919,
82.305379608006));
#215211=CARTESIAN_POINT('Ctrl Pts',(-23.0514739923294,83.5176506330175,
82.1156872009436));
#215212=CARTESIAN_POINT('Ctrl Pts',(-23.0655889575854,83.7414080500905,
81.9261708923171));
#215213=CARTESIAN_POINT('Ctrl Pts',(-23.0797039228413,83.9588567506015,
81.7284375853734));
#215214=CARTESIAN_POINT('Ctrl Pts',(-23.0938188880973,84.1694090888517,
81.5229273256865));
#215215=CARTESIAN_POINT('Ctrl Pts',(-23.1038933836672,84.3196899121112,
81.3762452642539));
#215216=CARTESIAN_POINT('Ctrl Pts',(-23.1139678792372,84.4664580709411,
81.2256022909389));
#215217=CARTESIAN_POINT('Ctrl Pts',(-23.1240423748071,84.6095094049711,
81.0711715801781));
#215218=CARTESIAN_POINT('Ctrl Pts',(-23.1381651212178,84.8100432878027,
80.8546857272689));
#215219=CARTESIAN_POINT('Ctrl Pts',(-23.1522876470482,85.0032687820581,
80.630758074656));
#215220=CARTESIAN_POINT('Ctrl Pts',(-23.1663998896936,85.188646319028,80.399892177041));
#215221=CARTESIAN_POINT('Ctrl Pts',(-23.1804719706654,85.3734962947653,
80.1696832948306));
#215222=CARTESIAN_POINT('Ctrl Pts',(-23.1945338268983,85.5505427275545,
79.9325757540413));
#215223=CARTESIAN_POINT('Ctrl Pts',(-23.2085754814538,85.7192839577915,
79.6891085031162));
#215224=CARTESIAN_POINT('Ctrl Pts',(-23.2225931230926,85.8877366202471,
79.4460576104477));
#215225=CARTESIAN_POINT('Ctrl Pts',(-23.2365906320896,86.0479122750287,
79.196668899111));
#215226=CARTESIAN_POINT('Ctrl Pts',(-23.2505580826043,86.1993479138062,
78.9415158489488));
#215227=CARTESIAN_POINT('Ctrl Pts',(-23.2644919766457,86.3504197320023,
78.6869757980239));
#215228=CARTESIAN_POINT('Ctrl Pts',(-23.2783959564609,86.4927933085359,
78.4266992478357));
#215229=CARTESIAN_POINT('Ctrl Pts',(-23.2922601675774,86.6260475700772,
78.1612901952401));
#215230=CARTESIAN_POINT('Ctrl Pts',(-23.2975737953986,86.6771188892796,
78.0595689422945));
#215231=CARTESIAN_POINT('Ctrl Pts',(-23.3028815815996,86.7268510904777,
77.9570941250128));
#215232=CARTESIAN_POINT('Ctrl Pts',(-23.3081829713998,86.7752220564,77.8539010146614));
#215233=CARTESIAN_POINT('Origin',(-54.462516693425,66.6776194928561,69.5544896765311));
#215234=CARTESIAN_POINT('',(-55.3469857987243,58.2763555356819,66.0834535849112));
#215235=CARTESIAN_POINT('',(-55.5509564659454,58.2763798771986,66.0833946695127));
#215236=CARTESIAN_POINT('',(-54.462516693425,58.276355535683,66.0834535849087));
#215237=CARTESIAN_POINT('',(-55.3469876474783,58.2763332605869,66.0835074998374));
#215238=CARTESIAN_POINT('Ctrl Pts',(-55.3469857987243,58.2763555356809,
66.0834535849137));
#215239=CARTESIAN_POINT('Ctrl Pts',(-55.3469865205619,58.2763468384005,
66.0834746357315));
#215240=CARTESIAN_POINT('Ctrl Pts',(-55.34698692564,58.2763419577341,66.0834864489592));
#215241=CARTESIAN_POINT('Ctrl Pts',(-55.3469876474783,58.2763332605869,
66.0835074998374));
#215242=CARTESIAN_POINT('',(-55.5974859706232,58.587245489697,73.6987840815406));
#215243=CARTESIAN_POINT('Ctrl Pts',(-55.5958816852329,58.5872629367333,
73.6988181411009));
#215244=CARTESIAN_POINT('Ctrl Pts',(-55.5642543225698,58.1370349043123,
72.819904863597));
#215245=CARTESIAN_POINT('Ctrl Pts',(-55.5337095641794,57.8330219216737,
71.8734645115865));
#215246=CARTESIAN_POINT('Ctrl Pts',(-55.4920076933008,57.6391257286882,
70.5747597609728));
#215247=CARTESIAN_POINT('Ctrl Pts',(-55.4815921437647,57.6083851839778,
70.2504131744609));
#215248=CARTESIAN_POINT('Ctrl Pts',(-55.4607410660172,57.5817045190807,
69.5965855223251));
#215249=CARTESIAN_POINT('Ctrl Pts',(-55.4503222021789,57.5861334573964,
69.2675652529914));
#215250=CARTESIAN_POINT('Ctrl Pts',(-55.4246589713448,57.6412754033317,
68.4543773063773));
#215251=CARTESIAN_POINT('Ctrl Pts',(-55.409556102247,57.7130444170084,67.9726706635946));
#215252=CARTESIAN_POINT('Ctrl Pts',(-55.3785950880418,57.9352139923274,
67.0155987805645));
#215253=CARTESIAN_POINT('Ctrl Pts',(-55.3627155406804,58.0868340317194,
66.5421780378772));
#215254=CARTESIAN_POINT('Ctrl Pts',(-55.3469876474783,58.2763332605869,
66.0835074998374));
#215255=CARTESIAN_POINT('',(-55.7997963168797,58.5872206257229,73.6987355424395));
#215256=CARTESIAN_POINT('',(-55.7986426798444,58.5872330572012,73.6987598112127));
#215257=CARTESIAN_POINT('Ctrl Pts',(-55.8013975426223,58.587203371073,73.698701857855));
#215258=CARTESIAN_POINT('Ctrl Pts',(-55.7703307595377,58.1370141619865,
72.8198332392404));
#215259=CARTESIAN_POINT('Ctrl Pts',(-55.738609114948,57.8330252662733,71.8734459075331));
#215260=CARTESIAN_POINT('Ctrl Pts',(-55.6969348134739,57.6391324266434,
70.5748181414704));
#215261=CARTESIAN_POINT('Ctrl Pts',(-55.6866939433116,57.608389849271,70.2504736082707));
#215262=CARTESIAN_POINT('Ctrl Pts',(-55.6660029351568,57.5817073282663,
69.5967087730762));
#215263=CARTESIAN_POINT('Ctrl Pts',(-55.6555661301364,57.5861300062074,
69.2677545658034));
#215264=CARTESIAN_POINT('Ctrl Pts',(-55.629490900948,57.6412378757168,68.4547261711262));
#215265=CARTESIAN_POINT('Ctrl Pts',(-55.6137725475604,57.7129722962947,
67.9731075839917));
#215266=CARTESIAN_POINT('Ctrl Pts',(-55.5823353923309,57.9351089370947,
67.0159225655129));
#215267=CARTESIAN_POINT('Ctrl Pts',(-55.5667469045371,58.0867766859385,
66.5423084960526));
#215268=CARTESIAN_POINT('Ctrl Pts',(-55.5509584931268,58.2763555356848,
66.0834535849044));
#215269=CARTESIAN_POINT('Origin',(-54.462516693425,66.6776194928561,69.5544896765311));
#215270=CARTESIAN_POINT('',(-53.7366673713217,58.276355535683,66.0834535849087));
#215271=CARTESIAN_POINT('Ctrl Pts',(-55.5509564659454,58.2763798771986,
66.0833946695127));
#215272=CARTESIAN_POINT('Ctrl Pts',(-55.5293519760116,58.5357993236408,
65.4555106945378));
#215273=CARTESIAN_POINT('Ctrl Pts',(-55.5073947993138,58.8647867368264,
64.8586951524983));
#215274=CARTESIAN_POINT('Ctrl Pts',(-55.4641515221015,59.641820374335,63.7604976646574));
#215275=CARTESIAN_POINT('Ctrl Pts',(-55.4432920030105,60.0850422111019,
63.2607833392951));
#215276=CARTESIAN_POINT('Ctrl Pts',(-55.4034957953534,61.0069687435062,
62.42663124984));
#215277=CARTESIAN_POINT('Ctrl Pts',(-55.3847616723786,61.4710034794686,
62.0809506872743));
#215278=CARTESIAN_POINT('Ctrl Pts',(-55.3493583763049,62.4130313959237,
61.50976809141));
#215279=CARTESIAN_POINT('Ctrl Pts',(-55.3328563273452,62.8840698709349,
61.2772171285064));
#215280=CARTESIAN_POINT('Ctrl Pts',(-55.3066526577161,63.6494857328239,
60.9784691431388));
#215281=CARTESIAN_POINT('Ctrl Pts',(-55.2971246844391,63.9315843450776,
60.884021908299));
#215282=CARTESIAN_POINT('Ctrl Pts',(-55.2686864356095,64.7811364350475,
60.6452191699261));
#215283=CARTESIAN_POINT('Ctrl Pts',(-55.2497306634879,65.3584552015835,
60.5416338472421));
#215284=CARTESIAN_POINT('Ctrl Pts',(-55.2154989596548,66.4315305155951,
60.454474878268));
#215285=CARTESIAN_POINT('Ctrl Pts',(-55.1999659970024,66.9237640368931,
60.454476440718));
#215286=CARTESIAN_POINT('Ctrl Pts',(-55.1694541313247,67.8729393850907,
60.5315775352599));
#215287=CARTESIAN_POINT('Ctrl Pts',(-55.1545490352729,68.3287977518769,
60.6037724386958));
#215288=CARTESIAN_POINT('Ctrl Pts',(-55.12154803696,69.326174810265,60.8405448962535));
#215289=CARTESIAN_POINT('Ctrl Pts',(-55.1038064141092,69.861815684947,61.0216955323755));
#215290=CARTESIAN_POINT('Ctrl Pts',(-55.063999601112,71.0064666283551,61.5317097012693));
#215291=CARTESIAN_POINT('Ctrl Pts',(-55.0417962598498,71.6018231054538,
61.8827158375686));
#215292=CARTESIAN_POINT('Ctrl Pts',(-55.0016951825324,72.600435801391,62.6360073565726));
#215293=CARTESIAN_POINT('Ctrl Pts',(-54.9841070732111,73.0167318888312,
63.0153149028952));
#215294=CARTESIAN_POINT('Ctrl Pts',(-54.956911094595,73.5946968075922,63.6493272193589));
#215295=CARTESIAN_POINT('Ctrl Pts',(-54.947487901833,73.7832613577235,63.877628380177));
#215296=CARTESIAN_POINT('Ctrl Pts',(-54.9190534935064,74.3148611040193,
64.5893308930821));
#215297=CARTESIAN_POINT('Ctrl Pts',(-54.9000080938475,74.6221306839518,
65.0974704511788));
#215298=CARTESIAN_POINT('Ctrl Pts',(-54.8651085839444,75.0997198591477,
66.0958640835209));
#215299=CARTESIAN_POINT('Ctrl Pts',(-54.8489882282909,75.2818881212308,
66.5778429379041));
#215300=CARTESIAN_POINT('Ctrl Pts',(-54.8161206223998,75.5641844346651,
67.572499567804));
#215301=CARTESIAN_POINT('Ctrl Pts',(-54.7994273699867,75.662931038084,68.0836078723164));
#215302=CARTESIAN_POINT('Ctrl Pts',(-54.7659657458026,75.7735740350487,
69.1318698417486));
#215303=CARTESIAN_POINT('Ctrl Pts',(-54.749361305166,75.7826879763227,69.6673118176174));
#215304=CARTESIAN_POINT('Ctrl Pts',(-54.723226180653,75.7237379107367,70.4947770869297));
#215305=CARTESIAN_POINT('Ctrl Pts',(-54.7138851163246,75.6884499719406,
70.7879122301499));
#215306=CARTESIAN_POINT('Ctrl Pts',(-54.6854713453321,75.5386710585311,
71.6684501055308));
#215307=CARTESIAN_POINT('Ctrl Pts',(-54.6664084456847,75.3804204367525,
72.2467631845367));
#215308=CARTESIAN_POINT('Ctrl Pts',(-54.6307736532416,74.9733416854762,
73.3097646919201));
#215309=CARTESIAN_POINT('Ctrl Pts',(-54.6139269174089,74.7355907205756,
73.7959745111832));
#215310=CARTESIAN_POINT('Ctrl Pts',(-54.5842320055116,74.250242856249,74.5985898232458));
#215311=CARTESIAN_POINT('Ctrl Pts',(-54.5715492183761,74.0222783036838,
74.9251093954127));
#215312=CARTESIAN_POINT('Ctrl Pts',(-54.5411564525276,73.4229474861732,
75.6737032519809));
#215313=CARTESIAN_POINT('Ctrl Pts',(-54.5237921110022,73.0324247648255,
76.0783440664095));
#215314=CARTESIAN_POINT('Ctrl Pts',(-54.4849014956126,72.0913866883103,
76.8882046029579));
#215315=CARTESIAN_POINT('Ctrl Pts',(-54.4632576605534,71.5274824055733,
77.2727186656698));
#215316=CARTESIAN_POINT('Ctrl Pts',(-54.424685322754,70.4492787161637,77.8427152235626));
#215317=CARTESIAN_POINT('Ctrl Pts',(-54.4080137844851,69.9510881874095,
78.0518127948251));
#215318=CARTESIAN_POINT('Ctrl Pts',(-54.3697944876016,68.7882585464024,
78.4223285187575));
#215319=CARTESIAN_POINT('Ctrl Pts',(-54.3481195233592,68.1180159738578,
78.5555229109669));
#215320=CARTESIAN_POINT('Ctrl Pts',(-54.3171705141335,67.1431958327321,
78.6374858473127));
#215321=CARTESIAN_POINT('Ctrl Pts',(-54.3078829134622,66.8461257552885,
78.6478491855203));
#215322=CARTESIAN_POINT('Ctrl Pts',(-54.2824028362145,66.0302894258696,
78.6363115634944));
#215323=CARTESIAN_POINT('Ctrl Pts',(-54.2661991957931,65.5130826681465,
78.5845712617889));
#215324=CARTESIAN_POINT('Ctrl Pts',(-54.2405085930586,64.7161012667595,
78.4352019279697));
#215325=CARTESIAN_POINT('Ctrl Pts',(-54.2312097061039,64.4318372928247,
78.3676086043772));
#215326=CARTESIAN_POINT('Ctrl Pts',(-54.1936146716957,63.2963495553903,
78.039093676153));
#215327=CARTESIAN_POINT('Ctrl Pts',(-54.1662304751788,62.4823262415862,
77.6675044830376));
#215328=CARTESIAN_POINT('Ctrl Pts',(-54.118931725783,61.2309279616505,76.8568237565957));
#215329=CARTESIAN_POINT('Ctrl Pts',(-54.099645498139,60.7601649384632,76.4808359800358));
#215330=CARTESIAN_POINT('Ctrl Pts',(-54.0618618311743,59.9011709522606,
75.6428327128146));
#215331=CARTESIAN_POINT('Ctrl Pts',(-54.0431808362138,59.5147800172535,
75.1831579282922));
#215332=CARTESIAN_POINT('Ctrl Pts',(-54.0078044448732,58.8865153419934,
74.2652719391899));
#215333=CARTESIAN_POINT('Ctrl Pts',(-53.9912907602423,58.6330018531612,
73.8179267415289));
#215334=CARTESIAN_POINT('Ctrl Pts',(-53.9656531530641,58.2960950129963,
73.085124826228));
#215335=CARTESIAN_POINT('Ctrl Pts',(-53.9564336345394,58.1865554971259,
72.8128896896097));
#215336=CARTESIAN_POINT('Ctrl Pts',(-53.909615991058,57.6991564449222,71.4090211601971));
#215337=CARTESIAN_POINT('Ctrl Pts',(-53.871311701512,57.5335351163601,70.2161476308588));
#215338=CARTESIAN_POINT('Ctrl Pts',(-53.8015513714535,57.6619983086808,
68.0128916894792));
#215339=CARTESIAN_POINT('Ctrl Pts',(-53.7689112883543,57.8899947788509,
67.018597621202));
#215340=CARTESIAN_POINT('Ctrl Pts',(-53.7366673713217,58.276355535683,66.0834535849087));
#215341=CARTESIAN_POINT('',(-53.5332787937082,58.276355535683,66.0834535849087));
#215342=CARTESIAN_POINT('',(-54.462516693425,58.276355535683,66.0834535849087));
#215343=CARTESIAN_POINT('Ctrl Pts',(-53.5332787937082,58.276355535683,66.0834535849087));
#215344=CARTESIAN_POINT('Ctrl Pts',(-53.5655626775805,57.8867451875228,
67.0264629022823));
#215345=CARTESIAN_POINT('Ctrl Pts',(-53.5970516509312,57.6582247284551,
68.0295019086322));
#215346=CARTESIAN_POINT('Ctrl Pts',(-53.6676791533075,57.5354242743256,
70.2411464584609));
#215347=CARTESIAN_POINT('Ctrl Pts',(-53.7043653688208,57.7042326106747,
71.4332008671241));
#215348=CARTESIAN_POINT('Ctrl Pts',(-53.7518962835288,58.1953384732383,
72.8357123780027));
#215349=CARTESIAN_POINT('Ctrl Pts',(-53.7612947348906,58.3057274807103,
73.1079302723123));
#215350=CARTESIAN_POINT('Ctrl Pts',(-53.7862473225142,58.6365895942013,
73.8223905877668));
#215351=CARTESIAN_POINT('Ctrl Pts',(-53.8016632114925,58.8802475200011,
74.2528015851126));
#215352=CARTESIAN_POINT('Ctrl Pts',(-53.8461401751329,59.6694318506876,
75.4149068128443));
#215353=CARTESIAN_POINT('Ctrl Pts',(-53.875528330836,60.2915996961264,76.0873249387124));
#215354=CARTESIAN_POINT('Ctrl Pts',(-53.9225729919868,61.4550088496706,
77.016929560116));
#215355=CARTESIAN_POINT('Ctrl Pts',(-53.9408334467599,61.9401457211529,
77.3339501839349));
#215356=CARTESIAN_POINT('Ctrl Pts',(-53.977277277685,62.9453814781525,77.8617235755638));
#215357=CARTESIAN_POINT('Ctrl Pts',(-53.995278074046,63.4614421781021,78.07481546934));
#215358=CARTESIAN_POINT('Ctrl Pts',(-54.0296422055439,64.4957981534369,
78.3944612651201));
#215359=CARTESIAN_POINT('Ctrl Pts',(-54.0462059068673,65.0103444407188,
78.5057820273322));
#215360=CARTESIAN_POINT('Ctrl Pts',(-54.0773745812104,65.9757803903488,
78.62847541936));
#215361=CARTESIAN_POINT('Ctrl Pts',(-54.0918530074528,66.4235068791955,
78.6520287760528));
#215362=CARTESIAN_POINT('Ctrl Pts',(-54.1403128133875,67.9273566874276,
78.6200062744246));
#215363=CARTESIAN_POINT('Ctrl Pts',(-54.1732503539562,68.9716109476033,
78.4135544007001));
#215364=CARTESIAN_POINT('Ctrl Pts',(-54.2169174594595,70.2318207791961,
77.9260997599377));
#215365=CARTESIAN_POINT('Ctrl Pts',(-54.2264512621277,70.5013847242329,
77.80646056663));
#215366=CARTESIAN_POINT('Ctrl Pts',(-54.2519427279785,71.2125176461925,
77.4485015693435));
#215367=CARTESIAN_POINT('Ctrl Pts',(-54.2677356448227,71.6409576010732,
77.1863967565669));
#215368=CARTESIAN_POINT('Ctrl Pts',(-54.2998622272673,72.4530656255441,
76.5921373222878));
#215369=CARTESIAN_POINT('Ctrl Pts',(-54.3161473410997,72.8349827406509,
76.2605415590481));
#215370=CARTESIAN_POINT('Ctrl Pts',(-54.3517907845278,73.6051258911224,
75.4703339182632));
#215371=CARTESIAN_POINT('Ctrl Pts',(-54.3707287271076,73.9795165901898,
75.0014946722767));
#215372=CARTESIAN_POINT('Ctrl Pts',(-54.4084654085077,74.6252684857957,
74.0054013195963));
#215373=CARTESIAN_POINT('Ctrl Pts',(-54.4273542154633,74.8967110002721,
73.4816083068042));
#215374=CARTESIAN_POINT('Ctrl Pts',(-54.455941123101,75.2262509370908,72.6591201293671));
#215375=CARTESIAN_POINT('Ctrl Pts',(-54.4655159703041,75.3232727549448,
72.3776994682275));
#215376=CARTESIAN_POINT('Ctrl Pts',(-54.4955040289261,75.5862504835227,
71.4731000360478));
#215377=CARTESIAN_POINT('Ctrl Pts',(-54.5157455546589,75.6998411821233,
70.8367892945741));
#215378=CARTESIAN_POINT('Ctrl Pts',(-54.553591351842,75.7829174207925,69.6585502476179));
#215379=CARTESIAN_POINT('Ctrl Pts',(-54.5709597629142,75.773187030605,69.120975511141));
#215380=CARTESIAN_POINT('Ctrl Pts',(-54.6049064040635,75.6596473684368,
68.0598205514083));
#215381=CARTESIAN_POINT('Ctrl Pts',(-54.6215179372701,75.5571124338195,
67.5381882265612));
#215382=CARTESIAN_POINT('Ctrl Pts',(-54.6544696694349,75.268936383534,66.5420041139739));
#215383=CARTESIAN_POINT('Ctrl Pts',(-54.6707279760388,75.0877995034649,
66.0681362343352));
#215384=CARTESIAN_POINT('Ctrl Pts',(-54.7061676472104,74.6077637515443,
65.0709037461789));
#215385=CARTESIAN_POINT('Ctrl Pts',(-54.7249207921526,74.294433378991,64.5571022944996));
#215386=CARTESIAN_POINT('Ctrl Pts',(-54.7625453618885,73.5760389004118,
63.6053990232175));
#215387=CARTESIAN_POINT('Ctrl Pts',(-54.781435990255,73.1740194179169,63.1688303405712));
#215388=CARTESIAN_POINT('Ctrl Pts',(-54.8191787545644,72.2923760428621,
62.3814911264832));
#215389=CARTESIAN_POINT('Ctrl Pts',(-54.8375876280151,71.8151169441302,
62.0322875949448));
#215390=CARTESIAN_POINT('Ctrl Pts',(-54.8654485062721,71.0519849546158,
61.5806362743694));
#215391=CARTESIAN_POINT('Ctrl Pts',(-54.8748073230891,70.7893271961805,
61.4420751545686));
#215392=CARTESIAN_POINT('Ctrl Pts',(-54.9011635586761,70.0364678518818,
61.0908868353993));
#215393=CARTESIAN_POINT('Ctrl Pts',(-54.9182752578256,69.5336214813441,
60.9082365854418));
#215394=CARTESIAN_POINT('Ctrl Pts',(-54.9521294825018,68.4948704348333,
60.6315063744957));
#215395=CARTESIAN_POINT('Ctrl Pts',(-54.9688975589155,67.9606901776106,
60.5391822805108));
#215396=CARTESIAN_POINT('Ctrl Pts',(-55.0014383011775,66.9307320458366,
60.4546151403975));
#215397=CARTESIAN_POINT('Ctrl Pts',(-55.0171040942008,66.4375248985683,
60.4542627280721));
#215398=CARTESIAN_POINT('Ctrl Pts',(-55.0513165144325,65.3633367342361,
60.5409138398399));
#215399=CARTESIAN_POINT('Ctrl Pts',(-55.069463862521,64.7858546030156,60.6442081211182));
#215400=CARTESIAN_POINT('Ctrl Pts',(-55.0970861308951,63.9360441440502,
60.8826100723));
#215401=CARTESIAN_POINT('Ctrl Pts',(-55.1064307458234,63.6538826901546,
60.9769174549123));
#215402=CARTESIAN_POINT('Ctrl Pts',(-55.1323657620152,62.8897840562762,
61.2747011696298));
#215403=CARTESIAN_POINT('Ctrl Pts',(-55.1490609507609,62.4199951699038,
61.5061833247957));
#215404=CARTESIAN_POINT('Ctrl Pts',(-55.1820030100303,61.522283991715,62.0492269412328));
#215405=CARTESIAN_POINT('Ctrl Pts',(-55.1982907980861,61.0963763792673,
62.3603126797909));
#215406=CARTESIAN_POINT('Ctrl Pts',(-55.2367067708785,60.1755747206076,
63.1641104969289));
#215407=CARTESIAN_POINT('Ctrl Pts',(-55.2589711383476,59.7056367005308,
63.6803953102331));
#215408=CARTESIAN_POINT('Ctrl Pts',(-55.3029292155024,58.8882690149415,
64.8163076429406));
#215409=CARTESIAN_POINT('Ctrl Pts',(-55.3246879318393,58.5450181575742,
65.4331850361657));
#215410=CARTESIAN_POINT('Ctrl Pts',(-55.3469857987243,58.2763555356809,
66.0834535849137));
#215411=CARTESIAN_POINT('Origin',(-54.462516693425,66.6776194928561,69.5544896765311));
#215412=CARTESIAN_POINT('',(-51.7190489450981,58.276355535683,66.0834535849087));
#215413=CARTESIAN_POINT('',(-51.9229031375498,58.2763555332145,66.0834535908833));
#215414=CARTESIAN_POINT('',(-54.462516693425,58.276355535683,66.0834535849087));
#215415=CARTESIAN_POINT('Ctrl Pts',(-51.7190489450981,58.276355535683,66.0834535849086));
#215416=CARTESIAN_POINT('Ctrl Pts',(-51.7297909865996,58.1452767990722,
66.4007153581577));
#215417=CARTESIAN_POINT('Ctrl Pts',(-51.7405829583826,58.0321969222248,
66.7253355117126));
#215418=CARTESIAN_POINT('Ctrl Pts',(-51.7671844604377,57.8013703463813,
67.5327114967342));
#215419=CARTESIAN_POINT('Ctrl Pts',(-51.7830641197152,57.704284738644,68.0200041119831));
#215420=CARTESIAN_POINT('Ctrl Pts',(-51.8080188068358,57.6138010436533,
68.804368958479));
#215421=CARTESIAN_POINT('Ctrl Pts',(-51.817194791681,57.5943064002912,69.0974220773683));
#215422=CARTESIAN_POINT('Ctrl Pts',(-51.8592177464655,57.5701720672488,
70.4382974657879));
#215423=CARTESIAN_POINT('Ctrl Pts',(-51.8927662132002,57.7325169240372,
71.4811043123403));
#215424=CARTESIAN_POINT('Ctrl Pts',(-51.9446543809477,58.2613918916844,
73.0410264061283));
#215425=CARTESIAN_POINT('Ctrl Pts',(-51.9634037738247,58.5096182058567,
73.5884180661377));
#215426=CARTESIAN_POINT('Ctrl Pts',(-52.0016163719075,59.1099745473828,
74.6258755825583));
#215427=CARTESIAN_POINT('Ctrl Pts',(-52.0209296563522,59.4605480935123,
75.113455015466));
#215428=CARTESIAN_POINT('Ctrl Pts',(-52.0588686893564,60.2532267253739,
76.0133347474263));
#215429=CARTESIAN_POINT('Ctrl Pts',(-52.0776830551728,60.6935439328099,
76.4232844203296));
#215430=CARTESIAN_POINT('Ctrl Pts',(-52.1126338797061,61.5634236510416,
77.0855951123235));
#215431=CARTESIAN_POINT('Ctrl Pts',(-52.1285697204729,61.9794687477448,
77.3519202515112));
#215432=CARTESIAN_POINT('Ctrl Pts',(-52.1537182355886,62.6742548444957,
77.7207936911086));
#215433=CARTESIAN_POINT('Ctrl Pts',(-52.1629927917558,62.9399662666728,
77.8457741971178));
#215434=CARTESIAN_POINT('Ctrl Pts',(-52.2098136240202,64.3075493608403,
78.4099093559652));
#215435=CARTESIAN_POINT('Ctrl Pts',(-52.2480628999824,65.4818136675885,
78.643259277779));
#215436=CARTESIAN_POINT('Ctrl Pts',(-52.3040881464568,67.2477783879154,
78.6451840249999));
#215437=CARTESIAN_POINT('Ctrl Pts',(-52.3225131095039,67.8265701659199,
78.5902911792699));
#215438=CARTESIAN_POINT('Ctrl Pts',(-52.3595295668438,68.9539700452295,
78.3732328713076));
#215439=CARTESIAN_POINT('Ctrl Pts',(-52.3778973643229,69.5004860289171,
78.2137877221895));
#215440=CARTESIAN_POINT('Ctrl Pts',(-52.4140545301813,70.5576359137233,
77.7945606084078));
#215441=CARTESIAN_POINT('Ctrl Pts',(-52.4320745666133,71.0658550902994,
77.5355097194339));
#215442=CARTESIAN_POINT('Ctrl Pts',(-52.4674002329574,71.9927932922179,
76.9475651068214));
#215443=CARTESIAN_POINT('Ctrl Pts',(-52.4845761304828,72.4135503083147,
76.6261047834406));
#215444=CARTESIAN_POINT('Ctrl Pts',(-52.5179670940298,73.1857150076729,
75.9216717201334));
#215445=CARTESIAN_POINT('Ctrl Pts',(-52.5342433170281,73.5370541495871,
75.5415152241367));
#215446=CARTESIAN_POINT('Ctrl Pts',(-52.5662763717388,74.1521757655702,
74.7502628796883));
#215447=CARTESIAN_POINT('Ctrl Pts',(-52.581950416172,74.4189726128819,74.3436958487136));
#215448=CARTESIAN_POINT('Ctrl Pts',(-52.6169307455104,74.9394935738121,
73.3923854213503));
#215449=CARTESIAN_POINT('Ctrl Pts',(-52.6358128319037,75.1743424436644,
72.8398680566229));
#215450=CARTESIAN_POINT('Ctrl Pts',(-52.6642021536451,75.4411186332504,
71.9870297038072));
#215451=CARTESIAN_POINT('Ctrl Pts',(-52.6736001389969,75.5153668048818,
71.7016713015829));
#215452=CARTESIAN_POINT('Ctrl Pts',(-52.7005200820087,75.6869461038813,
70.8802940815234));
#215453=CARTESIAN_POINT('Ctrl Pts',(-52.7181571859923,75.7501682284098,
70.3384477093478));
#215454=CARTESIAN_POINT('Ctrl Pts',(-52.7539696199146,75.7798597050836,
69.2129442652462));
#215455=CARTESIAN_POINT('Ctrl Pts',(-52.7721897099371,75.7393861088041,
68.6315478859276));
#215456=CARTESIAN_POINT('Ctrl Pts',(-52.8065558247652,75.5619672989915,
67.5685563511103));
#215457=CARTESIAN_POINT('Ctrl Pts',(-52.8225403875164,75.4403337548272,
67.0866159433306));
#215458=CARTESIAN_POINT('Ctrl Pts',(-52.861854617124,75.0431684405423,65.9235202423042));
#215459=CARTESIAN_POINT('Ctrl Pts',(-52.8846025666856,74.7233642266042,
65.2611991817657));
#215460=CARTESIAN_POINT('Ctrl Pts',(-52.9238158502275,74.0571175243991,
64.2231705879217));
#215461=CARTESIAN_POINT('Ctrl Pts',(-52.9398941888697,73.7523626374077,
63.8249208396988));
#215462=CARTESIAN_POINT('Ctrl Pts',(-52.9766967184228,72.9768367067566,
62.9682840108232));
#215463=CARTESIAN_POINT('Ctrl Pts',(-52.9969933203808,72.4861149505907,
62.5316963366546));
#215464=CARTESIAN_POINT('Ctrl Pts',(-53.0334867491832,71.5460372241218,
61.8618144110017));
#215465=CARTESIAN_POINT('Ctrl Pts',(-53.0494388776599,71.1161258988521,
61.6060056457897));
#215466=CARTESIAN_POINT('Ctrl Pts',(-53.0979197277774,69.747581117297,60.9374950055504));
#215467=CARTESIAN_POINT('Ctrl Pts',(-53.1293484776116,68.7584477903061,
60.6467731515279));
#215468=CARTESIAN_POINT('Ctrl Pts',(-53.1712046497495,67.4513676644178,
60.4926926534559));
#215469=CARTESIAN_POINT('Ctrl Pts',(-53.1805221582027,67.1594503901744,
60.4724914816801));
#215470=CARTESIAN_POINT('Ctrl Pts',(-53.2070124229002,66.3213843424688,
60.4550213283923));
#215471=CARTESIAN_POINT('Ctrl Pts',(-53.2238855276084,65.7757832089102,
60.4928163888376));
#215472=CARTESIAN_POINT('Ctrl Pts',(-53.2576262207124,64.714181512971,60.6632305163589));
#215473=CARTESIAN_POINT('Ctrl Pts',(-53.2744219506812,64.1998171398207,
60.7926368877312));
#215474=CARTESIAN_POINT('Ctrl Pts',(-53.3098179404078,63.1462982245024,
61.1579359757481));
#215475=CARTESIAN_POINT('Ctrl Pts',(-53.3280076005827,62.6127810599663,
61.4028372586244));
#215476=CARTESIAN_POINT('Ctrl Pts',(-53.3556258902385,61.8491815284432,
61.847079914686));
#215477=CARTESIAN_POINT('Ctrl Pts',(-53.3649702061992,61.599336313249,62.0093576969857));
#215478=CARTESIAN_POINT('Ctrl Pts',(-53.3898639392663,60.9604045687096,
62.4704870885438));
#215479=CARTESIAN_POINT('Ctrl Pts',(-53.4055080051247,60.5867619892367,
62.7890561532968));
#215480=CARTESIAN_POINT('Ctrl Pts',(-53.437438933781,59.8718678681658,63.5060318544576));
#215481=CARTESIAN_POINT('Ctrl Pts',(-53.4535879884448,59.5356605431283,
63.9069659835912));
#215482=CARTESIAN_POINT('Ctrl Pts',(-53.4858087684677,58.9459658308018,
64.7476712063653));
#215483=CARTESIAN_POINT('Ctrl Pts',(-53.5018112337239,58.6910935895951,
65.1842073837295));
#215484=CARTESIAN_POINT('Ctrl Pts',(-53.5230144855764,58.4039439418394,
65.7859480088557));
#215485=CARTESIAN_POINT('Ctrl Pts',(-53.5281604188844,58.3381254207757,
65.9339463209189));
#215486=CARTESIAN_POINT('Ctrl Pts',(-53.5332787937082,58.276355535683,66.0834535849087));
#215487=CARTESIAN_POINT('Ctrl Pts',(-53.7366673713217,58.276355535683,66.0834535849087));
#215488=CARTESIAN_POINT('Ctrl Pts',(-53.7311924318832,58.3419586614738,
65.9246683802505));
#215489=CARTESIAN_POINT('Ctrl Pts',(-53.7257379418286,58.4121273391153,
65.7675881140914));
#215490=CARTESIAN_POINT('Ctrl Pts',(-53.7012784846244,58.7467389739019,
65.0723349768854));
#215491=CARTESIAN_POINT('Ctrl Pts',(-53.68226410661,59.0594466298307,64.5592909907682));
#215492=CARTESIAN_POINT('Ctrl Pts',(-53.6440710268083,59.7730809282138,
63.6131281747025));
#215493=CARTESIAN_POINT('Ctrl Pts',(-53.6251642980075,60.1701800452071,
63.1806622316127));
#215494=CARTESIAN_POINT('Ctrl Pts',(-53.5909939976614,60.9706951840624,
62.4622180755958));
#215495=CARTESIAN_POINT('Ctrl Pts',(-53.575474758473,61.3611218065782,62.1650275357795));
#215496=CARTESIAN_POINT('Ctrl Pts',(-53.543512083073,62.1990648694285,61.6281266777756));
#215497=CARTESIAN_POINT('Ctrl Pts',(-53.5271071357313,62.6465335046139,
61.3914618649718));
#215498=CARTESIAN_POINT('Ctrl Pts',(-53.4940927068657,63.5919501222416,
60.9882198705243));
#215499=CARTESIAN_POINT('Ctrl Pts',(-53.4776501716035,64.0893400320841,
60.8250483118051));
#215500=CARTESIAN_POINT('Ctrl Pts',(-53.4515011764791,64.8874480684872,
60.6374817478447));
#215501=CARTESIAN_POINT('Ctrl Pts',(-53.441970765598,65.1800727413696,60.5836984088002));
#215502=CARTESIAN_POINT('Ctrl Pts',(-53.4135047195804,66.0556830139493,
60.4668081126836));
#215503=CARTESIAN_POINT('Ctrl Pts',(-53.3945384953424,66.6427094200249,
60.4456171533872));
#215504=CARTESIAN_POINT('Ctrl Pts',(-53.3570293722958,67.8210826162455,
60.517054256725));
#215505=CARTESIAN_POINT('Ctrl Pts',(-53.33824063788,68.4095227784195,60.6111539031541));
#215506=CARTESIAN_POINT('Ctrl Pts',(-53.3037808204978,69.4466278606999,
60.8832650107809));
#215507=CARTESIAN_POINT('Ctrl Pts',(-53.2882999316967,69.8984319767658,
61.0407412355476));
#215508=CARTESIAN_POINT('Ctrl Pts',(-53.2565712011872,70.8080872919673,
61.4406270428976));
#215509=CARTESIAN_POINT('Ctrl Pts',(-53.2403824324189,71.2618801399946,
61.688099632371));
#215510=CARTESIAN_POINT('Ctrl Pts',(-53.2040930968364,72.2133226175424,
62.3173872972681));
#215511=CARTESIAN_POINT('Ctrl Pts',(-53.183939473219,72.697496313979,62.714845756158));
#215512=CARTESIAN_POINT('Ctrl Pts',(-53.1462258971347,73.5268006904438,
63.552417439899));
#215513=CARTESIAN_POINT('Ctrl Pts',(-53.1289153258879,73.8797380436296,
63.9808333396457));
#215514=CARTESIAN_POINT('Ctrl Pts',(-53.1020034726543,74.357971412337,64.6832433562619));
#215515=CARTESIAN_POINT('Ctrl Pts',(-53.0925914463726,74.5124263739884,
64.9357619592791));
#215516=CARTESIAN_POINT('Ctrl Pts',(-53.0641411353165,74.9390844612585,
65.7164939021594));
#215517=CARTESIAN_POINT('Ctrl Pts',(-53.0450838003077,75.1721256350204,
66.2642924312581));
#215518=CARTESIAN_POINT('Ctrl Pts',(-53.0092068472208,75.5135324920802,
67.3513984616382));
#215519=CARTESIAN_POINT('Ctrl Pts',(-52.9921213947985,75.6298054510112,
67.8855577007919));
#215520=CARTESIAN_POINT('Ctrl Pts',(-52.9591460990218,75.7584613520713,
68.9147142293431));
#215521=CARTESIAN_POINT('Ctrl Pts',(-52.943370378706,75.7797701191653,69.4066621395435));
#215522=CARTESIAN_POINT('Ctrl Pts',(-52.911095693656,75.7412819636644,70.4246802732259));
#215523=CARTESIAN_POINT('Ctrl Pts',(-52.8947343811169,75.6755823410685,
70.9487203678477));
#215524=CARTESIAN_POINT('Ctrl Pts',(-52.8688560994954,75.5028705016795,
71.7525088367728));
#215525=CARTESIAN_POINT('Ctrl Pts',(-52.8595254225974,75.4268994499431,
72.0377218640758));
#215526=CARTESIAN_POINT('Ctrl Pts',(-52.8311270335815,75.1552027324261,
72.8888691141832));
#215527=CARTESIAN_POINT('Ctrl Pts',(-52.8120780996225,74.9173443869597,
73.4396479332205));
#215528=CARTESIAN_POINT('Ctrl Pts',(-52.7773610510153,74.3790085656657,
74.4103703648679));
#215529=CARTESIAN_POINT('Ctrl Pts',(-52.7614170741286,74.0936192220105,
74.8359587895104));
#215530=CARTESIAN_POINT('Ctrl Pts',(-52.7298730908476,73.470066651144,75.6148892266165));
#215531=CARTESIAN_POINT('Ctrl Pts',(-52.7143505704592,73.1362089965511,
75.9695032833215));
#215532=CARTESIAN_POINT('Ctrl Pts',(-52.682531006495,72.3886843419833,76.645699858249));
#215533=CARTESIAN_POINT('Ctrl Pts',(-52.6664022672045,71.9723579023323,
76.9617342519526));
#215534=CARTESIAN_POINT('Ctrl Pts',(-52.6322390103953,71.0507229972334,
77.5437483372261));
#215535=CARTESIAN_POINT('Ctrl Pts',(-52.6142123432411,70.5428224261473,
77.8014577569882));
#215536=CARTESIAN_POINT('Ctrl Pts',(-52.578175097805,69.486223313356,78.2183942640377));
#215537=CARTESIAN_POINT('Ctrl Pts',(-52.5605556197902,68.9398896018736,
78.3768269863344));
#215538=CARTESIAN_POINT('Ctrl Pts',(-52.5246847482757,67.8131002898757,
78.5919603651484));
#215539=CARTESIAN_POINT('Ctrl Pts',(-52.5063744298448,67.2347576412136,
78.6459569374812));
#215540=CARTESIAN_POINT('Ctrl Pts',(-52.4502646779272,65.4693496476904,
78.6416089451388));
#215541=CARTESIAN_POINT('Ctrl Pts',(-52.4139257778699,64.2954222045958,
78.4066522721589));
#215542=CARTESIAN_POINT('Ctrl Pts',(-52.3668074694311,62.9285056104644,
77.8406030075759));
#215543=CARTESIAN_POINT('Ctrl Pts',(-52.3574542691322,62.6628429772777,
77.7151943835185));
#215544=CARTESIAN_POINT('Ctrl Pts',(-52.3314026873732,61.9334863960864,
77.3266448147371));
#215545=CARTESIAN_POINT('Ctrl Pts',(-52.3148571809506,61.4861912750879,
77.0352832186051));
#215546=CARTESIAN_POINT('Ctrl Pts',(-52.2790825333981,60.5946063699471,
76.3358437178863));
#215547=CARTESIAN_POINT('Ctrl Pts',(-52.2598405536161,60.1600952896223,
75.9193679903975));
#215548=CARTESIAN_POINT('Ctrl Pts',(-52.2199383850187,59.3443572919324,
74.9656871986867));
#215549=CARTESIAN_POINT('Ctrl Pts',(-52.1996324508646,58.9738516611268,
74.4237562134378));
#215550=CARTESIAN_POINT('Ctrl Pts',(-52.159830619563,58.3814408224882,73.3178356340863));
#215551=CARTESIAN_POINT('Ctrl Pts',(-52.1405028579493,58.1511829363678,
72.7621712009817));
#215552=CARTESIAN_POINT('Ctrl Pts',(-52.1044482223889,57.8231178466625,
71.6783057699179));
#215553=CARTESIAN_POINT('Ctrl Pts',(-52.087817524682,57.7139444648366,71.1561539683518));
#215554=CARTESIAN_POINT('Ctrl Pts',(-52.0420519854254,57.5436879712687,
69.7238411266884));
#215555=CARTESIAN_POINT('Ctrl Pts',(-52.0126390402298,57.5725696407299,
68.8092010332304));
#215556=CARTESIAN_POINT('Ctrl Pts',(-51.9655607911578,57.8409930992436,
67.3461209787052));
#215557=CARTESIAN_POINT('Ctrl Pts',(-51.9472899306698,57.9991045718153,
66.789307985591));
#215558=CARTESIAN_POINT('Ctrl Pts',(-51.9267839175271,58.2308768134648,
66.1950996618202));
#215559=CARTESIAN_POINT('Ctrl Pts',(-51.9248440301999,58.2533412531563,
66.1391571437214));
#215560=CARTESIAN_POINT('Ctrl Pts',(-51.9229031375498,58.276355530746,66.083453596858));
#215561=CARTESIAN_POINT('Origin',(-54.462516693425,66.6776194928561,69.5544896765311));
#215562=CARTESIAN_POINT('',(-49.9050113929448,58.276355535683,66.0834535849087));
#215563=CARTESIAN_POINT('',(-50.1089321285242,58.276355535683,66.0834535849087));
#215564=CARTESIAN_POINT('',(-54.462516693425,58.276355535683,66.0834535849087));
#215565=CARTESIAN_POINT('Ctrl Pts',(-49.9050113929448,58.276355535683,66.0834535849087));
#215566=CARTESIAN_POINT('Ctrl Pts',(-49.9146376833535,58.1605312070027,
66.363793728952));
#215567=CARTESIAN_POINT('Ctrl Pts',(-49.9243138080825,58.0587404443406,
66.6499272247979));
#215568=CARTESIAN_POINT('Ctrl Pts',(-49.9515580498989,57.8121177239994,
67.471427229109));
#215569=CARTESIAN_POINT('Ctrl Pts',(-49.9687688148612,57.7016626603582,
68.0155058286091));
#215570=CARTESIAN_POINT('Ctrl Pts',(-50.0043152237878,57.5785750352218,
69.1409824503157));
#215571=CARTESIAN_POINT('Ctrl Pts',(-50.0226790664577,57.5706958512298,
69.7203997185111));
#215572=CARTESIAN_POINT('Ctrl Pts',(-50.0700859037347,57.6919873595473,
71.2010948169454));
#215573=CARTESIAN_POINT('Ctrl Pts',(-50.0981155088323,57.901108321059,72.089396074077));
#215574=CARTESIAN_POINT('Ctrl Pts',(-50.1427607988033,58.4223748973441,
73.3918995671297));
#215575=CARTESIAN_POINT('Ctrl Pts',(-50.158698840709,58.6437477551811,73.8360406501164));
#215576=CARTESIAN_POINT('Ctrl Pts',(-50.1838000986255,59.0521723087971,
74.511108620969));
#215577=CARTESIAN_POINT('Ctrl Pts',(-50.193034235206,59.2162213075673,74.7547833431456));
#215578=CARTESIAN_POINT('Ctrl Pts',(-50.2398490858395,60.1046299937437,
75.9456002244812));
#215579=CARTESIAN_POINT('Ctrl Pts',(-50.2781407182629,60.9985364195232,
76.7516063210605));
#215580=CARTESIAN_POINT('Ctrl Pts',(-50.353271030748,63.0396463716975,77.9685817028853));
#215581=CARTESIAN_POINT('Ctrl Pts',(-50.3914240457153,64.165605894035,78.3704740552869));
#215582=CARTESIAN_POINT('Ctrl Pts',(-50.4451731795604,65.842168222641,78.6204871531557));
#215583=CARTESIAN_POINT('Ctrl Pts',(-50.461353595056,66.3528744867564,78.6531063296549));
#215584=CARTESIAN_POINT('Ctrl Pts',(-50.4943139559629,67.378474783785,78.6321176486079));
#215585=CARTESIAN_POINT('Ctrl Pts',(-50.511036904118,67.8915159290587,78.5778473333094));
#215586=CARTESIAN_POINT('Ctrl Pts',(-50.5432465355915,68.8801642663428,
78.3873851183966));
#215587=CARTESIAN_POINT('Ctrl Pts',(-50.5587389673875,69.354788650321,78.2552951422154));
#215588=CARTESIAN_POINT('Ctrl Pts',(-50.583940284417,70.0958202741404,77.9826496449354));
#215589=CARTESIAN_POINT('Ctrl Pts',(-50.5934933843494,70.3700261754071,
77.8661747027161));
#215590=CARTESIAN_POINT('Ctrl Pts',(-50.6219859413768,71.1652013490339,
77.4812779949944));
#215591=CARTESIAN_POINT('Ctrl Pts',(-50.6409237167971,71.6664960982399,
77.1757422003745));
#215592=CARTESIAN_POINT('Ctrl Pts',(-50.6763378807529,72.5574722536808,
76.5068886530519));
#215593=CARTESIAN_POINT('Ctrl Pts',(-50.6930710464352,72.9515749083736,
76.1534290051907));
#215594=CARTESIAN_POINT('Ctrl Pts',(-50.7260223099667,73.6523580210189,
75.4050648915069));
#215595=CARTESIAN_POINT('Ctrl Pts',(-50.7421497152092,73.9616699917789,
75.0151501759862));
#215596=CARTESIAN_POINT('Ctrl Pts',(-50.7748067987056,74.5273539247205,
74.1678795193282));
#215597=CARTESIAN_POINT('Ctrl Pts',(-50.7912098810465,74.779226674521,73.7096867698027));
#215598=CARTESIAN_POINT('Ctrl Pts',(-50.8283330401849,75.2505826166256,
72.6443390962046));
#215599=CARTESIAN_POINT('Ctrl Pts',(-50.8491231513436,75.4476356806003,
72.0303058935975));
#215600=CARTESIAN_POINT('Ctrl Pts',(-50.8874941927951,75.6904825234003,
70.8595051234087));
#215601=CARTESIAN_POINT('Ctrl Pts',(-50.9048197603625,75.7531415644071,
70.3092523220413));
#215602=CARTESIAN_POINT('Ctrl Pts',(-50.9317880127308,75.772030474855,69.4604356269019));
#215603=CARTESIAN_POINT('Ctrl Pts',(-50.9412446810199,75.7641302129071,
69.1640047887181));
#215604=CARTESIAN_POINT('Ctrl Pts',(-50.9696989533205,75.6971824565697,
68.2794181303715));
#215605=CARTESIAN_POINT('Ctrl Pts',(-50.9887247546056,75.5952797477216,
67.6960827496695));
#215606=CARTESIAN_POINT('Ctrl Pts',(-51.0250367061594,75.2883452243661,
66.5885792041862));
#215607=CARTESIAN_POINT('Ctrl Pts',(-51.0425797657269,75.0899108323937,
66.0652813064536));
#215608=CARTESIAN_POINT('Ctrl Pts',(-51.0775110688586,74.6092042509539,
65.0815682163962));
#215609=CARTESIAN_POINT('Ctrl Pts',(-51.0947969734681,74.3314962344145,
64.6214136999578));
#215610=CARTESIAN_POINT('Ctrl Pts',(-51.1279166649473,73.7140401509426,
63.7771410902842));
#215611=CARTESIAN_POINT('Ctrl Pts',(-51.1438020793535,73.3791882248007,
63.3918640769683));
#215612=CARTESIAN_POINT('Ctrl Pts',(-51.1792414538755,72.5752140017154,
62.6102914883718));
#215613=CARTESIAN_POINT('Ctrl Pts',(-51.1988411835993,72.094690709306,62.2292704752158));
#215614=CARTESIAN_POINT('Ctrl Pts',(-51.2357170665386,71.1169936572975,
61.6032010717346));
#215615=CARTESIAN_POINT('Ctrl Pts',(-51.2527597871759,70.6285324823468,
61.3495324946817));
#215616=CARTESIAN_POINT('Ctrl Pts',(-51.287916534422,69.5938927469422,60.9261632208876));
#215617=CARTESIAN_POINT('Ctrl Pts',(-51.3060043217276,69.0485740446644,
60.7606719443466));
#215618=CARTESIAN_POINT('Ctrl Pts',(-51.3421598214664,67.934464811533,60.533808294777));
#215619=CARTESIAN_POINT('Ctrl Pts',(-51.3598341688668,67.3681329371056,
60.4728847533926));
#215620=CARTESIAN_POINT('Ctrl Pts',(-51.4002746967788,66.0763747861971,
60.4555165893947));
#215621=CARTESIAN_POINT('Ctrl Pts',(-51.4232630002298,65.3543436284031,
60.5321993747226));
#215622=CARTESIAN_POINT('Ctrl Pts',(-51.4636153297325,64.1118883107877,
60.8166375859706));
#215623=CARTESIAN_POINT('Ctrl Pts',(-51.4806582044059,63.586988269362,60.9882165208285));
#215624=CARTESIAN_POINT('Ctrl Pts',(-51.5060913559596,62.8411300632569,
61.3095628688017));
#215625=CARTESIAN_POINT('Ctrl Pts',(-51.5142995740101,62.6059561312179,
61.4231290637743));
#215626=CARTESIAN_POINT('Ctrl Pts',(-51.5379184528011,61.9478040952251,
61.7766731081608));
#215627=CARTESIAN_POINT('Ctrl Pts',(-51.5534318886634,61.5387509664118,
62.0406616117935));
#215628=CARTESIAN_POINT('Ctrl Pts',(-51.5780070871286,60.9191133937169,
62.5149219064706));
#215629=CARTESIAN_POINT('Ctrl Pts',(-51.5871702059434,60.6942752001404,
62.705000669812));
#215630=CARTESIAN_POINT('Ctrl Pts',(-51.6290211295816,59.7134012114723,
63.6194479110496));
#215631=CARTESIAN_POINT('Ctrl Pts',(-51.6623823994008,59.0767722619121,
64.4601621641708));
#215632=CARTESIAN_POINT('Ctrl Pts',(-51.7031473001465,58.4805834086687,
65.6171256403115));
#215633=CARTESIAN_POINT('Ctrl Pts',(-51.7110858807856,58.373524068264,65.8482677588338));
#215634=CARTESIAN_POINT('Ctrl Pts',(-51.7190489450981,58.276355535683,66.0834535849086));
#215635=CARTESIAN_POINT('Ctrl Pts',(-51.9229031375498,58.276355530746,66.083453596858));
#215636=CARTESIAN_POINT('Ctrl Pts',(-51.9066584569547,58.4689780276898,
65.6172318680371));
#215637=CARTESIAN_POINT('Ctrl Pts',(-51.8903671818083,58.7001181376414,
65.1677498718171));
#215638=CARTESIAN_POINT('Ctrl Pts',(-51.8567750261386,59.2600464270107,
64.2711065545253));
#215639=CARTESIAN_POINT('Ctrl Pts',(-51.8393335771109,59.5947731060437,
63.8301720239684));
#215640=CARTESIAN_POINT('Ctrl Pts',(-51.8064926448627,60.2848652969986,
63.0750287758916));
#215641=CARTESIAN_POINT('Ctrl Pts',(-51.7912378456738,60.6287658210384,
62.7528659666705));
#215642=CARTESIAN_POINT('Ctrl Pts',(-51.7540899580665,61.5303275168572,
62.0309817897715));
#215643=CARTESIAN_POINT('Ctrl Pts',(-51.7326467220305,62.1112109213727,
61.6648951873634));
#215644=CARTESIAN_POINT('Ctrl Pts',(-51.6958595553788,63.144881879531,61.1661829224993));
#215645=CARTESIAN_POINT('Ctrl Pts',(-51.6808649979164,63.5768836711471,
60.9970743285224));
#215646=CARTESIAN_POINT('Ctrl Pts',(-51.6475424666645,64.5645712707152,
60.6951006710349));
#215647=CARTESIAN_POINT('Ctrl Pts',(-51.6295815813372,65.1237046144991,
60.5801318943607));
#215648=CARTESIAN_POINT('Ctrl Pts',(-51.6020861452689,65.9822427504294,
60.4862893635124));
#215649=CARTESIAN_POINT('Ctrl Pts',(-51.5926856426807,66.2759498740023,
60.4685408819194));
#215650=CARTESIAN_POINT('Ctrl Pts',(-51.5658158243222,67.111431733078,60.4586485236363));
#215651=CARTESIAN_POINT('Ctrl Pts',(-51.548234974849,67.6523594844531,60.5006281173763));
#215652=CARTESIAN_POINT('Ctrl Pts',(-51.5116901283149,68.782621052906,60.690859871711));
#215653=CARTESIAN_POINT('Ctrl Pts',(-51.4926875717132,69.3674141003031,
60.8504690468474));
#215654=CARTESIAN_POINT('Ctrl Pts',(-51.4573922890429,70.3966496544497,
61.2451115053121));
#215655=CARTESIAN_POINT('Ctrl Pts',(-51.4412970110226,70.8458665983852,
61.4611181558444));
#215656=CARTESIAN_POINT('Ctrl Pts',(-51.4053923165603,71.8123189681,62.027741444852));
#215657=CARTESIAN_POINT('Ctrl Pts',(-51.3859380166555,72.3157147916126,
62.3970486157093));
#215658=CARTESIAN_POINT('Ctrl Pts',(-51.3500832598207,73.1511722389079,
63.1531936849593));
#215659=CARTESIAN_POINT('Ctrl Pts',(-51.3338769617531,73.496155691826,63.5219916343335));
#215660=CARTESIAN_POINT('Ctrl Pts',(-51.2984535933001,74.1811404506166,
64.3885382682181));
#215661=CARTESIAN_POINT('Ctrl Pts',(-51.2796655308721,74.5059119262911,
64.8953350221338));
#215662=CARTESIAN_POINT('Ctrl Pts',(-51.2420078521155,75.0465997312735,
65.9573889766624));
#215663=CARTESIAN_POINT('Ctrl Pts',(-51.2231169997875,75.2628083268442,
66.5092501744975));
#215664=CARTESIAN_POINT('Ctrl Pts',(-51.1853034100103,75.5849402611807,
67.6470109015176));
#215665=CARTESIAN_POINT('Ctrl Pts',(-51.1668269068216,75.6901165191788,
68.2302007927246));
#215666=CARTESIAN_POINT('Ctrl Pts',(-51.1388976071206,75.7619025294626,
69.1150714484619));
#215667=CARTESIAN_POINT('Ctrl Pts',(-51.1295337372783,75.7714024648193,
69.4116741122853));
#215668=CARTESIAN_POINT('Ctrl Pts',(-51.1030906296812,75.7573250217166,
70.2440195880202));
#215669=CARTESIAN_POINT('Ctrl Pts',(-51.0858958042147,75.700899034983,70.7779825825479));
#215670=CARTESIAN_POINT('Ctrl Pts',(-51.0520446944832,75.4942747147157,
71.8315741008777));
#215671=CARTESIAN_POINT('Ctrl Pts',(-51.0353585289282,75.3441563616161,
72.3490678790225));
#215672=CARTESIAN_POINT('Ctrl Pts',(-51.0027307823126,74.9687850928878,
73.3139374287333));
#215673=CARTESIAN_POINT('Ctrl Pts',(-50.9868874434386,74.7506283652911,
73.7620299782548));
#215674=CARTESIAN_POINT('Ctrl Pts',(-50.9524775979752,74.1982749419539,
74.6937510060772));
#215675=CARTESIAN_POINT('Ctrl Pts',(-50.9343115959941,73.851662385872,75.1674547776925));
#215676=CARTESIAN_POINT('Ctrl Pts',(-50.9066674140993,73.2640931755435,
75.8263331465221));
#215677=CARTESIAN_POINT('Ctrl Pts',(-50.8973217425598,73.0555284415371,
76.0383104446865));
#215678=CARTESIAN_POINT('Ctrl Pts',(-50.8710903428876,72.4457864247927,
76.6000898098844));
#215679=CARTESIAN_POINT('Ctrl Pts',(-50.854099884282,72.0237359436145,76.9254649701064));
#215680=CARTESIAN_POINT('Ctrl Pts',(-50.8182450177606,71.0611827188948,
77.5411462999966));
#215681=CARTESIAN_POINT('Ctrl Pts',(-50.7993634060826,70.5148462065648,
77.8175403811517));
#215682=CARTESIAN_POINT('Ctrl Pts',(-50.7652851830786,69.5065847435217,
78.2059023661214));
#215683=CARTESIAN_POINT('Ctrl Pts',(-50.7503208419736,69.0558068048182,
78.3405130464432));
#215684=CARTESIAN_POINT('Ctrl Pts',(-50.7112164587197,67.8481684378219,
78.6013405062761));
#215685=CARTESIAN_POINT('Ctrl Pts',(-50.6876878372036,67.0822485392285,
78.6677751324582));
#215686=CARTESIAN_POINT('Ctrl Pts',(-50.6488921054763,65.855090021021,78.6190672115604));
#215687=CARTESIAN_POINT('Ctrl Pts',(-50.6341413594616,65.3951515695407,
78.5655047520926));
#215688=CARTESIAN_POINT('Ctrl Pts',(-50.5963750843635,64.2249825391195,
78.33779364235));
#215689=CARTESIAN_POINT('Ctrl Pts',(-50.5738938554618,63.5280612165873,
78.112651914641));
#215690=CARTESIAN_POINT('Ctrl Pts',(-50.5368219599937,62.4639131746578,
77.6210734798956));
#215691=CARTESIAN_POINT('Ctrl Pts',(-50.5226929158353,62.0763273093222,
77.406444917496));
#215692=CARTESIAN_POINT('Ctrl Pts',(-50.4751077633651,60.8242974683905,
76.5884753004597));
#215693=CARTESIAN_POINT('Ctrl Pts',(-50.4426746836312,60.0494402382401,
75.86365452694));
#215694=CARTESIAN_POINT('Ctrl Pts',(-50.3996305760705,59.2396772045108,
74.7882500359777));
#215695=CARTESIAN_POINT('Ctrl Pts',(-50.3902460389154,59.0747993299534,
74.545717979835));
#215696=CARTESIAN_POINT('Ctrl Pts',(-50.3650565516947,58.6605054081258,
73.8680062214918));
#215697=CARTESIAN_POINT('Ctrl Pts',(-50.3494191532467,58.434900102059,73.4194768297401));
#215698=CARTESIAN_POINT('Ctrl Pts',(-50.304431063181,57.9031719808351,72.1011313949032));
#215699=CARTESIAN_POINT('Ctrl Pts',(-50.2747514895586,57.6905336946499,
71.2002732586477));
#215700=CARTESIAN_POINT('Ctrl Pts',(-50.2274030973064,57.570396953899,69.7058979582394));
#215701=CARTESIAN_POINT('Ctrl Pts',(-50.2091218482721,57.5792338353981,
69.12577343449));
#215702=CARTESIAN_POINT('Ctrl Pts',(-50.1724353252622,57.7054849798947,
67.9897595629765));
#215703=CARTESIAN_POINT('Ctrl Pts',(-50.1542207163723,57.8198572872672,
67.4360846626437));
#215704=CARTESIAN_POINT('Ctrl Pts',(-50.1271781319156,58.0690980510039,
66.6209286899905));
#215705=CARTESIAN_POINT('Ctrl Pts',(-50.1180768395745,58.1664030290617,
66.3495816246336));
#215706=CARTESIAN_POINT('Ctrl Pts',(-50.1089321285242,58.276355535683,66.0834535849087));
#215707=CARTESIAN_POINT('Origin',(-61.5936228798467,66.6770802411476,69.5524554490054));
#215708=CARTESIAN_POINT('',(-62.6023291620188,58.2758162839759,66.0814193573862));
#215709=CARTESIAN_POINT('',(-62.8075051404766,58.2758467353478,66.0813456540807));
#215710=CARTESIAN_POINT('',(-61.5936228798467,58.2758162839768,66.0814193573839));
#215711=CARTESIAN_POINT('',(-62.6023317437084,58.2757853463631,66.0814942394464));
#215712=CARTESIAN_POINT('Ctrl Pts',(-62.6023291620188,58.2758162839749,
66.0814193573885));
#215713=CARTESIAN_POINT('Ctrl Pts',(-62.6023301287421,58.2758046991418,
66.0814473972124));
#215714=CARTESIAN_POINT('Ctrl Pts',(-62.6023310954659,58.2757931144483,
66.0814754370963));
#215715=CARTESIAN_POINT('Ctrl Pts',(-62.6023320621901,58.2757815298943,
66.0815034770401));
#215716=CARTESIAN_POINT('',(-62.7290132089978,57.5946335568169,69.9232336695064));
#215717=CARTESIAN_POINT('Ctrl Pts',(-62.7269877844547,57.5945799011542,
69.9232858703779));
#215718=CARTESIAN_POINT('Ctrl Pts',(-62.7059767167849,57.5678166503396,
69.2677915511051));
#215719=CARTESIAN_POINT('Ctrl Pts',(-62.6852394928937,57.6120930723197,
68.6113136984255));
#215720=CARTESIAN_POINT('Ctrl Pts',(-62.6544240531954,57.7834457997657,
67.6449849877674));
#215721=CARTESIAN_POINT('Ctrl Pts',(-62.6442290356214,57.8574078132741,
67.3279207418244));
#215722=CARTESIAN_POINT('Ctrl Pts',(-62.6234162513844,58.040356981802,66.6984486864255));
#215723=CARTESIAN_POINT('Ctrl Pts',(-62.6128525065426,58.1497114542633,
66.3866500398473));
#215724=CARTESIAN_POINT('Ctrl Pts',(-62.6023317437084,58.2757853463631,
66.0814942394464));
#215725=CARTESIAN_POINT('',(-62.9304638037219,57.5945049974057,69.9232129291766));
#215726=CARTESIAN_POINT('',(-62.9299583493521,57.5945773164048,69.9232225584337));
#215727=CARTESIAN_POINT('Ctrl Pts',(-62.9325038108326,57.5945747891981,
69.9231606454938));
#215728=CARTESIAN_POINT('Ctrl Pts',(-62.9116762545802,57.5675772732949,
69.2617048911573));
#215729=CARTESIAN_POINT('Ctrl Pts',(-62.8907033963375,57.6129186405627,
68.5992795600948));
#215730=CARTESIAN_POINT('Ctrl Pts',(-62.85911645307,57.7866934413854,67.6304133938896));
#215731=CARTESIAN_POINT('Ctrl Pts',(-62.8487672427708,57.8604331702437,
67.3163960962927));
#215732=CARTESIAN_POINT('Ctrl Pts',(-62.8281485912862,58.0423315204011,
66.6928186356272));
#215733=CARTESIAN_POINT('Ctrl Pts',(-62.8178556351171,58.1508626454292,
66.3838559993944));
#215734=CARTESIAN_POINT('Ctrl Pts',(-62.8075076622655,58.2758162839768,
66.0814193573839));
#215735=CARTESIAN_POINT('Origin',(-61.5936228798467,66.6770802411476,69.5524554490054));
#215736=CARTESIAN_POINT('',(-60.993278523103,58.2758162839768,66.0814193573839));
#215737=CARTESIAN_POINT('Ctrl Pts',(-62.8075051404766,58.2758467353478,
66.0813456540807));
#215738=CARTESIAN_POINT('Ctrl Pts',(-62.7827585996791,58.5746718414298,
65.3580900839858));
#215739=CARTESIAN_POINT('Ctrl Pts',(-62.7575867818917,58.9656412879929,
64.6764534053843));
#215740=CARTESIAN_POINT('Ctrl Pts',(-62.7076612405528,59.9079275399909,
63.4361951464086));
#215741=CARTESIAN_POINT('Ctrl Pts',(-62.6834874527537,60.453825861867,62.8815352655141));
#215742=CARTESIAN_POINT('Ctrl Pts',(-62.6418528328706,61.4740133937407,
62.0805138507002));
#215743=CARTESIAN_POINT('Ctrl Pts',(-62.6249116919099,61.9115880273756,
61.7941115554923));
#215744=CARTESIAN_POINT('Ctrl Pts',(-62.5926328302465,62.8008280984047,
61.3158394451234));
#215745=CARTESIAN_POINT('Ctrl Pts',(-62.5772771158596,63.2482362687151,
61.1197685888594));
#215746=CARTESIAN_POINT('Ctrl Pts',(-62.5522217402567,63.9905960020285,
60.8633383483942));
#215747=CARTESIAN_POINT('Ctrl Pts',(-62.5426740764964,64.2765858947229,
60.7800225781601));
#215748=CARTESIAN_POINT('Ctrl Pts',(-62.5141917610593,65.1358303777023,
60.5748768688081));
#215749=CARTESIAN_POINT('Ctrl Pts',(-62.4952519587902,65.7173373284889,
60.494239432827));
#215750=CARTESIAN_POINT('Ctrl Pts',(-62.4586443494421,66.8678934254916,
60.4467937668689));
#215751=CARTESIAN_POINT('Ctrl Pts',(-62.4407218880458,67.4341768201499,
60.4763172308115));
#215752=CARTESIAN_POINT('Ctrl Pts',(-62.4067121422934,68.4796855133982,
60.6294031440396));
#215753=CARTESIAN_POINT('Ctrl Pts',(-62.3907689417157,68.9587860956276,
60.7397335511125));
#215754=CARTESIAN_POINT('Ctrl Pts',(-62.3588267718022,69.9100311455759,
61.0416056107918));
#215755=CARTESIAN_POINT('Ctrl Pts',(-62.342864162994,70.3797482102385,61.2351967274013));
#215756=CARTESIAN_POINT('Ctrl Pts',(-62.3064768420909,71.3942058159256,
61.7563561812658));
#215757=CARTESIAN_POINT('Ctrl Pts',(-62.2859769344181,71.9257607533805,
62.1038465208793));
#215758=CARTESIAN_POINT('Ctrl Pts',(-62.2480189698315,72.8422683937824,
62.8501602504118));
#215759=CARTESIAN_POINT('Ctrl Pts',(-62.2308009241964,73.2354454508964,
63.2343739445442));
#215760=CARTESIAN_POINT('Ctrl Pts',(-62.1951974733025,73.9622073414218,
64.0859907161967));
#215761=CARTESIAN_POINT('Ctrl Pts',(-62.1768342962594,74.2910940309015,
64.5542461698788));
#215762=CARTESIAN_POINT('Ctrl Pts',(-62.1402813141876,74.8541666534339,
65.5418640199265));
#215763=CARTESIAN_POINT('Ctrl Pts',(-62.1224831178287,75.087935532165,66.0585888868009));
#215764=CARTESIAN_POINT('Ctrl Pts',(-62.0817639257673,75.5068656162761,
67.275558289919));
#215765=CARTESIAN_POINT('Ctrl Pts',(-62.0586270483711,75.6596174315433,
67.9829420927733));
#215766=CARTESIAN_POINT('Ctrl Pts',(-62.0175060546965,75.7801278767569,
69.2636845606806));
#215767=CARTESIAN_POINT('Ctrl Pts',(-61.99987197195,75.7804715495623,69.8301848231031));
#215768=CARTESIAN_POINT('Ctrl Pts',(-61.9726963351648,75.7009037857973,
70.6869416792319));
#215769=CARTESIAN_POINT('Ctrl Pts',(-61.9633329853358,75.6593103335437,
70.9793370954806));
#215770=CARTESIAN_POINT('Ctrl Pts',(-61.9349406935905,75.4911724330965,
71.8536028518237));
#215771=CARTESIAN_POINT('Ctrl Pts',(-61.915867253474,75.3216558936171,72.4255773475958));
#215772=CARTESIAN_POINT('Ctrl Pts',(-61.881532200228,74.9100731217729,73.4376279523369));
#215773=CARTESIAN_POINT('Ctrl Pts',(-61.8659985082016,74.6851893526394,
73.8822273586314));
#215774=CARTESIAN_POINT('Ctrl Pts',(-61.833264459617,74.1444827544418,74.7635106413054));
#215775=CARTESIAN_POINT('Ctrl Pts',(-61.8160830782531,73.823960567157,75.1950871383287));
#215776=CARTESIAN_POINT('Ctrl Pts',(-61.7822572443624,73.1135399396358,
75.9932919904183));
#215777=CARTESIAN_POINT('Ctrl Pts',(-61.7657762630245,72.7256138598147,
76.3588960487237));
#215778=CARTESIAN_POINT('Ctrl Pts',(-61.7312540836744,71.8628284640962,
77.0397003278377));
#215779=CARTESIAN_POINT('Ctrl Pts',(-61.7132339311628,71.3858258825639,
77.3485136648221));
#215780=CARTESIAN_POINT('Ctrl Pts',(-61.6772032272859,70.3799360315444,
77.8735394216446));
#215781=CARTESIAN_POINT('Ctrl Pts',(-61.6595801463188,69.853192360704,78.0884905207624));
#215782=CARTESIAN_POINT('Ctrl Pts',(-61.6237352249995,68.7564464131023,
78.4203673109301));
#215783=CARTESIAN_POINT('Ctrl Pts',(-61.6054645307211,68.1883319352046,
78.5346450594559));
#215784=CARTESIAN_POINT('Ctrl Pts',(-61.5494981065453,66.4354979537243,
78.7161279993807));
#215785=CARTESIAN_POINT('Ctrl Pts',(-61.5132749974563,65.2452066928191,
78.6067908307184));
#215786=CARTESIAN_POINT('Ctrl Pts',(-61.4439774707116,63.1528917115972,
77.9906812584831));
#215787=CARTESIAN_POINT('Ctrl Pts',(-61.4133567723254,62.2492109921292,
77.5535520320839));
#215788=CARTESIAN_POINT('Ctrl Pts',(-61.372511416718,61.195681842865,76.8098067289323));
#215789=CARTESIAN_POINT('Ctrl Pts',(-61.3631996323689,60.9650192984978,
76.6296890041399));
#215790=CARTESIAN_POINT('Ctrl Pts',(-61.3251373636124,60.0585343567079,
75.8486100481436));
#215791=CARTESIAN_POINT('Ctrl Pts',(-61.2973225302177,59.465488555232,75.1595635958174));
#215792=CARTESIAN_POINT('Ctrl Pts',(-61.2495715790222,58.6638192095476,
73.8858242979422));
#215793=CARTESIAN_POINT('Ctrl Pts',(-61.2302911091849,58.3949457432561,
73.3467533407717));
#215794=CARTESIAN_POINT('Ctrl Pts',(-61.1925163314495,57.9681958687,72.2251964261833));
#215795=CARTESIAN_POINT('Ctrl Pts',(-61.1738295834256,57.8110238947228,
71.6456003758838));
#215796=CARTESIAN_POINT('Ctrl Pts',(-61.1385558059292,57.6277603155242,
70.5519746426347));
#215797=CARTESIAN_POINT('Ctrl Pts',(-61.1221533967664,57.5859523878683,
70.0429852871717));
#215798=CARTESIAN_POINT('Ctrl Pts',(-61.0966297976346,57.5876547657298,
69.2399596518455));
#215799=CARTESIAN_POINT('Ctrl Pts',(-61.0874121528402,57.602464249246,68.9469350082234));
#215800=CARTESIAN_POINT('Ctrl Pts',(-61.0501113182517,57.7193395302956,
67.7687383620738));
#215801=CARTESIAN_POINT('Ctrl Pts',(-61.0216484906896,57.9369166166898,
66.9016890073447));
#215802=CARTESIAN_POINT('Ctrl Pts',(-60.9932785231031,58.2758162839768,
66.0814193573839));
#215803=CARTESIAN_POINT('',(-60.7885639123434,58.2758162839768,66.0814193573839));
#215804=CARTESIAN_POINT('',(-61.5936228798467,58.2758162839768,66.0814193573839));
#215805=CARTESIAN_POINT('Ctrl Pts',(-60.7885639123434,58.2758162839768,
66.0814193573839));
#215806=CARTESIAN_POINT('Ctrl Pts',(-60.8165473472842,57.9369608312523,
66.9015819908227));
#215807=CARTESIAN_POINT('Ctrl Pts',(-60.8442152543235,57.7193974192671,
67.7685080573625));
#215808=CARTESIAN_POINT('Ctrl Pts',(-60.8820788621428,57.6024881991777,
68.9465773614098));
#215809=CARTESIAN_POINT('Ctrl Pts',(-60.8914689841111,57.5876670022784,
69.2396014868228));
#215810=CARTESIAN_POINT('Ctrl Pts',(-60.9169257724154,57.5859338443228,
70.0423343359673));
#215811=CARTESIAN_POINT('Ctrl Pts',(-60.9328238216174,57.627672833315,70.5510319849962));
#215812=CARTESIAN_POINT('Ctrl Pts',(-60.9775352109377,57.8608162618331,
71.9434798747403));
#215813=CARTESIAN_POINT('Ctrl Pts',(-61.0066469216558,58.1415007775707,
72.8062831413013));
#215814=CARTESIAN_POINT('Ctrl Pts',(-61.0534060471856,58.8027561945617,
74.1304666122758));
#215815=CARTESIAN_POINT('Ctrl Pts',(-61.071649492068,59.1095844962329,74.6215940641858));
#215816=CARTESIAN_POINT('Ctrl Pts',(-61.1078882009044,59.7961967047495,
75.5179145969811));
#215817=CARTESIAN_POINT('Ctrl Pts',(-61.1257064779507,60.1705752195452,
75.9241636522968));
#215818=CARTESIAN_POINT('Ctrl Pts',(-61.1587188475635,60.9416661273783,
76.6216060002487));
#215819=CARTESIAN_POINT('Ctrl Pts',(-61.1741112087812,61.3296977850336,
76.9195013345673));
#215820=CARTESIAN_POINT('Ctrl Pts',(-61.208855899165,62.2422348086538,77.5098160220488));
#215821=CARTESIAN_POINT('Ctrl Pts',(-61.228270860995,62.7755579818415,77.7844390413501));
#215822=CARTESIAN_POINT('Ctrl Pts',(-61.2642438684955,63.8191658535208,
78.1974642400836));
#215823=CARTESIAN_POINT('Ctrl Pts',(-61.2807198566024,64.3221095717221,
78.3477933918406));
#215824=CARTESIAN_POINT('Ctrl Pts',(-61.3283324670262,65.783379249252,78.6501568821174));
#215825=CARTESIAN_POINT('Ctrl Pts',(-61.3597192290084,66.7568480676607,
78.693599470245));
#215826=CARTESIAN_POINT('Ctrl Pts',(-61.4281169265037,68.8961192897166,
78.446827760361));
#215827=CARTESIAN_POINT('Ctrl Pts',(-61.4664202734848,70.0356498357558,
78.0820517269475));
#215828=CARTESIAN_POINT('Ctrl Pts',(-61.5224094342196,71.5794231561345,
77.2291128902152));
#215829=CARTESIAN_POINT('Ctrl Pts',(-61.5407709521873,72.0579438740127,
76.901627865946));
#215830=CARTESIAN_POINT('Ctrl Pts',(-61.5776828394934,72.937946573046,76.1670772939815));
#215831=CARTESIAN_POINT('Ctrl Pts',(-61.5960250555282,73.3387725571802,
75.7632155309537));
#215832=CARTESIAN_POINT('Ctrl Pts',(-61.6320400842896,74.0596370682187,
74.8862341888564));
#215833=CARTESIAN_POINT('Ctrl Pts',(-61.6499384167133,74.3781316996655,
74.4150828476952));
#215834=CARTESIAN_POINT('Ctrl Pts',(-61.6855335246671,74.9114633913786,
73.4408177884735));
#215835=CARTESIAN_POINT('Ctrl Pts',(-61.7031153881128,75.1290740315015,
72.9418853840914));
#215836=CARTESIAN_POINT('Ctrl Pts',(-61.7368933998136,75.4651026724446,
71.9336157900771));
#215837=CARTESIAN_POINT('Ctrl Pts',(-61.7531680691965,75.5868127939801,
71.4275376897543));
#215838=CARTESIAN_POINT('Ctrl Pts',(-61.7857433181699,75.7403393205686,
70.4139912827648));
#215839=CARTESIAN_POINT('Ctrl Pts',(-61.8019744568581,75.77422227908,69.9086982042928));
#215840=CARTESIAN_POINT('Ctrl Pts',(-61.8373848076953,75.7560669168494,
68.8029687331288));
#215841=CARTESIAN_POINT('Ctrl Pts',(-61.8561363593999,75.6867723500449,
68.2051688784902));
#215842=CARTESIAN_POINT('Ctrl Pts',(-61.8937598743357,75.4331074672901,
67.040131079595));
#215843=CARTESIAN_POINT('Ctrl Pts',(-61.9126494440181,75.2509564655508,
66.4753756260395));
#215844=CARTESIAN_POINT('Ctrl Pts',(-61.9503885951798,74.7802486150384,
65.3911999619088));
#215845=CARTESIAN_POINT('Ctrl Pts',(-61.968795420232,74.4931720024805,64.8741972967853));
#215846=CARTESIAN_POINT('Ctrl Pts',(-61.9966562260526,73.9894400224411,
64.1444245840252));
#215847=CARTESIAN_POINT('Ctrl Pts',(-62.0060150486286,73.8089918375229,
63.9085880933557));
#215848=CARTESIAN_POINT('Ctrl Pts',(-62.0324031298607,73.271861586515,63.2735741056103));
#215849=CARTESIAN_POINT('Ctrl Pts',(-62.0495464558552,72.8910095255566,
62.8964371446764));
#215850=CARTESIAN_POINT('Ctrl Pts',(-62.0819374027553,72.0991586949565,
62.2398540898828));
#215851=CARTESIAN_POINT('Ctrl Pts',(-62.0972543547778,71.6940639775007,
61.9562095194195));
#215852=CARTESIAN_POINT('Ctrl Pts',(-62.129099833235,70.8197771606755,61.4446186812144));
#215853=CARTESIAN_POINT('Ctrl Pts',(-62.1456004240847,70.3499645204559,
61.221257008585));
#215854=CARTESIAN_POINT('Ctrl Pts',(-62.1807049022731,69.3148423125416,
60.8338002075288));
#215855=CARTESIAN_POINT('Ctrl Pts',(-62.1989001788807,68.7474384662482,
60.6819222598256));
#215856=CARTESIAN_POINT('Ctrl Pts',(-62.2265394851784,67.8758442776549,
60.53686683111));
#215857=CARTESIAN_POINT('Ctrl Pts',(-62.235884325555,67.5800952234876,60.502459011075));
#215858=CARTESIAN_POINT('Ctrl Pts',(-62.2613184522206,66.7771778698587,
60.4488021160657));
#215859=CARTESIAN_POINT('Ctrl Pts',(-62.2775119444156,66.2692202919945,
60.4573923659707));
#215860=CARTESIAN_POINT('Ctrl Pts',(-62.3087892996319,65.280280849755,60.5571639643559));
#215861=CARTESIAN_POINT('Ctrl Pts',(-62.3238535962417,64.8006291363324,
60.6448601307839));
#215862=CARTESIAN_POINT('Ctrl Pts',(-62.3473142461334,64.0775673291655,
60.8380822025366));
#215863=CARTESIAN_POINT('Ctrl Pts',(-62.3555518205413,63.8278589097013,
60.916501249032));
#215864=CARTESIAN_POINT('Ctrl Pts',(-62.380624321535,63.0830599950247,61.186225556435));
#215865=CARTESIAN_POINT('Ctrl Pts',(-62.3975665990526,62.6010054913371,
61.4101948690422));
#215866=CARTESIAN_POINT('Ctrl Pts',(-62.4359648220922,61.5402401777661,
62.0209777247797));
#215867=CARTESIAN_POINT('Ctrl Pts',(-62.4574452932637,60.9808127241981,
62.4346733468827));
#215868=CARTESIAN_POINT('Ctrl Pts',(-62.4995279255077,60.0106482273865,
63.3404009052831));
#215869=CARTESIAN_POINT('Ctrl Pts',(-62.5197370473476,59.5939033403095,
63.8201297648542));
#215870=CARTESIAN_POINT('Ctrl Pts',(-62.5498902602688,59.0418253317485,
64.6087332374532));
#215871=CARTESIAN_POINT('Ctrl Pts',(-62.5601640094589,58.8679605841081,
64.8882131315763));
#215872=CARTESIAN_POINT('Ctrl Pts',(-62.5810561208043,58.5484688232857,
65.4699227574098));
#215873=CARTESIAN_POINT('Ctrl Pts',(-62.5916621719048,58.4036453073442,
65.7720231602976));
#215874=CARTESIAN_POINT('Ctrl Pts',(-62.6023291620188,58.2758162839749,
66.0814193573885));
#215875=CARTESIAN_POINT('Origin',(-61.5936228798467,66.6770802411476,69.5524554490054));
#215876=CARTESIAN_POINT('',(-58.974273988216,58.2758162753068,66.0814193783688));
#215877=CARTESIAN_POINT('',(-59.1795703763521,58.275816290262,66.0814193421713));
#215878=CARTESIAN_POINT('',(-61.5936228798467,58.2758162839768,66.0814193573839));
#215879=CARTESIAN_POINT('Ctrl Pts',(-58.9742739875024,58.2758162752982,
66.0814193783896));
#215880=CARTESIAN_POINT('Ctrl Pts',(-58.9911038138538,58.0715593177539,
66.5758010506857));
#215881=CARTESIAN_POINT('Ctrl Pts',(-59.0081251209979,57.9113071395147,
67.0873265040614));
#215882=CARTESIAN_POINT('Ctrl Pts',(-59.0633622145753,57.5418582166893,
68.7763376497993));
#215883=CARTESIAN_POINT('Ctrl Pts',(-59.1001880361245,57.5189956372051,
69.9815383517207));
#215884=CARTESIAN_POINT('Ctrl Pts',(-59.1769506047935,57.9415126003576,
72.3381137918141));
#215885=CARTESIAN_POINT('Ctrl Pts',(-59.2141023465274,58.3852626414375,
73.4659946727289));
#215886=CARTESIAN_POINT('Ctrl Pts',(-59.2804378253646,59.5019504018343,
75.1995352173277));
#215887=CARTESIAN_POINT('Ctrl Pts',(-59.3074037942511,60.0693039913178,
75.8539871979905));
#215888=CARTESIAN_POINT('Ctrl Pts',(-59.3567993348846,61.2376021988887,
76.8675410777012));
#215889=CARTESIAN_POINT('Ctrl Pts',(-59.379048121626,61.8040067040322,77.2564515187191));
#215890=CARTESIAN_POINT('Ctrl Pts',(-59.4101600368057,62.665999914094,77.7148996843177));
#215891=CARTESIAN_POINT('Ctrl Pts',(-59.4193782968166,62.929738949022,77.8392941371504));
#215892=CARTESIAN_POINT('Ctrl Pts',(-59.4473201316425,63.7426779625362,
78.1759638046202));
#215893=CARTESIAN_POINT('Ctrl Pts',(-59.4661662278638,64.3069346828376,
78.3477956756026));
#215894=CARTESIAN_POINT('Ctrl Pts',(-59.494716409947,65.1731993978973,78.5221155288877));
#215895=CARTESIAN_POINT('Ctrl Pts',(-59.5042582022465,65.4652465181133,
78.5662183241016));
#215896=CARTESIAN_POINT('Ctrl Pts',(-59.5289780514452,66.2340909413064,
78.6442759770403));
#215897=CARTESIAN_POINT('Ctrl Pts',(-59.5440323453596,66.7123245113538,
78.6549936863834));
#215898=CARTESIAN_POINT('Ctrl Pts',(-59.5674248403096,67.4441681822125,
78.6136986733134));
#215899=CARTESIAN_POINT('Ctrl Pts',(-59.57561052084,67.6984335496873,78.5885712552251));
#215900=CARTESIAN_POINT('Ctrl Pts',(-59.6019313915972,68.5076002506141,
78.4740133444789));
#215901=CARTESIAN_POINT('Ctrl Pts',(-59.6201701450891,69.0554059998211,
78.3438477157663));
#215902=CARTESIAN_POINT('Ctrl Pts',(-59.6512970835278,69.9811404253804,
78.0309581578981));
#215903=CARTESIAN_POINT('Ctrl Pts',(-59.6644189740089,70.3650219160779,
77.8711638200664));
#215904=CARTESIAN_POINT('Ctrl Pts',(-59.6940122776478,71.1947236006463,
77.4570336833513));
#215905=CARTESIAN_POINT('Ctrl Pts',(-59.7105209139073,71.6326795192761,
77.1900915948514));
#215906=CARTESIAN_POINT('Ctrl Pts',(-59.7463544810056,72.5287828863619,
76.534224948955));
#215907=CARTESIAN_POINT('Ctrl Pts',(-59.7652519010259,72.9756540813877,
76.1339068713837));
#215908=CARTESIAN_POINT('Ctrl Pts',(-59.7936257547136,73.5791854720248,
75.4750636182617));
#215909=CARTESIAN_POINT('Ctrl Pts',(-59.8030263097735,73.7677339744296,
75.2479775613684));
#215910=CARTESIAN_POINT('Ctrl Pts',(-59.829384649667,74.2614816435717,74.5907088525881));
#215911=CARTESIAN_POINT('Ctrl Pts',(-59.8464597131991,74.5408036513983,
74.1425531515353));
#215912=CARTESIAN_POINT('Ctrl Pts',(-59.878925249695,75.0023994276505,73.2348115483913));
#215913=CARTESIAN_POINT('Ctrl Pts',(-59.8943318225078,75.1892173679364,
72.7795614929971));
#215914=CARTESIAN_POINT('Ctrl Pts',(-59.9272701617939,75.5040722447159,
71.791144133584));
#215915=CARTESIAN_POINT('Ctrl Pts',(-59.9447982877611,75.6225906238265,
71.2569639124577));
#215916=CARTESIAN_POINT('Ctrl Pts',(-59.9813618271596,75.7684301293272,
70.1263829293776));
#215917=CARTESIAN_POINT('Ctrl Pts',(-59.9999665523777,75.7865036260607,
69.5313429436259));
#215918=CARTESIAN_POINT('Ctrl Pts',(-60.0280581225139,75.7264397887533,
68.6436455588647));
#215919=CARTESIAN_POINT('Ctrl Pts',(-60.0374337131608,75.6920722794492,
68.3496418588188));
#215920=CARTESIAN_POINT('Ctrl Pts',(-60.0645239597047,75.5523465640712,
67.5114130736661));
#215921=CARTESIAN_POINT('Ctrl Pts',(-60.0823494810074,75.4115013628887,
66.9744516372166));
#215922=CARTESIAN_POINT('Ctrl Pts',(-60.1195679273578,75.0095579413445,
65.8660093281956));
#215923=CARTESIAN_POINT('Ctrl Pts',(-60.1390205161559,74.7364157729125,
65.3019042324966));
#215924=CARTESIAN_POINT('Ctrl Pts',(-60.1752363848728,74.1359845803842,
64.3312910834203));
#215925=CARTESIAN_POINT('Ctrl Pts',(-60.1917865248931,73.8275063813815,
63.9162143441071));
#215926=CARTESIAN_POINT('Ctrl Pts',(-60.2231695427559,73.169996016359,63.1729511098809));
#215927=CARTESIAN_POINT('Ctrl Pts',(-60.2379525545349,72.8269866850854,
62.8416666264532));
#215928=CARTESIAN_POINT('Ctrl Pts',(-60.2715699470804,72.000872928672,62.160565141108));
#215929=CARTESIAN_POINT('Ctrl Pts',(-60.2904595269813,71.5061378533602,
61.8282726276767));
#215930=CARTESIAN_POINT('Ctrl Pts',(-60.3279705543224,70.466353576707,61.269085250254));
#215931=CARTESIAN_POINT('Ctrl Pts',(-60.3461616892115,69.9245495720509,
61.0420640976496));
#215932=CARTESIAN_POINT('Ctrl Pts',(-60.3738156326458,69.0806136893065,
60.7808665141748));
#215933=CARTESIAN_POINT('Ctrl Pts',(-60.3831614764318,68.7924150616687,
60.7069423313539));
#215934=CARTESIAN_POINT('Ctrl Pts',(-60.4090671731526,67.9899813686328,
60.542581068052));
#215935=CARTESIAN_POINT('Ctrl Pts',(-60.4257343281076,67.4707817327735,
60.4820867986367));
#215936=CARTESIAN_POINT('Ctrl Pts',(-60.4578635074531,66.4485183276783,
60.451463132225));
#215937=CARTESIAN_POINT('Ctrl Pts',(-60.4733677527643,65.9473848483799,
60.4778837818462));
#215938=CARTESIAN_POINT('Ctrl Pts',(-60.5045987239673,64.9614375358099,
60.6120977543049));
#215939=CARTESIAN_POINT('Ctrl Pts',(-60.5202690540823,64.4781399883781,
60.7185390121146));
#215940=CARTESIAN_POINT('Ctrl Pts',(-60.554551462598,63.4460687161177,61.0358292203882));
#215941=CARTESIAN_POINT('Ctrl Pts',(-60.5727682647228,62.9041818506703,
61.2616412093218));
#215942=CARTESIAN_POINT('Ctrl Pts',(-60.6098300336945,61.8593306985531,
61.8208395923513));
#215943=CARTESIAN_POINT('Ctrl Pts',(-60.6287747734129,61.3601399426014,
62.155244787345));
#215944=CARTESIAN_POINT('Ctrl Pts',(-60.6855784598625,59.9815838596318,
63.2908375436745));
#215945=CARTESIAN_POINT('Ctrl Pts',(-60.7219797380526,59.2222036094218,
64.2174450661231));
#215946=CARTESIAN_POINT('Ctrl Pts',(-60.76945264915,58.5197435485548,65.5302025555244));
#215947=CARTESIAN_POINT('Ctrl Pts',(-60.7790684393769,58.3907983366686,
65.8031178504267));
#215948=CARTESIAN_POINT('Ctrl Pts',(-60.7885639123434,58.2758162839768,
66.0814193573839));
#215949=CARTESIAN_POINT('Ctrl Pts',(-60.9932785231031,58.2758162839768,
66.0814193573839));
#215950=CARTESIAN_POINT('Ctrl Pts',(-60.9836574173467,58.3907473120026,
65.8032413500608));
#215951=CARTESIAN_POINT('Ctrl Pts',(-60.9741335746798,58.5196312768922,
65.5304403346781));
#215952=CARTESIAN_POINT('Ctrl Pts',(-60.9270767181657,59.2219598823845,
64.2177907759692));
#215953=CARTESIAN_POINT('Ctrl Pts',(-60.8888495077651,59.9812789843619,
63.2911689638367));
#215954=CARTESIAN_POINT('Ctrl Pts',(-60.8322317794888,61.3597740556388,
62.1555056628057));
#215955=CARTESIAN_POINT('Ctrl Pts',(-60.8132145108189,61.8589609984774,
61.8210694669032));
#215956=CARTESIAN_POINT('Ctrl Pts',(-60.7750208682129,62.9037877655204,
61.2618208629497));
#215957=CARTESIAN_POINT('Ctrl Pts',(-60.7561185972566,63.4456715069743,
61.0359790233309));
#215958=CARTESIAN_POINT('Ctrl Pts',(-60.721830257427,64.477378335204,60.7187498471518));
#215959=CARTESIAN_POINT('Ctrl Pts',(-60.7061891359679,64.9602845356755,
60.6123406655328));
#215960=CARTESIAN_POINT('Ctrl Pts',(-60.6737997807858,65.9593277127877,
60.4761687121902));
#215961=CARTESIAN_POINT('Ctrl Pts',(-60.6570865355666,66.474199778111,60.4500939653191));
#215962=CARTESIAN_POINT('Ctrl Pts',(-60.6240285138677,67.5037440395565,
60.4853864037791));
#215963=CARTESIAN_POINT('Ctrl Pts',(-60.6078027272971,68.0165517576591,
60.5468497135589));
#215964=CARTESIAN_POINT('Ctrl Pts',(-60.5818657107383,68.8126432717828,
60.7118007384783));
#215965=CARTESIAN_POINT('Ctrl Pts',(-60.5723287908477,69.1007688658806,
60.786410917448));
#215966=CARTESIAN_POINT('Ctrl Pts',(-60.5438441306482,69.9444216977029,
61.0496571008243));
#215967=CARTESIAN_POINT('Ctrl Pts',(-60.5248796499584,70.4859273562666,
61.2780491295712));
#215968=CARTESIAN_POINT('Ctrl Pts',(-60.4896548250228,71.4612757412648,
61.8055946956147));
#215969=CARTESIAN_POINT('Ctrl Pts',(-60.4731368229985,71.8986014309954,
62.0933608398127));
#215970=CARTESIAN_POINT('Ctrl Pts',(-60.4427964367961,72.6411614875954,
62.6794382413306));
#215971=CARTESIAN_POINT('Ctrl Pts',(-60.4291071651479,72.9548101017499,
62.9646837622432));
#215972=CARTESIAN_POINT('Ctrl Pts',(-60.3973406433091,73.6375194682958,
63.6787631400394));
#215973=CARTESIAN_POINT('Ctrl Pts',(-60.3796177587049,73.9887549030509,
64.122226045083));
#215974=CARTESIAN_POINT('Ctrl Pts',(-60.3401194862685,74.6672830748177,
65.1651930946685));
#215975=CARTESIAN_POINT('Ctrl Pts',(-60.3182272479531,74.9728948688753,
65.7747773161216));
#215976=CARTESIAN_POINT('Ctrl Pts',(-60.2784671051933,75.401781746051,66.9400457991524));
#215977=CARTESIAN_POINT('Ctrl Pts',(-60.2609020586654,75.5465592047606,
67.4842568298563));
#215978=CARTESIAN_POINT('Ctrl Pts',(-60.2222460400084,75.7499098948984,
68.6880320557067));
#215979=CARTESIAN_POINT('Ctrl Pts',(-60.2010841832317,75.7886956464272,
69.3477287843693));
#215980=CARTESIAN_POINT('Ctrl Pts',(-60.1621997556977,75.7279122212125,
70.5650223770047));
#215981=CARTESIAN_POINT('Ctrl Pts',(-60.1447616738229,75.6483764654476,
71.1204788855499));
#215982=CARTESIAN_POINT('Ctrl Pts',(-60.1091224528921,75.3858741071912,
72.2190296645011));
#215983=CARTESIAN_POINT('Ctrl Pts',(-60.0909494791804,75.2017370326686,
72.7593112313773));
#215984=CARTESIAN_POINT('Ctrl Pts',(-60.0546575342054,74.7353549782504,
73.7970219676803));
#215985=CARTESIAN_POINT('Ctrl Pts',(-60.0369333867693,74.4543718763219,
74.2922735798259));
#215986=CARTESIAN_POINT('Ctrl Pts',(-60.0008984767205,73.7968468880922,
75.2335348482422));
#215987=CARTESIAN_POINT('Ctrl Pts',(-59.982524972817,73.4199477940229,75.6761361533574));
#215988=CARTESIAN_POINT('Ctrl Pts',(-59.9262689039094,72.1513027115486,
76.9057234160608));
#215989=CARTESIAN_POINT('Ctrl Pts',(-59.8899075616287,71.1455924541413,
77.5568329908592));
#215990=CARTESIAN_POINT('Ctrl Pts',(-59.8225564684792,69.1771385069917,
78.3415598177888));
#215991=CARTESIAN_POINT('Ctrl Pts',(-59.7938698603394,68.2630575438678,
78.551529702784));
#215992=CARTESIAN_POINT('Ctrl Pts',(-59.7478083985132,66.8067769738529,
78.6569038840467));
#215993=CARTESIAN_POINT('Ctrl Pts',(-59.7309666231927,66.2781321343834,
78.6490832631358));
#215994=CARTESIAN_POINT('Ctrl Pts',(-59.7050207793426,65.4596078240484,
78.5654550958333));
#215995=CARTESIAN_POINT('Ctrl Pts',(-59.6958263910263,65.1676876787616,
78.5211865101182));
#215996=CARTESIAN_POINT('Ctrl Pts',(-59.6682566110299,64.3016287448672,
78.3463637163783));
#215997=CARTESIAN_POINT('Ctrl Pts',(-59.6498248026862,63.7374927199421,
78.174195837292));
#215998=CARTESIAN_POINT('Ctrl Pts',(-59.6218885118325,62.9247555053169,
77.8370397192005));
#215999=CARTESIAN_POINT('Ctrl Pts',(-59.6126077341618,62.6610669258908,
77.7124747335175));
#216000=CARTESIAN_POINT('Ctrl Pts',(-59.5819615934409,61.8062678371396,
77.2571863633938));
#216001=CARTESIAN_POINT('Ctrl Pts',(-59.5610950063817,61.2461417411016,
76.873152214441));
#216002=CARTESIAN_POINT('Ctrl Pts',(-59.5125333127205,60.081336540321,75.8666618148354));
#216003=CARTESIAN_POINT('Ctrl Pts',(-59.4850150054097,59.5123514979381,
75.2128184311312));
#216004=CARTESIAN_POINT('Ctrl Pts',(-59.4204115384272,58.3923723042013,
73.4809525463652));
#216005=CARTESIAN_POINT('Ctrl Pts',(-59.3821095492668,57.9466601155748,
72.3541034375975));
#216006=CARTESIAN_POINT('Ctrl Pts',(-59.3068948782278,57.5199243416264,
69.9991888063659));
#216007=CARTESIAN_POINT('Ctrl Pts',(-59.2686839989018,57.5404091526254,
68.7946198347029));
#216008=CARTESIAN_POINT('Ctrl Pts',(-59.2139668682485,57.9075501483386,
67.0993459426679));
#216009=CARTESIAN_POINT('Ctrl Pts',(-59.1969006211707,58.0691564265514,
66.581616980467));
#216010=CARTESIAN_POINT('Ctrl Pts',(-59.1795703768786,58.2758162902684,
66.0814193421557));
#216011=CARTESIAN_POINT('Origin',(-61.5936228798467,66.6770802411476,69.5524554490054));
#216012=CARTESIAN_POINT('',(-57.1603612091034,58.2758162839768,66.0814193573839));
#216013=CARTESIAN_POINT('',(-57.3654750273695,58.2758162995835,66.0814193196097));
#216014=CARTESIAN_POINT('',(-61.5936228798467,58.2758162839768,66.0814193573839));
#216015=CARTESIAN_POINT('Ctrl Pts',(-57.1603612091034,58.2758162839768,
66.0814193573839));
#216016=CARTESIAN_POINT('Ctrl Pts',(-57.1712661222024,58.1452475191716,
66.3974467995468));
#216017=CARTESIAN_POINT('Ctrl Pts',(-57.1822082696841,58.0325603578707,
66.7207210309766));
#216018=CARTESIAN_POINT('Ctrl Pts',(-57.2022902639678,57.8577543618638,
67.3310862654529));
#216019=CARTESIAN_POINT('Ctrl Pts',(-57.2114561398119,57.7908072758794,
67.6161847140629));
#216020=CARTESIAN_POINT('Ctrl Pts',(-57.2488139815612,57.5751044910439,
68.7859228785457));
#216021=CARTESIAN_POINT('Ctrl Pts',(-57.2775002790807,57.5438792129275,
69.6870618058065));
#216022=CARTESIAN_POINT('Ctrl Pts',(-57.3153519316008,57.6781633218177,
70.8696153349638));
#216023=CARTESIAN_POINT('Ctrl Pts',(-57.3245791482665,57.7253640432311,
71.1593761419318));
#216024=CARTESIAN_POINT('Ctrl Pts',(-57.3713979897335,58.0349246889547,
72.6125612709308));
#216025=CARTESIAN_POINT('Ctrl Pts',(-57.4096981557563,58.5104086352701,
73.7185760902699));
#216026=CARTESIAN_POINT('Ctrl Pts',(-57.4848700000108,59.8571791108076,
75.6780789692153));
#216027=CARTESIAN_POINT('Ctrl Pts',(-57.5230595210081,60.7131947610366,
76.5142356270351));
#216028=CARTESIAN_POINT('Ctrl Pts',(-57.5796441116146,62.2072545352926,
77.4902858809949));
#216029=CARTESIAN_POINT('Ctrl Pts',(-57.5986519251277,62.740165289574,77.7676356633207));
#216030=CARTESIAN_POINT('Ctrl Pts',(-57.6368452303225,63.8403216663152,
78.2083996142362));
#216031=CARTESIAN_POINT('Ctrl Pts',(-57.655766277681,64.4039667314164,78.3732002473953));
#216032=CARTESIAN_POINT('Ctrl Pts',(-57.6897387779918,65.4543830364979,
78.5728746111333));
#216033=CARTESIAN_POINT('Ctrl Pts',(-57.7050478799915,65.9356663071116,
78.6251205984618));
#216034=CARTESIAN_POINT('Ctrl Pts',(-57.7370708345046,66.9327473194481,
78.6534610644127));
#216035=CARTESIAN_POINT('Ctrl Pts',(-57.7537613267708,67.4469907610752,
78.6244398746684));
#216036=CARTESIAN_POINT('Ctrl Pts',(-57.7871348189707,68.4754525927143,
78.4782860108434));
#216037=CARTESIAN_POINT('Ctrl Pts',(-57.8036443426759,68.9875269111625,
78.3596362446721));
#216038=CARTESIAN_POINT('Ctrl Pts',(-57.8298588862109,69.7692601472806,
78.1055921361851));
#216039=CARTESIAN_POINT('Ctrl Pts',(-57.8393871631765,70.0473385829312,
77.9998858624186));
#216040=CARTESIAN_POINT('Ctrl Pts',(-57.8678503423865,70.8566869358599,
77.6458904277372));
#216041=CARTESIAN_POINT('Ctrl Pts',(-57.8868175490356,71.3696771208958,
77.3596542156613));
#216042=CARTESIAN_POINT('Ctrl Pts',(-57.9238936972256,72.3291526637955,
76.6953454487992));
#216043=CARTESIAN_POINT('Ctrl Pts',(-57.9422489360509,72.7739700497115,
76.3196359653321));
#216044=CARTESIAN_POINT('Ctrl Pts',(-57.9770719450073,73.5315159120539,
75.5440567629026));
#216045=CARTESIAN_POINT('Ctrl Pts',(-57.9933836481066,73.8526463595235,
75.1554750045786));
#216046=CARTESIAN_POINT('Ctrl Pts',(-58.0187848528206,74.3072610344771,
74.5017513189591));
#216047=CARTESIAN_POINT('Ctrl Pts',(-58.028037645517,74.4628283109775,74.253233815517));
#216048=CARTESIAN_POINT('Ctrl Pts',(-58.0701920469263,75.1141070978494,
73.0915228206117));
#216049=CARTESIAN_POINT('Ctrl Pts',(-58.1037242784327,75.4630308272156,
72.1050031088081));
#216050=CARTESIAN_POINT('Ctrl Pts',(-58.1524676847489,75.7222762122848,
70.5852533494513));
#216051=CARTESIAN_POINT('Ctrl Pts',(-58.1682524561354,75.7655562463051,
70.0833465289902));
#216052=CARTESIAN_POINT('Ctrl Pts',(-58.2047836169146,75.7690907655136,
68.935399037384));
#216053=CARTESIAN_POINT('Ctrl Pts',(-58.2255939759217,75.7024113135775,
68.2919709574742));
#216054=CARTESIAN_POINT('Ctrl Pts',(-58.2552154228212,75.5073742760806,
67.3751486446046));
#216055=CARTESIAN_POINT('Ctrl Pts',(-58.2643773180735,75.4328036095068,
67.092360514292));
#216056=CARTESIAN_POINT('Ctrl Pts',(-58.3045017033824,75.0484451482113,
65.8759556777904));
#216057=CARTESIAN_POINT('Ctrl Pts',(-58.336068754348,74.6019405620201,64.9925218483251));
#216058=CARTESIAN_POINT('Ctrl Pts',(-58.3822526367361,73.7358253968244,
63.8043649141929));
#216059=CARTESIAN_POINT('Ctrl Pts',(-58.3974266595016,73.4178414285652,
63.4345663647324));
#216060=CARTESIAN_POINT('Ctrl Pts',(-58.4279556190062,72.7308328995985,
62.7545488554096));
#216061=CARTESIAN_POINT('Ctrl Pts',(-58.4432567326164,72.3637128552019,
62.4445964553867));
#216062=CARTESIAN_POINT('Ctrl Pts',(-58.4764805164098,71.5137406186533,
61.8351638570873));
#216063=CARTESIAN_POINT('Ctrl Pts',(-58.4940433119074,71.0238101118098,
61.5489677739113));
#216064=CARTESIAN_POINT('Ctrl Pts',(-58.539322767445,69.7133632638821,60.9394952450883));
#216065=CARTESIAN_POINT('Ctrl Pts',(-58.5674459569514,68.8667077798379,
60.686361062059));
#216066=CARTESIAN_POINT('Ctrl Pts',(-58.6096268545979,67.5336098069249,
60.4907231393167));
#216067=CARTESIAN_POINT('Ctrl Pts',(-58.6241568416528,67.0657078671985,
60.4586331073629));
#216068=CARTESIAN_POINT('Ctrl Pts',(-58.6613914551525,65.8811233892635,
60.4690142903216));
#216069=CARTESIAN_POINT('Ctrl Pts',(-58.6843080721214,65.1680742831271,
60.5599388880564));
#216070=CARTESIAN_POINT('Ctrl Pts',(-58.7254861003152,63.8936855332633,
60.878427776453));
#216071=CARTESIAN_POINT('Ctrl Pts',(-58.743973657381,63.3299318828987,61.0799916400413));
#216072=CARTESIAN_POINT('Ctrl Pts',(-58.7812950465515,62.2609946026372,
61.5856475973009));
#216073=CARTESIAN_POINT('Ctrl Pts',(-58.8000170831936,61.7573601925702,
61.8864137427804));
#216074=CARTESIAN_POINT('Ctrl Pts',(-58.8333116900395,60.9048892011469,
62.5143197920547));
#216075=CARTESIAN_POINT('Ctrl Pts',(-58.8479994067537,60.546159044615,62.8245024333472));
#216076=CARTESIAN_POINT('Ctrl Pts',(-58.8806737948661,59.815039009383,63.563928902679));
#216077=CARTESIAN_POINT('Ctrl Pts',(-58.8987004399109,59.4553575779274,
64.0029717438398));
#216078=CARTESIAN_POINT('Ctrl Pts',(-58.934685010945,58.8232541514026,64.9409774547609));
#216079=CARTESIAN_POINT('Ctrl Pts',(-58.9522657383296,58.5519691498512,
65.4377396990574));
#216080=CARTESIAN_POINT('Ctrl Pts',(-58.9714304678815,58.3106519828565,
65.9979863624172));
#216081=CARTESIAN_POINT('Ctrl Pts',(-58.9728517828832,58.2930770112353,
66.0396416509611));
#216082=CARTESIAN_POINT('Ctrl Pts',(-58.9742739875024,58.2758162752982,
66.0814193783896));
#216083=CARTESIAN_POINT('Ctrl Pts',(-59.1795703768786,58.2758162902684,
66.0814193421557));
#216084=CARTESIAN_POINT('Ctrl Pts',(-59.1783554619545,58.2903039194333,
66.0463536174298));
#216085=CARTESIAN_POINT('Ctrl Pts',(-59.1771395900977,58.3050129701034,
66.0113740408932));
#216086=CARTESIAN_POINT('Ctrl Pts',(-59.1580023294326,58.5398278942509,
65.4626057038298));
#216087=CARTESIAN_POINT('Ctrl Pts',(-59.1399707993854,58.8066445512896,
64.9700978274778));
#216088=CARTESIAN_POINT('Ctrl Pts',(-59.1045782801853,59.4265937330867,
64.0414972473066));
#216089=CARTESIAN_POINT('Ctrl Pts',(-59.0870175121321,59.7781931064481,
63.6072414840463));
#216090=CARTESIAN_POINT('Ctrl Pts',(-59.0544426846447,60.4877515876011,
62.8792057532509));
#216091=CARTESIAN_POINT('Ctrl Pts',(-59.0395901828067,60.8325871584719,
62.575210473491));
#216092=CARTESIAN_POINT('Ctrl Pts',(-59.0012790595759,61.7841913576702,
61.856553700059));
#216093=CARTESIAN_POINT('Ctrl Pts',(-58.9783540265279,62.4208275422783,
61.4869994547136));
#216094=CARTESIAN_POINT('Ctrl Pts',(-58.9400811224291,63.5174394878648,
61.016804275142));
#216095=CARTESIAN_POINT('Ctrl Pts',(-58.9251903171076,63.953093187273,60.8679542643804));
#216096=CARTESIAN_POINT('Ctrl Pts',(-58.8909811787837,64.9811578734939,
60.6017069430898));
#216097=CARTESIAN_POINT('Ctrl Pts',(-58.8720516156921,65.577749454958,60.5090310517618));
#216098=CARTESIAN_POINT('Ctrl Pts',(-58.8212592288542,67.166698702915,60.4218549865817));
#216099=CARTESIAN_POINT('Ctrl Pts',(-58.7892241126204,68.1565398106472,
60.529219092223));
#216100=CARTESIAN_POINT('Ctrl Pts',(-58.7201571117459,70.2523067611285,
61.1112638136952));
#216101=CARTESIAN_POINT('Ctrl Pts',(-58.681850112035,71.32198831223,61.6492411305714));
#216102=CARTESIAN_POINT('Ctrl Pts',(-58.6258058726589,72.7171825145136,
62.7344864657189));
#216103=CARTESIAN_POINT('Ctrl Pts',(-58.6073477142965,73.1408941228739,
63.1347737130986));
#216104=CARTESIAN_POINT('Ctrl Pts',(-58.5703125342873,73.8980738912673,
64.0016995709332));
#216105=CARTESIAN_POINT('Ctrl Pts',(-58.5519771880011,74.2315657457138,
64.4648818344744));
#216106=CARTESIAN_POINT('Ctrl Pts',(-58.5158348585072,74.8089160117557,
65.4499994977671));
#216107=CARTESIAN_POINT('Ctrl Pts',(-58.4977904556718,75.0510264461407,
65.9700094761895));
#216108=CARTESIAN_POINT('Ctrl Pts',(-58.4613656205717,75.4318737860649,
67.0419846493673));
#216109=CARTESIAN_POINT('Ctrl Pts',(-58.443127277265,75.5710199766267,67.5911489293482));
#216110=CARTESIAN_POINT('Ctrl Pts',(-58.401200214888,75.775568699142,68.9007522046425));
#216111=CARTESIAN_POINT('Ctrl Pts',(-58.3773978757872,75.7982019020291,
69.6635873513281));
#216112=CARTESIAN_POINT('Ctrl Pts',(-58.3437328865942,75.6977249455514,
70.7112048530297));
#216113=CARTESIAN_POINT('Ctrl Pts',(-58.3343624876357,75.6558120920739,
71.0005941924054));
#216114=CARTESIAN_POINT('Ctrl Pts',(-58.3048335829351,75.4788394292506,
71.9107461828793));
#216115=CARTESIAN_POINT('Ctrl Pts',(-58.2851404281767,75.2926736038043,
72.5196181081777));
#216116=CARTESIAN_POINT('Ctrl Pts',(-58.2491126807415,74.8472787644228,
73.5689448890223));
#216117=CARTESIAN_POINT('Ctrl Pts',(-58.2329863022464,74.6115832198505,
74.01653283224));
#216118=CARTESIAN_POINT('Ctrl Pts',(-58.1978145991745,74.0174894617805,
74.9475511251046));
#216119=CARTESIAN_POINT('Ctrl Pts',(-58.1791932012746,73.6458381627093,
75.419744531366));
#216120=CARTESIAN_POINT('Ctrl Pts',(-58.1416916477773,72.8180576880623,
76.2808866161529));
#216121=CARTESIAN_POINT('Ctrl Pts',(-58.1227926241545,72.364574562876,76.6683380391131));
#216122=CARTESIAN_POINT('Ctrl Pts',(-58.085241683661,71.395467668143,77.3441215888984));
#216123=CARTESIAN_POINT('Ctrl Pts',(-58.0670255559941,70.8831010247478,
77.6322224346307));
#216124=CARTESIAN_POINT('Ctrl Pts',(-58.039360530937,70.07443944786,77.9890273496044));
#216125=CARTESIAN_POINT('Ctrl Pts',(-58.0300144317083,69.7965888814801,
78.0956667373039));
#216126=CARTESIAN_POINT('Ctrl Pts',(-58.0042966191099,69.0239109083977,
78.3494909837965));
#216127=CARTESIAN_POINT('Ctrl Pts',(-57.9878171919291,68.5209926492301,
78.4684767935116));
#216128=CARTESIAN_POINT('Ctrl Pts',(-57.9554716500303,67.5034843834249,
78.6193907481706));
#216129=CARTESIAN_POINT('Ctrl Pts',(-57.9396109832204,66.9908056785546,
78.6515675826335));
#216130=CARTESIAN_POINT('Ctrl Pts',(-57.9079361110378,65.9817938881639,
78.6294811702175));
#216131=CARTESIAN_POINT('Ctrl Pts',(-57.8921897251693,65.4871604701479,
78.5779694030605));
#216132=CARTESIAN_POINT('Ctrl Pts',(-57.8578333563049,64.4236249111287,
78.3782280819368));
#216133=CARTESIAN_POINT('Ctrl Pts',(-57.8396197007314,63.8598222823445,
78.2147522744286));
#216134=CARTESIAN_POINT('Ctrl Pts',(-57.8025602807082,62.7587331594926,
77.7765177574505));
#216135=CARTESIAN_POINT('Ctrl Pts',(-57.783615510512,62.2250870609842,77.5003096720798));
#216136=CARTESIAN_POINT('Ctrl Pts',(-57.7268277078365,60.72787190169,76.5269614998672));
#216137=CARTESIAN_POINT('Ctrl Pts',(-57.6904418637172,59.8693583329943,
75.6918143451122));
#216138=CARTESIAN_POINT('Ctrl Pts',(-57.6146038668323,58.5181702844445,
73.7338174485842));
#216139=CARTESIAN_POINT('Ctrl Pts',(-57.5779208905498,58.0405516256518,
72.6284875540146));
#216140=CARTESIAN_POINT('Ctrl Pts',(-57.5304110418408,57.7283444453723,
71.175855912788));
#216141=CARTESIAN_POINT('Ctrl Pts',(-57.5210235783432,57.6806385854151,
70.8863747100672));
#216142=CARTESIAN_POINT('Ctrl Pts',(-57.495566040701,57.5885386883781,70.088717004058));
#216143=CARTESIAN_POINT('Ctrl Pts',(-57.4796645880626,57.5727680432773,
69.5783168669611));
#216144=CARTESIAN_POINT('Ctrl Pts',(-57.4445551732079,57.6317087077653,
68.4709984834795));
#216145=CARTESIAN_POINT('Ctrl Pts',(-57.4253083431831,57.7226285145801,
67.8773212063199));
#216146=CARTESIAN_POINT('Ctrl Pts',(-57.3924371001932,57.9774322139581,
66.8825423187258));
#216147=CARTESIAN_POINT('Ctrl Pts',(-57.3789776946765,58.1126384309615,
66.476373532874));
#216148=CARTESIAN_POINT('Ctrl Pts',(-57.3654750286597,58.2758162995991,
66.081419319572));
#216149=CARTESIAN_POINT('Origin',(-64.4265543961493,66.6762871555627,69.5530424137804));
#216150=CARTESIAN_POINT('',(-64.4174334691588,58.2772202579669,66.0829140514164));
#216151=CARTESIAN_POINT('',(-64.5675364832717,58.2772202579675,66.082914051415));
#216152=CARTESIAN_POINT('',(-64.4265543961493,58.2772202579675,66.082914051415));
#216153=CARTESIAN_POINT('',(-64.4174351716144,58.277199894009,66.0829633405634));
#216154=CARTESIAN_POINT('Ctrl Pts',(-64.4174351716144,58.277199894009,66.0829633405634));
#216155=CARTESIAN_POINT('Ctrl Pts',(-64.4174346041292,58.2772066819469,
66.0829469108273));
#216156=CARTESIAN_POINT('Ctrl Pts',(-64.417434036644,58.2772134699327,66.0829304811121));
#216157=CARTESIAN_POINT('Ctrl Pts',(-64.4174334691588,58.2772202579663,
66.0829140514177));
#216158=CARTESIAN_POINT('',(-64.5666618780602,57.6592844329271,70.6707464084894));
#216159=CARTESIAN_POINT('Ctrl Pts',(-64.5657843992066,57.6576119963886,
70.6709037535128));
#216160=CARTESIAN_POINT('Ctrl Pts',(-64.5410292719686,57.5614849398986,
69.8953704510566));
#216161=CARTESIAN_POINT('Ctrl Pts',(-64.5157599548511,57.5657910825955,
69.1106652615182));
#216162=CARTESIAN_POINT('Ctrl Pts',(-64.4664991797538,57.7750153078076,
67.5621750354682));
#216163=CARTESIAN_POINT('Ctrl Pts',(-64.4423690638959,57.978954721852,66.8048452266616));
#216164=CARTESIAN_POINT('Ctrl Pts',(-64.4174351716144,58.277199894009,66.0829633405634));
#216165=CARTESIAN_POINT('Origin',(-64.5675364832709,66.6762871555627,69.5530424137804));
#216166=CARTESIAN_POINT('Origin',(-27.5423496375577,75.0034579025039,72.9903965241317));
#216167=CARTESIAN_POINT('',(-30.7042591052867,64.0608503561673,68.4693880411344));
#216168=CARTESIAN_POINT('',(-31.000413750398,64.0608503608518,68.4693880297961));
#216169=CARTESIAN_POINT('',(-27.5423496375574,64.0608503608518,68.4693880297962));
#216170=CARTESIAN_POINT('',(-32.4074704173708,66.4978162345236,64.7498540653719));
#216171=CARTESIAN_POINT('Ctrl Pts',(-30.7042591049894,64.0608503561645,
68.469388041141));
#216172=CARTESIAN_POINT('Ctrl Pts',(-30.7071426846446,64.0154427292201,
68.5792922457301));
#216173=CARTESIAN_POINT('Ctrl Pts',(-30.7100288359184,63.9716878124109,
68.6898879365682));
#216174=CARTESIAN_POINT('Ctrl Pts',(-30.7314888541783,63.6592255927563,
69.515848345412));
#216175=CARTESIAN_POINT('Ctrl Pts',(-30.7502936496543,63.4586766831916,
70.2550526413332));
#216176=CARTESIAN_POINT('Ctrl Pts',(-30.7880156107471,63.1998218385888,
71.7795464886297));
#216177=CARTESIAN_POINT('Ctrl Pts',(-30.8067238829455,63.1456222748352,
72.5617688967935));
#216178=CARTESIAN_POINT('Ctrl Pts',(-30.8440085560865,63.1912631012398,
74.0910038605536));
#216179=CARTESIAN_POINT('Ctrl Pts',(-30.8623806888472,63.2843220029158,
74.8346162191063));
#216180=CARTESIAN_POINT('Ctrl Pts',(-30.8896020570695,63.5293171722439,
75.9345472556964));
#216181=CARTESIAN_POINT('Ctrl Pts',(-30.8987252784131,63.6294757519157,
76.3004507737405));
#216182=CARTESIAN_POINT('Ctrl Pts',(-30.9264298438691,63.9844125068962,
77.3889408620437));
#216183=CARTESIAN_POINT('Ctrl Pts',(-30.9451999321401,64.2918757388179,
78.0922147103967));
#216184=CARTESIAN_POINT('Ctrl Pts',(-30.9827948279128,65.0460302084666,
79.443360642876));
#216185=CARTESIAN_POINT('Ctrl Pts',(-31.0014216297201,65.4936272557938,
80.0864685814755));
#216186=CARTESIAN_POINT('Ctrl Pts',(-31.0385692917722,66.486983830867,81.2492650194911));
#216187=CARTESIAN_POINT('Ctrl Pts',(-31.0568829521047,67.0254098981056,
81.7704875767997));
#216188=CARTESIAN_POINT('Ctrl Pts',(-31.0840384210422,67.9058691419586,
82.4745158470988));
#216189=CARTESIAN_POINT('Ctrl Pts',(-31.093149591856,68.2135849339152,82.6971936583157));
#216190=CARTESIAN_POINT('Ctrl Pts',(-31.1208186669922,69.1732907502562,
83.3236831828682));
#216191=CARTESIAN_POINT('Ctrl Pts',(-31.1395718503685,69.8542827350363,
83.6793461590018));
#216192=CARTESIAN_POINT('Ctrl Pts',(-31.1771126375038,71.2892595856262,
84.2596240411037));
#216193=CARTESIAN_POINT('Ctrl Pts',(-31.1957134738935,72.0408913952483,
84.4801294607387));
#216194=CARTESIAN_POINT('Ctrl Pts',(-31.2328261856976,73.5432717103284,
84.7635335690407));
#216195=CARTESIAN_POINT('Ctrl Pts',(-31.2511267530039,74.2892704947723,
84.8322225911223));
#216196=CARTESIAN_POINT('Ctrl Pts',(-31.27829085742,75.4168647224421,84.8290518722946));
#216197=CARTESIAN_POINT('Ctrl Pts',(-31.2874176137634,75.7967068024047,
84.8096783011218));
#216198=CARTESIAN_POINT('Ctrl Pts',(-31.3151011656557,76.9370322232514,
84.6962911240781));
#216199=CARTESIAN_POINT('Ctrl Pts',(-31.3338592597317,77.6899539265179,
84.5467542393678));
#216200=CARTESIAN_POINT('Ctrl Pts',(-31.3714446839604,79.1716677353104,
84.099739215657));
#216201=CARTESIAN_POINT('Ctrl Pts',(-31.3900924872514,79.8959898635215,
83.8003273456125));
#216202=CARTESIAN_POINT('Ctrl Pts',(-31.4272898551173,81.2442366145827,
83.079540342749));
#216203=CARTESIAN_POINT('Ctrl Pts',(-31.4456237094184,81.8681769529739,
82.6658180832174));
#216204=CARTESIAN_POINT('Ctrl Pts',(-31.4728620679002,82.7447383616365,
81.9568596407687));
#216205=CARTESIAN_POINT('Ctrl Pts',(-31.4820247386137,83.0288090084183,
81.703525893715));
#216206=CARTESIAN_POINT('Ctrl Pts',(-31.5097611848295,83.8451716263661,
80.9016443138406));
#216207=CARTESIAN_POINT('Ctrl Pts',(-31.5285389512676,84.3370626439491,
80.3148454401391));
#216208=CARTESIAN_POINT('Ctrl Pts',(-31.5691345184249,85.2786526219638,
78.9412856508615));
#216209=CARTESIAN_POINT('Ctrl Pts',(-31.5907117268863,85.7017499304334,
78.1420236914736));
#216210=CARTESIAN_POINT('Ctrl Pts',(-31.6221043829196,86.1683425611218,
76.9488947412377));
#216211=CARTESIAN_POINT('Ctrl Pts',(-31.6314474138179,86.2895437986178,
76.588815954066));
#216212=CARTESIAN_POINT('Ctrl Pts',(-31.6560186422131,86.5635709402545,
75.6234676084616));
#216213=CARTESIAN_POINT('Ctrl Pts',(-31.6710282838724,86.6862204675412,
75.0108756967406));
#216214=CARTESIAN_POINT('Ctrl Pts',(-31.7047675321177,86.8502176585972,
73.6347652353876));
#216215=CARTESIAN_POINT('Ctrl Pts',(-31.7235797176853,86.8671287452743,
72.8711147785176));
#216216=CARTESIAN_POINT('Ctrl Pts',(-31.7649925390056,86.7415693506148,
71.1850076867866));
#216217=CARTESIAN_POINT('Ctrl Pts',(-31.7873184587275,86.5638698267206,
70.2701811467465));
#216218=CARTESIAN_POINT('Ctrl Pts',(-31.8195363190033,86.1654160742036,
69.0236293135017));
#216219=CARTESIAN_POINT('Ctrl Pts',(-31.8289255265732,86.0323725551848,
68.6674815589585));
#216220=CARTESIAN_POINT('Ctrl Pts',(-31.864605379975,85.4592745234184,67.3330086651307));
#216221=CARTESIAN_POINT('Ctrl Pts',(-31.8904165834867,84.904201553612,66.4097114912461));
#216222=CARTESIAN_POINT('Ctrl Pts',(-31.9263510455404,83.9925590087104,
65.2752873839397));
#216223=CARTESIAN_POINT('Ctrl Pts',(-31.9358141557968,83.7383140241215,
64.9885755380937));
#216224=CARTESIAN_POINT('Ctrl Pts',(-31.9582133427393,83.0984926032058,
64.333952009465));
#216225=CARTESIAN_POINT('Ctrl Pts',(-31.9711202053359,82.7011068458162,
63.9787473451167));
#216226=CARTESIAN_POINT('Ctrl Pts',(-32.0026750237428,81.6849222116455,
63.1868450686939));
#216227=CARTESIAN_POINT('Ctrl Pts',(-32.0214467219376,81.0455491664941,
62.7803666280733));
#216228=CARTESIAN_POINT('Ctrl Pts',(-32.0580526551226,79.7158129680039,
62.1039103319514));
#216229=CARTESIAN_POINT('Ctrl Pts',(-32.075846193602,79.0301274923185,61.8320897087201));
#216230=CARTESIAN_POINT('Ctrl Pts',(-32.1123249726576,77.6067419305098,
61.4162476024319));
#216231=CARTESIAN_POINT('Ctrl Pts',(-32.1308571115243,76.8716126199349,
61.2751065960188));
#216232=CARTESIAN_POINT('Ctrl Pts',(-32.1583469877466,75.7504384481428,
61.1681240910288));
#216233=CARTESIAN_POINT('Ctrl Pts',(-32.1675726846286,75.371262005641,61.150260309778));
#216234=CARTESIAN_POINT('Ctrl Pts',(-32.1954647981057,74.2308178101296,
61.1513751461698));
#216235=CARTESIAN_POINT('Ctrl Pts',(-32.2143190124741,73.4715995168137,
61.2254997029869));
#216236=CARTESIAN_POINT('Ctrl Pts',(-32.2522664768761,71.9560477104346,
61.5227405919284));
#216237=CARTESIAN_POINT('Ctrl Pts',(-32.2711443340109,71.2041837518262,
61.7494284969278));
#216238=CARTESIAN_POINT('Ctrl Pts',(-32.309981978744,69.7424751132151,62.3536892187749));
#216239=CARTESIAN_POINT('Ctrl Pts',(-32.3297211176139,69.0374464536894,
62.7325117135954));
#216240=CARTESIAN_POINT('Ctrl Pts',(-32.3590866547182,68.036971548557,63.4083530833487));
#216241=CARTESIAN_POINT('Ctrl Pts',(-32.36901237901,67.7101173600655,63.6547298689732));
#216242=CARTESIAN_POINT('Ctrl Pts',(-32.3889871549098,67.0835947800557,
64.1800127839679));
#216243=CARTESIAN_POINT('Ctrl Pts',(-32.3990228511724,66.7843163110995,
64.4585267821791));
#216244=CARTESIAN_POINT('Ctrl Pts',(-32.4090802221679,66.5000364877912,
64.7519499557376));
#216245=CARTESIAN_POINT('',(-32.7070018384414,66.4978162197124,64.7498540510208));
#216246=CARTESIAN_POINT('Origin',(-32.557235790491,62.9783364609362,61.3397527097253));
#216247=CARTESIAN_POINT('Ctrl Pts',(-32.7053886803439,66.4999818003679,
64.7520064024586));
#216248=CARTESIAN_POINT('Ctrl Pts',(-32.69553011162,66.7838357164023,64.4590189430342));
#216249=CARTESIAN_POINT('Ctrl Pts',(-32.6856649273,67.0826424505334,64.1808973524643));
#216250=CARTESIAN_POINT('Ctrl Pts',(-32.6657877293566,67.708153828014,63.6562902858532));
#216251=CARTESIAN_POINT('Ctrl Pts',(-32.6557887964716,68.0344722672034,
63.4101961781974));
#216252=CARTESIAN_POINT('Ctrl Pts',(-32.6262999049639,69.0332045268677,
62.7350772305994));
#216253=CARTESIAN_POINT('Ctrl Pts',(-32.6072197959714,69.7369472826996,
62.3565181907147));
#216254=CARTESIAN_POINT('Ctrl Pts',(-32.5689385580399,71.197168794757,61.7517989533017));
#216255=CARTESIAN_POINT('Ctrl Pts',(-32.5496988886399,71.9489320636044,
61.5246309910955));
#216256=CARTESIAN_POINT('Ctrl Pts',(-32.5123069727106,73.4641355241297,
61.2264875436045));
#216257=CARTESIAN_POINT('Ctrl Pts',(-32.4941342755606,74.223093637015,61.1518955209385));
#216258=CARTESIAN_POINT('Ctrl Pts',(-32.4664075871642,75.3634572583079,
61.1500161322631));
#216259=CARTESIAN_POINT('Ctrl Pts',(-32.4571372927898,75.7427796746091,
61.1676383890037));
#216260=CARTESIAN_POINT('Ctrl Pts',(-32.4296885153319,76.8641116262045,
61.2739156704039));
#216261=CARTESIAN_POINT('Ctrl Pts',(-32.4118711067863,77.5992898795384,
61.4145763117665));
#216262=CARTESIAN_POINT('Ctrl Pts',(-32.3748773209694,79.0689253298945,
61.8428988407649));
#216263=CARTESIAN_POINT('Ctrl Pts',(-32.3556591558999,79.7978996496223,
62.1364547210756));
#216264=CARTESIAN_POINT('Ctrl Pts',(-32.3274982129129,80.8297798259273,
62.676374092178));
#216265=CARTESIAN_POINT('Ctrl Pts',(-32.3183713064889,81.1583600006871,
62.869019777627));
#216266=CARTESIAN_POINT('Ctrl Pts',(-32.2876728591593,82.2258550138294,
63.5661248169695));
#216267=CARTESIAN_POINT('Ctrl Pts',(-32.2658307792389,82.9168109882992,
64.1383494603416));
#216268=CARTESIAN_POINT('Ctrl Pts',(-32.23486475593,83.8015000256364,65.0581515036157));
#216269=CARTESIAN_POINT('Ctrl Pts',(-32.2256966396352,84.0527919668674,
65.3460777205622));
#216270=CARTESIAN_POINT('Ctrl Pts',(-32.1982533126496,84.7599044459102,
66.2401090071176));
#216271=CARTESIAN_POINT('Ctrl Pts',(-32.1798623274365,85.1719124448039,
66.878346835215));
#216272=CARTESIAN_POINT('Ctrl Pts',(-32.1431317556561,85.8630907085791,
68.2148211866102));
#216273=CARTESIAN_POINT('Ctrl Pts',(-32.1252359546489,86.1425911901294,
68.9090417134335));
#216274=CARTESIAN_POINT('Ctrl Pts',(-32.0875611591384,86.5854727520725,
70.4028444675641));
#216275=CARTESIAN_POINT('Ctrl Pts',(-32.0676444524148,86.7355291046516,
71.2023859468808));
#216276=CARTESIAN_POINT('Ctrl Pts',(-32.0294893527047,86.8653955626351,
72.7668782629184));
#216277=CARTESIAN_POINT('Ctrl Pts',(-32.0113448408402,86.8553566833968,
73.5270791544992));
#216278=CARTESIAN_POINT('Ctrl Pts',(-31.979996561774,86.7151982900055,74.8051252905583));
#216279=CARTESIAN_POINT('Ctrl Pts',(-31.9670375712713,86.6227916829676,
75.3247451323471));
#216280=CARTESIAN_POINT('Ctrl Pts',(-31.944840905975,86.4042186066256,76.2073552875076));
#216281=CARTESIAN_POINT('Ctrl Pts',(-31.9356138391446,86.2944722024968,
76.5735745492717));
#216282=CARTESIAN_POINT('Ctrl Pts',(-31.9079019692038,85.9130993046381,
77.6532264364888));
#216283=CARTESIAN_POINT('Ctrl Pts',(-31.8893055272082,85.590048538782,78.3463600610293));
#216284=CARTESIAN_POINT('Ctrl Pts',(-31.8522266233887,84.8233265681204,
79.6468179367242));
#216285=CARTESIAN_POINT('Ctrl Pts',(-31.8341954264111,84.384079288709,80.2527455045997));
#216286=CARTESIAN_POINT('Ctrl Pts',(-31.7954192498862,83.3308394184371,
81.4492901129661));
#216287=CARTESIAN_POINT('Ctrl Pts',(-31.7744777428662,82.7043190559933,
82.0233852119809));
#216288=CARTESIAN_POINT('Ctrl Pts',(-31.7350937174841,81.4068920363101,
82.9783585419448));
#216289=CARTESIAN_POINT('Ctrl Pts',(-31.7166924725776,80.7495141984602,
83.3704831346131));
#216290=CARTESIAN_POINT('Ctrl Pts',(-31.6854021877319,79.5972140386992,
83.9146054460994));
#216291=CARTESIAN_POINT('Ctrl Pts',(-31.6727692925259,79.1218395882889,
84.1025460178052));
#216292=CARTESIAN_POINT('Ctrl Pts',(-31.6508516209878,78.2725307300772,
84.3763103513238));
#216293=CARTESIAN_POINT('Ctrl Pts',(-31.6415771462094,77.903790584014,84.4757759950525));
#216294=CARTESIAN_POINT('Ctrl Pts',(-31.6063238455528,76.4894928033484,
84.7848090554636));
#216295=CARTESIAN_POINT('Ctrl Pts',(-31.5799383618991,75.422119384323,84.8706816344041));
#216296=CARTESIAN_POINT('Ctrl Pts',(-31.5350170505017,73.5891271361704,
84.7705654860981));
#216297=CARTESIAN_POINT('Ctrl Pts',(-31.5163791926102,72.8264335972992,
84.6537271396055));
#216298=CARTESIAN_POINT('Ctrl Pts',(-31.4785596356244,71.3393754622557,
84.274880775917));
#216299=CARTESIAN_POINT('Ctrl Pts',(-31.4596683236531,70.6182861336933,
84.014704384785));
#216300=CARTESIAN_POINT('Ctrl Pts',(-31.4127644084642,68.8806102415118,
83.190068806834));
#216301=CARTESIAN_POINT('Ctrl Pts',(-31.3841098190006,67.9124382865636,
82.5423603132802));
#216302=CARTESIAN_POINT('Ctrl Pts',(-31.346463958581,66.7718729432973,81.5089613897664));
#216303=CARTESIAN_POINT('Ctrl Pts',(-31.3372185118236,66.5023947921537,
81.2400550046652));
#216304=CARTESIAN_POINT('Ctrl Pts',(-31.3097513689028,65.7453175508535,
80.4080248239167));
#216305=CARTESIAN_POINT('Ctrl Pts',(-31.291380037766,65.297350173782,79.8113812998257));
#216306=CARTESIAN_POINT('Ctrl Pts',(-31.2545593074383,64.5168065285002,
78.5376458706384));
#216307=CARTESIAN_POINT('Ctrl Pts',(-31.2364814277601,64.1867836197617,
77.8629103381064));
#216308=CARTESIAN_POINT('Ctrl Pts',(-31.1990043797762,63.6472878523156,
76.4297260793805));
#216309=CARTESIAN_POINT('Ctrl Pts',(-31.1796109502199,63.4449878567384,
75.6724400221149));
#216310=CARTESIAN_POINT('Ctrl Pts',(-31.1512319403437,63.2574028599595,
74.5250858009222));
#216311=CARTESIAN_POINT('Ctrl Pts',(-31.1420080999806,63.2141357960004,
74.1466687520122));
#216312=CARTESIAN_POINT('Ctrl Pts',(-31.1145807159917,63.1402361027004,
73.022198413814));
#216313=CARTESIAN_POINT('Ctrl Pts',(-31.0962361987064,63.1618075858758,
72.2746107871689));
#216314=CARTESIAN_POINT('Ctrl Pts',(-31.0595156189855,63.3456446913962,
70.7914046029045));
#216315=CARTESIAN_POINT('Ctrl Pts',(-31.0415259421293,63.5078929487642,
70.0591575253195));
#216316=CARTESIAN_POINT('Ctrl Pts',(-31.0156884362488,63.8341785308065,
69.0502524767953));
#216317=CARTESIAN_POINT('Ctrl Pts',(-31.0080604239167,63.9418373514177,
68.7574460275236));
#216318=CARTESIAN_POINT('Ctrl Pts',(-31.000413750398,64.0608503608518,68.4693880297961));
#216319=CARTESIAN_POINT('Origin',(-27.5423496375577,75.0034579025039,72.9903965241317));
#216320=CARTESIAN_POINT('',(-28.8902889611216,64.0608503608518,68.4693880297961));
#216321=CARTESIAN_POINT('',(-29.1863798856003,64.0608503608518,68.4693880297961));
#216322=CARTESIAN_POINT('',(-27.5423496375574,64.0608503608518,68.4693880297962));
#216323=CARTESIAN_POINT('Ctrl Pts',(-28.8902889611216,64.0608503608518,
68.4693880297961));
#216324=CARTESIAN_POINT('Ctrl Pts',(-28.8995283196927,63.9171340345322,
68.8172377094005));
#216325=CARTESIAN_POINT('Ctrl Pts',(-28.9087847528996,63.7900030671402,
69.1719427226877));
#216326=CARTESIAN_POINT('Ctrl Pts',(-28.9365166291705,63.4572271982444,
70.2616197964341));
#216327=CARTESIAN_POINT('Ctrl Pts',(-28.9548136304281,63.3054826777762,
71.0107377528076));
#216328=CARTESIAN_POINT('Ctrl Pts',(-28.9826977015882,63.1877012504632,
72.1465920055058));
#216329=CARTESIAN_POINT('Ctrl Pts',(-28.992003005461,63.1667315488403,72.5256171768658));
#216330=CARTESIAN_POINT('Ctrl Pts',(-29.0195714907716,63.1586040887462,
73.6523155198278));
#216331=CARTESIAN_POINT('Ctrl Pts',(-29.0374679866773,63.2239830584802,
74.3984706514494));
#216332=CARTESIAN_POINT('Ctrl Pts',(-29.0745754382403,63.5010448035412,
75.9038613978213));
#216333=CARTESIAN_POINT('Ctrl Pts',(-29.0938293810776,63.7189370449008,
76.6582798779555));
#216334=CARTESIAN_POINT('Ctrl Pts',(-29.1312567613625,64.2921896779695,
78.0921469569484));
#216335=CARTESIAN_POINT('Ctrl Pts',(-29.1494411325762,64.6421002606472,
78.7697908854879));
#216336=CARTESIAN_POINT('Ctrl Pts',(-29.1834627585719,65.4002903058035,
79.9449581265054));
#216337=CARTESIAN_POINT('Ctrl Pts',(-29.1990955258074,65.7886947130422,
80.4519580793481));
#216338=CARTESIAN_POINT('Ctrl Pts',(-29.2236639274506,66.4707109623571,
81.2072584793979));
#216339=CARTESIAN_POINT('Ctrl Pts',(-29.2327815371745,66.7388238095533,
81.4768807592511));
#216340=CARTESIAN_POINT('Ctrl Pts',(-29.2598230607728,67.5669082104724,
82.2331012105019));
#216341=CARTESIAN_POINT('Ctrl Pts',(-29.2778991999651,68.1601308107924,
82.6805319137459));
#216342=CARTESIAN_POINT('Ctrl Pts',(-29.3141450709817,69.4278956972455,
83.4619064130423));
#216343=CARTESIAN_POINT('Ctrl Pts',(-29.3319583200587,70.1002537270503,
83.7930815033909));
#216344=CARTESIAN_POINT('Ctrl Pts',(-29.3672593377321,71.4644647671734,
84.3112586206249));
#216345=CARTESIAN_POINT('Ctrl Pts',(-29.3846907416036,72.1510031810128,
84.5034276001188));
#216346=CARTESIAN_POINT('Ctrl Pts',(-29.4197344481068,73.5737642407376,
84.7665150208697));
#216347=CARTESIAN_POINT('Ctrl Pts',(-29.437267317923,74.3077937902918,84.832569043604));
#216348=CARTESIAN_POINT('Ctrl Pts',(-29.4732775384949,75.7913509524845,
84.8275898529678));
#216349=CARTESIAN_POINT('Ctrl Pts',(-29.491613648245,76.5375895026883,84.7541701288638));
#216350=CARTESIAN_POINT('Ctrl Pts',(-29.5187968222645,77.6440722559224,
84.5381724213967));
#216351=CARTESIAN_POINT('Ctrl Pts',(-29.5279055197581,78.0125445201575,
84.4476811094524));
#216352=CARTESIAN_POINT('Ctrl Pts',(-29.5556043135655,79.1112967674302,
84.1211728795115));
#216353=CARTESIAN_POINT('Ctrl Pts',(-29.5743943826445,79.8235803821709,
83.8317491984357));
#216354=CARTESIAN_POINT('Ctrl Pts',(-29.6166217721661,81.361006721127,83.0253745327922));
#216355=CARTESIAN_POINT('Ctrl Pts',(-29.6397325115422,82.1606716055852,
82.4716152157968));
#216356=CARTESIAN_POINT('Ctrl Pts',(-29.6727251246817,83.1677281029812,
81.5734914110518));
#216357=CARTESIAN_POINT('Ctrl Pts',(-29.6820549745417,83.4392103276158,
81.3068204495254));
#216358=CARTESIAN_POINT('Ctrl Pts',(-29.7135942069433,84.3181727138243,
80.3560312747861));
#216359=CARTESIAN_POINT('Ctrl Pts',(-29.7354604105003,84.8590724017529,
79.6148479509096));
#216360=CARTESIAN_POINT('Ctrl Pts',(-29.7671521272747,85.4962376963539,
78.4882156517042));
#216361=CARTESIAN_POINT('Ctrl Pts',(-29.7764893680399,85.6671975926004,
78.1487972975652));
#216362=CARTESIAN_POINT('Ctrl Pts',(-29.8140375203506,86.2911770042174,
76.7458108067079));
#216363=CARTESIAN_POINT('Ctrl Pts',(-29.8417316022383,86.603683301564,75.6267776870563));
#216364=CARTESIAN_POINT('Ctrl Pts',(-29.889083706918,86.8460191498429,73.7163248453229));
#216365=CARTESIAN_POINT('Ctrl Pts',(-29.9076925494568,86.868159572991,72.944711902705));
#216366=CARTESIAN_POINT('Ctrl Pts',(-29.9450551075506,86.762717067064,71.4145921473615));
#216367=CARTESIAN_POINT('Ctrl Pts',(-29.9639086151304,86.6366337551139,
70.6596153030522));
#216368=CARTESIAN_POINT('Ctrl Pts',(-30.0085206985524,86.1656157605052,
68.9041916152091));
#216369=CARTESIAN_POINT('Ctrl Pts',(-30.0338700129661,85.7578132587307,
67.9273261156758));
#216370=CARTESIAN_POINT('Ctrl Pts',(-30.0693094538078,85.0332503972255,
66.6872515359413));
#216371=CARTESIAN_POINT('Ctrl Pts',(-30.0787573876203,84.8244766729224,
66.3666538540317));
#216372=CARTESIAN_POINT('Ctrl Pts',(-30.1002157099478,84.3110038478021,
65.6559414998619));
#216373=CARTESIAN_POINT('Ctrl Pts',(-30.112200390852,83.9966297791216,65.2736936378709));
#216374=CARTESIAN_POINT('Ctrl Pts',(-30.1428896282947,83.1402829464073,
64.3561117856364));
#216375=CARTESIAN_POINT('Ctrl Pts',(-30.1617389531945,82.5689029361146,
63.8513143523389));
#216376=CARTESIAN_POINT('Ctrl Pts',(-30.1997201187605,81.3183893218145,
62.9446825912728));
#216377=CARTESIAN_POINT('Ctrl Pts',(-30.2186358410031,80.6395783999868,
62.5487071409636));
#216378=CARTESIAN_POINT('Ctrl Pts',(-30.2562907179915,79.2474660775924,
61.9122079365959));
#216379=CARTESIAN_POINT('Ctrl Pts',(-30.2748230233428,78.5404412751904,
61.6666327809114));
#216380=CARTESIAN_POINT('Ctrl Pts',(-30.3023168365406,77.4464782846083,
61.3992032615102));
#216381=CARTESIAN_POINT('Ctrl Pts',(-30.3115448502552,77.0738292245333,
61.3268776539251));
#216382=CARTESIAN_POINT('Ctrl Pts',(-30.3394414902501,75.9452472279289,
61.1636368586258));
#216383=CARTESIAN_POINT('Ctrl Pts',(-30.3582986518662,75.1833974202189,
61.1275629500521));
#216384=CARTESIAN_POINT('Ctrl Pts',(-30.3962644743953,73.6408288637397,
61.2032308449913));
#216385=CARTESIAN_POINT('Ctrl Pts',(-30.4151542734454,72.8640206097579,
61.319199271877));
#216386=CARTESIAN_POINT('Ctrl Pts',(-30.4527642488833,71.379827850808,61.6940280567394));
#216387=CARTESIAN_POINT('Ctrl Pts',(-30.4712801870707,70.6742226457001,
61.9451999629897));
#216388=CARTESIAN_POINT('Ctrl Pts',(-30.4987242331526,69.6534852610907,
62.4214951159395));
#216389=CARTESIAN_POINT('Ctrl Pts',(-30.5079245437531,69.3178539669437,
62.5981979017771));
#216390=CARTESIAN_POINT('Ctrl Pts',(-30.5357803140262,68.3345629208456,
63.1777954724162));
#216391=CARTESIAN_POINT('Ctrl Pts',(-30.5546204634495,67.7167695413567,
63.6274130181923));
#216392=CARTESIAN_POINT('Ctrl Pts',(-30.5924875226138,66.5608460375821,
64.6528080587044));
#216393=CARTESIAN_POINT('Ctrl Pts',(-30.6112979661866,66.0281591470195,
65.2291405841927));
#216394=CARTESIAN_POINT('Ctrl Pts',(-30.6487638962762,65.105627462703,66.4503606319373));
#216395=CARTESIAN_POINT('Ctrl Pts',(-30.6672161329818,64.7125007167355,
67.088250543124));
#216396=CARTESIAN_POINT('Ctrl Pts',(-30.6916656655681,64.2672696883344,
67.9921921862697));
#216397=CARTESIAN_POINT('Ctrl Pts',(-30.6979556134436,64.1601112148153,
68.2291379675095));
#216398=CARTESIAN_POINT('Ctrl Pts',(-30.7042591049894,64.0608503561645,
68.469388041141));
#216399=CARTESIAN_POINT('Ctrl Pts',(-31.000413750398,64.0608503608518,68.4693880297961));
#216400=CARTESIAN_POINT('Ctrl Pts',(-30.9894496917122,64.2314952323248,
68.056360746201));
#216401=CARTESIAN_POINT('Ctrl Pts',(-30.9784421942637,64.4254828637911,
67.6530958066313));
#216402=CARTESIAN_POINT('Ctrl Pts',(-30.9489866486578,65.0109590167339,
66.5941692359763));
#216403=CARTESIAN_POINT('Ctrl Pts',(-30.9306856435903,65.4435799455716,
65.9639821995385));
#216404=CARTESIAN_POINT('Ctrl Pts',(-30.9027964538502,66.1776565319684,
65.0891727800485));
#216405=CARTESIAN_POINT('Ctrl Pts',(-30.8934900614081,66.435349072473,64.8104443940101));
#216406=CARTESIAN_POINT('Ctrl Pts',(-30.8659179066328,67.2390950257741,
64.02081564219));
#216407=CARTESIAN_POINT('Ctrl Pts',(-30.8480189096461,67.8206066990283,
63.5487143437753));
#216408=CARTESIAN_POINT('Ctrl Pts',(-30.8109072024215,69.0947801507967,
62.7005335799142));
#216409=CARTESIAN_POINT('Ctrl Pts',(-30.7916515945159,69.7882978510282,
62.3322610185254));
#216410=CARTESIAN_POINT('Ctrl Pts',(-30.7542197263624,71.2171650947603,
61.7465901632417));
#216411=CARTESIAN_POINT('Ctrl Pts',(-30.7360324769979,71.9474318085476,
61.526544373066));
#216412=CARTESIAN_POINT('Ctrl Pts',(-30.7082843981268,73.0660586956442,
61.304047188608));
#216413=CARTESIAN_POINT('Ctrl Pts',(-30.6990064488469,73.4417148441884,
61.2479421664651));
#216414=CARTESIAN_POINT('Ctrl Pts',(-30.6715352735179,74.5626272885663,
61.1352798461866));
#216415=CARTESIAN_POINT('Ctrl Pts',(-30.6537045524294,75.3112417532731,
61.1310797775953));
#216416=CARTESIAN_POINT('Ctrl Pts',(-30.6166987175427,76.8360320209113,
61.2670725843473));
#216417=CARTESIAN_POINT('Ctrl Pts',(-30.5974786215739,77.6079706799152,
61.4140776267444));
#216418=CARTESIAN_POINT('Ctrl Pts',(-30.5601372717332,79.0885388976018,
61.8517288475339));
#216419=CARTESIAN_POINT('Ctrl Pts',(-30.5420056674958,79.7949462173665,
62.1368509983944));
#216420=CARTESIAN_POINT('Ctrl Pts',(-30.5143121205572,80.8061506797072,
62.663089451141));
#216421=CARTESIAN_POINT('Ctrl Pts',(-30.5050377472477,81.1345263561437,
62.8545929730509));
#216422=CARTESIAN_POINT('Ctrl Pts',(-30.4775977076468,82.0790997762352,
63.4681772621597));
#216423=CARTESIAN_POINT('Ctrl Pts',(-30.4597881954024,82.6652183852194,
63.9330903470363));
#216424=CARTESIAN_POINT('Ctrl Pts',(-30.4227954929986,83.7692646956418,
64.9931677192314));
#216425=CARTESIAN_POINT('Ctrl Pts',(-30.4035642689954,84.2795254235964,
65.5910991644193));
#216426=CARTESIAN_POINT('Ctrl Pts',(-30.3661762013661,85.1607767831556,
66.8595510141587));
#216427=CARTESIAN_POINT('Ctrl Pts',(-30.3480147281005,85.5334673392602,
67.5243832837642));
#216428=CARTESIAN_POINT('Ctrl Pts',(-30.3173044039153,86.041964649879,68.6795630408262));
#216429=CARTESIAN_POINT('Ctrl Pts',(-30.305008169594,86.2147106522098,69.1511613564153));
#216430=CARTESIAN_POINT('Ctrl Pts',(-30.2835062852645,86.4654097595363,
69.9987605462407));
#216431=CARTESIAN_POINT('Ctrl Pts',(-30.2743102972342,86.5559953283855,
70.3702618605894));
#216432=CARTESIAN_POINT('Ctrl Pts',(-30.2467410045947,86.7726957501231,
71.4924223678137));
#216433=CARTESIAN_POINT('Ctrl Pts',(-30.2282552018806,86.8446118847982,
72.251514321688));
#216434=CARTESIAN_POINT('Ctrl Pts',(-30.1913586402202,86.8418313287905,
73.7590405627578));
#216435=CARTESIAN_POINT('Ctrl Pts',(-30.1733966849236,86.7697985538877,
74.5040444843898));
#216436=CARTESIAN_POINT('Ctrl Pts',(-30.1353420039617,86.471887487321,76.0453335157137));
#216437=CARTESIAN_POINT('Ctrl Pts',(-30.1150845933223,86.2318747685675,
76.8348930447516));
#216438=CARTESIAN_POINT('Ctrl Pts',(-30.0857305276675,85.7638798586112,
77.9440350612097));
#216439=CARTESIAN_POINT('Ctrl Pts',(-30.0765347506624,85.5989836952713,
78.287570286964));
#216440=CARTESIAN_POINT('Ctrl Pts',(-30.0428586838187,84.9380281839819,
79.5097345220104));
#216441=CARTESIAN_POINT('Ctrl Pts',(-30.017992731629,84.3468343501822,80.3319735493999));
#216442=CARTESIAN_POINT('Ctrl Pts',(-29.9841355838273,83.399247034245,81.3471537239098));
#216443=CARTESIAN_POINT('Ctrl Pts',(-29.9749379466191,83.1266425298508,
81.6123764884997));
#216444=CARTESIAN_POINT('Ctrl Pts',(-29.9427149566454,82.133242284368,82.4898713784685));
#216445=CARTESIAN_POINT('Ctrl Pts',(-29.9193411863813,81.3523246666702,
83.0286095885796));
#216446=CARTESIAN_POINT('Ctrl Pts',(-29.8774996552059,79.8372895143436,
83.8256098815549));
#216447=CARTESIAN_POINT('Ctrl Pts',(-29.858996784471,79.1258264058366,84.1157666172291));
#216448=CARTESIAN_POINT('Ctrl Pts',(-29.8308165594585,78.0276657130448,
84.4437098691035));
#216449=CARTESIAN_POINT('Ctrl Pts',(-29.821439008496,77.658995259724,84.5347605156796));
#216450=CARTESIAN_POINT('Ctrl Pts',(-29.7936444395498,76.5527280944839,
84.7521691217944));
#216451=CARTESIAN_POINT('Ctrl Pts',(-29.7755815110642,75.8068502324153,
84.8265316423571));
#216452=CARTESIAN_POINT('Ctrl Pts',(-29.7391907940041,74.3205379707526,
84.8334988644688));
#216453=CARTESIAN_POINT('Ctrl Pts',(-29.7208679422368,73.5834173872748,
84.7678719069654));
#216454=CARTESIAN_POINT('Ctrl Pts',(-29.6850838483617,72.1500663534938,
84.5036674362149));
#216455=CARTESIAN_POINT('Ctrl Pts',(-29.6677084140159,71.456244169244,84.3091655361203));
#216456=CARTESIAN_POINT('Ctrl Pts',(-29.6316592996819,70.0858288212269,
83.786508493853));
#216457=CARTESIAN_POINT('Ctrl Pts',(-29.6130886579611,69.414090372518,83.4545299006175));
#216458=CARTESIAN_POINT('Ctrl Pts',(-29.5766865576869,68.1467291337866,
82.6711241672695));
#216459=CARTESIAN_POINT('Ctrl Pts',(-29.5586589112334,67.5534087372805,
82.2222968714626));
#216460=CARTESIAN_POINT('Ctrl Pts',(-29.5309788247731,66.725759117199,81.4641411953882));
#216461=CARTESIAN_POINT('Ctrl Pts',(-29.5215695524604,66.4580119297219,
81.1940541730017));
#216462=CARTESIAN_POINT('Ctrl Pts',(-29.4970774975597,65.792768169438,80.4550248991482));
#216463=CARTESIAN_POINT('Ctrl Pts',(-29.4822163965635,65.4179672352868,
79.9672046448307));
#216464=CARTESIAN_POINT('Ctrl Pts',(-29.4485768052823,64.6666833955792,
78.8138212272529));
#216465=CARTESIAN_POINT('Ctrl Pts',(-29.4297129690732,64.3133079962881,
78.1364498539328));
#216466=CARTESIAN_POINT('Ctrl Pts',(-29.3917545451264,63.733881245762,76.7038891397521));
#216467=CARTESIAN_POINT('Ctrl Pts',(-29.3729028524237,63.5130026749589,
75.9506039498728));
#216468=CARTESIAN_POINT('Ctrl Pts',(-29.335357217513,63.2297676312216,74.4462388096491));
#216469=CARTESIAN_POINT('Ctrl Pts',(-29.3168550496804,63.1613394074936,
73.6999727832052));
#216470=CARTESIAN_POINT('Ctrl Pts',(-29.2805033884888,63.1661536575647,
72.2056509896819));
#216471=CARTESIAN_POINT('Ctrl Pts',(-29.2624303821015,63.2391734706643,
71.4609495912181));
#216472=CARTESIAN_POINT('Ctrl Pts',(-29.2347456172582,63.4545805086691,
70.3543832748118));
#216473=CARTESIAN_POINT('Ctrl Pts',(-29.2253655360921,63.5453134983676,
69.9843922354757));
#216474=CARTESIAN_POINT('Ctrl Pts',(-29.2060769114822,63.7696440352676,
69.2290941472924));
#216475=CARTESIAN_POINT('Ctrl Pts',(-29.1962359460276,63.9055604679698,
68.8452502638799));
#216476=CARTESIAN_POINT('Ctrl Pts',(-29.1863798856003,64.0608503608518,
68.4693880297961));
#216477=CARTESIAN_POINT('Origin',(-27.5423496375577,75.0034579025039,72.9903965241317));
#216478=CARTESIAN_POINT('',(-27.0763524842809,64.0608503697698,68.4693880082113));
#216479=CARTESIAN_POINT('',(-27.372320352868,64.0608503540424,68.4693880462777));
#216480=CARTESIAN_POINT('',(-27.5423496375574,64.0608503608518,68.4693880297962));
#216481=CARTESIAN_POINT('Ctrl Pts',(-27.0763524848464,64.060850369775,68.4693880081986));
#216482=CARTESIAN_POINT('Ctrl Pts',(-27.0859054812614,63.9103020442731,
68.8337737939964));
#216483=CARTESIAN_POINT('Ctrl Pts',(-27.0954454003588,63.7779643153705,
69.2056558759773));
#216484=CARTESIAN_POINT('Ctrl Pts',(-27.1240969798107,63.4392340773519,
70.3330959904916));
#216485=CARTESIAN_POINT('Ctrl Pts',(-27.1433969711315,63.2889256567875,
71.103003032948));
#216486=CARTESIAN_POINT('Ctrl Pts',(-27.1716284560733,63.1800423553295,
72.2610696888224));
#216487=CARTESIAN_POINT('Ctrl Pts',(-27.1807979879519,63.162707149997,72.6415477925153));
#216488=CARTESIAN_POINT('Ctrl Pts',(-27.2080544187198,63.1657330101346,
73.7680523132948));
#216489=CARTESIAN_POINT('Ctrl Pts',(-27.226280950715,63.2382106843945,74.5120488357248));
#216490=CARTESIAN_POINT('Ctrl Pts',(-27.2627659024089,63.5225250141981,
75.9782701625852));
#216491=CARTESIAN_POINT('Ctrl Pts',(-27.280636774545,63.7340658601985,76.6971488914858));
#216492=CARTESIAN_POINT('Ctrl Pts',(-27.3162039900716,64.2797231648403,
78.059966517954));
#216493=CARTESIAN_POINT('Ctrl Pts',(-27.3338728650167,64.6079288137639,
78.7028384096687));
#216494=CARTESIAN_POINT('Ctrl Pts',(-27.3606241720471,65.1964491124216,
79.6348414696851));
#216495=CARTESIAN_POINT('Ctrl Pts',(-27.3697957489021,65.4158936025924,
79.9477438654496));
#216496=CARTESIAN_POINT('Ctrl Pts',(-27.4013118299121,66.2180890267998,
80.9813767335047));
#216497=CARTESIAN_POINT('Ctrl Pts',(-27.4239171150195,66.8700467560069,
81.6440703277155));
#216498=CARTESIAN_POINT('Ctrl Pts',(-27.4556963398358,67.8909836980437,
82.4634808560025));
#216499=CARTESIAN_POINT('Ctrl Pts',(-27.4648823409838,68.2008576031965,
82.688398678786));
#216500=CARTESIAN_POINT('Ctrl Pts',(-27.4994364915695,69.4025724377663,
83.4746672666346));
#216501=CARTESIAN_POINT('Ctrl Pts',(-27.5251904055295,70.3571083794556,
83.9312042596608));
#216502=CARTESIAN_POINT('Ctrl Pts',(-27.5598186225791,71.7211337912766,
84.3724476925238));
#216503=CARTESIAN_POINT('Ctrl Pts',(-27.5689345990207,72.0883185096068,
84.4719775829097));
#216504=CARTESIAN_POINT('Ctrl Pts',(-27.5991497969802,73.3133657456307,
84.7414756611852));
#216505=CARTESIAN_POINT('Ctrl Pts',(-27.6205145015352,74.1852477269069,
84.8341620975593));
#216506=CARTESIAN_POINT('Ctrl Pts',(-27.6600365696807,75.8143749013741,
84.8264712668729));
#216507=CARTESIAN_POINT('Ctrl Pts',(-27.6780294399353,76.5673293365037,
84.7506925613435));
#216508=CARTESIAN_POINT('Ctrl Pts',(-27.7095456087994,77.8403516610893,
84.4980831466947));
#216509=CARTESIAN_POINT('Ctrl Pts',(-27.7228394100444,78.3648806946213,
84.3559432110618));
#216510=CARTESIAN_POINT('Ctrl Pts',(-27.7453559160673,79.2394927715973,
84.0530677832568));
#216511=CARTESIAN_POINT('Ctrl Pts',(-27.7545658539053,79.5948966989033,
83.9103496798472));
#216512=CARTESIAN_POINT('Ctrl Pts',(-27.7821587000339,80.6352530604497,
83.4327931444223));
#216513=CARTESIAN_POINT('Ctrl Pts',(-27.8006470615131,81.2954395316747,
83.0488119057356));
#216514=CARTESIAN_POINT('Ctrl Pts',(-27.8375647517096,82.5210570054952,
82.1677915114698));
#216515=CARTESIAN_POINT('Ctrl Pts',(-27.8555428563217,83.0853060917096,
81.675015618743));
#216516=CARTESIAN_POINT('Ctrl Pts',(-27.8943606925205,84.1877046395505,
80.511158397832));
#216517=CARTESIAN_POINT('Ctrl Pts',(-27.9154137136888,84.7070185604496,
79.8280233776928));
#216518=CARTESIAN_POINT('Ctrl Pts',(-27.954775756408,85.5408208222249,78.4423817770702));
#216519=CARTESIAN_POINT('Ctrl Pts',(-27.9730483021463,85.8696066992172,
77.7534814086961));
#216520=CARTESIAN_POINT('Ctrl Pts',(-28.0009899984105,86.2602211074579,
76.6796629656115));
#216521=CARTESIAN_POINT('Ctrl Pts',(-28.0103578636748,86.3731278812414,
76.3154541562814));
#216522=CARTESIAN_POINT('Ctrl Pts',(-28.0380380813857,86.6546221253415,
75.2236967172088));
#216523=CARTESIAN_POINT('Ctrl Pts',(-28.0560037213047,86.7722114001575,
74.4849533402767));
#216524=CARTESIAN_POINT('Ctrl Pts',(-28.0906095327986,86.8621334167247,
73.0676475276407));
#216525=CARTESIAN_POINT('Ctrl Pts',(-28.1072187570474,86.8473184090742,
72.3928080836079));
#216526=CARTESIAN_POINT('Ctrl Pts',(-28.1430038445859,86.6913356491575,
70.9441242962121));
#216527=CARTESIAN_POINT('Ctrl Pts',(-28.1618406358991,86.5304058870406,
70.175580916619));
#216528=CARTESIAN_POINT('Ctrl Pts',(-28.1951734533827,86.1210812944039,
68.8779824025966));
#216529=CARTESIAN_POINT('Ctrl Pts',(-28.2094523077273,85.9073574683635,
68.340829905481));
#216530=CARTESIAN_POINT('Ctrl Pts',(-28.2330439245425,85.4884236466741,
67.4775219853328));
#216531=CARTESIAN_POINT('Ctrl Pts',(-28.2423408547897,85.3049865023518,
67.1419094369747));
#216532=CARTESIAN_POINT('Ctrl Pts',(-28.2782578417886,84.5357602216077,
65.8833966628341));
#216533=CARTESIAN_POINT('Ctrl Pts',(-28.3052941562291,83.8395419508508,
65.034402610614));
#216534=CARTESIAN_POINT('Ctrl Pts',(-28.3508743773173,82.4710875276948,
63.7704280698183));
#216535=CARTESIAN_POINT('Ctrl Pts',(-28.3695262107152,81.8557014650617,
63.3043203361268));
#216536=CARTESIAN_POINT('Ctrl Pts',(-28.407353268538,80.5479670079492,62.5012090031384));
#216537=CARTESIAN_POINT('Ctrl Pts',(-28.426232145784,79.8592840491543,62.1651667892801));
#216538=CARTESIAN_POINT('Ctrl Pts',(-28.4729976683636,78.062547718402,61.4946506627506));
#216539=CARTESIAN_POINT('Ctrl Pts',(-28.5015232990402,76.9289262117093,
61.2514541469712));
#216540=CARTESIAN_POINT('Ctrl Pts',(-28.5390377437249,75.3984674866269,
61.1511013270156));
#216541=CARTESIAN_POINT('Ctrl Pts',(-28.5482828995768,75.0178221458842,
61.1445222316161));
#216542=CARTESIAN_POINT('Ctrl Pts',(-28.5757505507809,73.893349166789,61.1792933163559));
#216543=CARTESIAN_POINT('Ctrl Pts',(-28.594122353014,73.153004926618,61.2724482235333));
#216544=CARTESIAN_POINT('Ctrl Pts',(-28.6309418007174,71.6949132916563,
61.5976226793957));
#216545=CARTESIAN_POINT('Ctrl Pts',(-28.649017270183,70.9806297221474,61.8298133038949));
#216546=CARTESIAN_POINT('Ctrl Pts',(-28.6864894179898,69.575702599145,62.4390419718151));
#216547=CARTESIAN_POINT('Ctrl Pts',(-28.7058811506698,68.8908880624085,
62.8204357804223));
#216548=CARTESIAN_POINT('Ctrl Pts',(-28.7342580628242,67.9360519571189,
63.4837221209304));
#216549=CARTESIAN_POINT('Ctrl Pts',(-28.7434809492352,67.6340703127547,
63.7158500381008));
#216550=CARTESIAN_POINT('Ctrl Pts',(-28.7709065445809,66.7747124842914,
64.4449361288401));
#216551=CARTESIAN_POINT('Ctrl Pts',(-28.7892499725978,66.2525531429998,
64.9804777332998));
#216552=CARTESIAN_POINT('Ctrl Pts',(-28.825967005064,65.3147788628337,66.1442571638897));
#216553=CARTESIAN_POINT('Ctrl Pts',(-28.8439537114784,64.9015594364278,
66.7701252758376));
#216554=CARTESIAN_POINT('Ctrl Pts',(-28.8715192451016,64.3702675886859,
67.769070856942));
#216555=CARTESIAN_POINT('Ctrl Pts',(-28.8808941421672,64.2069848415272,
68.1156854715423));
#216556=CARTESIAN_POINT('Ctrl Pts',(-28.8902889611216,64.0608503608518,
68.4693880297961));
#216557=CARTESIAN_POINT('Ctrl Pts',(-29.1863798856003,64.0608503608518,
68.4693880297961));
#216558=CARTESIAN_POINT('Ctrl Pts',(-29.1772971019915,64.2039566764104,
68.1230148146493));
#216559=CARTESIAN_POINT('Ctrl Pts',(-29.1681963644073,64.3635156285741,
67.7834200366463));
#216560=CARTESIAN_POINT('Ctrl Pts',(-29.1407582807609,64.8892662932338,
66.7900910426804));
#216561=CARTESIAN_POINT('Ctrl Pts',(-29.1223061210834,65.3014574016432,
66.1631089739329));
#216562=CARTESIAN_POINT('Ctrl Pts',(-29.0861268663779,66.2363096871553,
64.9983969506667));
#216563=CARTESIAN_POINT('Ctrl Pts',(-29.068189876378,66.7563087681588,64.4628250183807));
#216564=CARTESIAN_POINT('Ctrl Pts',(-29.0406822289049,67.6128254558339,
63.7327731944003));
#216565=CARTESIAN_POINT('Ctrl Pts',(-29.0313471682774,67.914223574994,63.4999911454192));
#216566=CARTESIAN_POINT('Ctrl Pts',(-28.9963513665927,69.0909345083389,
62.6785523531985));
#216567=CARTESIAN_POINT('Ctrl Pts',(-28.9712333861722,70.0323304310186,
62.1931766204282));
#216568=CARTESIAN_POINT('Ctrl Pts',(-28.9361534913813,71.3849850634084,
61.7106575668398));
#216569=CARTESIAN_POINT('Ctrl Pts',(-28.9268151025283,71.7504684387958,
61.599877742482));
#216570=CARTESIAN_POINT('Ctrl Pts',(-28.8986232864933,72.8790142670072,
61.3165687146644));
#216571=CARTESIAN_POINT('Ctrl Pts',(-28.8799524364392,73.6543621125435,
61.2017806268093));
#216572=CARTESIAN_POINT('Ctrl Pts',(-28.8427762630881,75.1809434534785,
61.1284459314993));
#216573=CARTESIAN_POINT('Ctrl Pts',(-28.8245393308412,75.9282621777524,
61.1632193224014));
#216574=CARTESIAN_POINT('Ctrl Pts',(-28.7973642074259,77.0461147177396,
61.3218872138268));
#216575=CARTESIAN_POINT('Ctrl Pts',(-28.7881723803851,77.4220834695785,
61.3939830137662));
#216576=CARTESIAN_POINT('Ctrl Pts',(-28.7605398889289,78.532781424215,61.6633444752674));
#216577=CARTESIAN_POINT('Ctrl Pts',(-28.7419026732506,79.2526837640225,
61.9132892238843));
#216578=CARTESIAN_POINT('Ctrl Pts',(-28.7024162990105,80.7361329678467,
62.594384563092));
#216579=CARTESIAN_POINT('Ctrl Pts',(-28.6816183982419,81.4860140308851,
63.0446887401063));
#216580=CARTESIAN_POINT('Ctrl Pts',(-28.6511205511374,82.4821459250204,
63.8037720993769));
#216581=CARTESIAN_POINT('Ctrl Pts',(-28.641824948786,82.7733845772097,64.0487477801449));
#216582=CARTESIAN_POINT('Ctrl Pts',(-28.6070570799447,83.8229911513047,
65.02169091833));
#216583=CARTESIAN_POINT('Ctrl Pts',(-28.5820663187113,84.4951307407757,
65.8354971314365));
#216584=CARTESIAN_POINT('Ctrl Pts',(-28.5471143492697,85.2527771483029,
67.0509431192));
#216585=CARTESIAN_POINT('Ctrl Pts',(-28.5377911122329,85.43878229314,67.3841804411063));
#216586=CARTESIAN_POINT('Ctrl Pts',(-28.5057992242645,86.0263292297969,
68.5677288913263));
#216587=CARTESIAN_POINT('Ctrl Pts',(-28.4833135204415,86.3425386972941,
69.4564276996115));
#216588=CARTESIAN_POINT('Ctrl Pts',(-28.4510316165937,86.6345637039432,
70.7447829463107));
#216589=CARTESIAN_POINT('Ctrl Pts',(-28.4416982118052,86.7008126253116,
71.120290507038));
#216590=CARTESIAN_POINT('Ctrl Pts',(-28.411148415327,86.8594463816134,72.3690443886639));
#216591=CARTESIAN_POINT('Ctrl Pts',(-28.3901404593192,86.872893009606,73.249356325545));
#216592=CARTESIAN_POINT('Ctrl Pts',(-28.359381835819,86.7525769523979,74.5012789418191));
#216593=CARTESIAN_POINT('Ctrl Pts',(-28.3500534201444,86.6980386709,74.8775490469038));
#216594=CARTESIAN_POINT('Ctrl Pts',(-28.3145658480163,86.4204866664645,
76.3047667337937));
#216595=CARTESIAN_POINT('Ctrl Pts',(-28.2888789614875,86.0729804728404,
77.3262086786382));
#216596=CARTESIAN_POINT('Ctrl Pts',(-28.2531279933201,85.4215351983815,
78.6286589200921));
#216597=CARTESIAN_POINT('Ctrl Pts',(-28.2437348693344,85.2340537504691,
78.9621005282212));
#216598=CARTESIAN_POINT('Ctrl Pts',(-28.2210600401188,84.7386072304263,
79.7512362195004));
#216599=CARTESIAN_POINT('Ctrl Pts',(-28.2078112198607,84.4144054699502,
80.1956830082397));
#216600=CARTESIAN_POINT('Ctrl Pts',(-28.1753363154878,83.5566907558226,
81.2144043629737));
#216601=CARTESIAN_POINT('Ctrl Pts',(-28.1559785536078,82.9948032368779,
81.7613995684301));
#216602=CARTESIAN_POINT('Ctrl Pts',(-28.1238812834247,81.9658428687735,
82.5815420877053));
#216603=CARTESIAN_POINT('Ctrl Pts',(-28.1109864229189,81.5265898795775,
82.8855280811803));
#216604=CARTESIAN_POINT('Ctrl Pts',(-28.0794700449832,80.418330375655,83.5465389759851));
#216605=CARTESIAN_POINT('Ctrl Pts',(-28.0607213368762,79.7326514086105,
83.8710079993923));
#216606=CARTESIAN_POINT('Ctrl Pts',(-28.0217400834737,78.2352384276097,
84.4111238918871));
#216607=CARTESIAN_POINT('Ctrl Pts',(-28.0015951829068,77.4219904435121,
84.6105569535184));
#216608=CARTESIAN_POINT('Ctrl Pts',(-27.9625972218464,75.8528788255984,
84.8233527843671));
#216609=CARTESIAN_POINT('Ctrl Pts',(-27.9441287971005,75.1033342352144,
84.8533811491028));
#216610=CARTESIAN_POINT('Ctrl Pts',(-27.9073341281364,73.5959182828425,
84.7708230227862));
#216611=CARTESIAN_POINT('Ctrl Pts',(-27.888726346834,72.8416347153993,84.6559924550591));
#216612=CARTESIAN_POINT('Ctrl Pts',(-27.8604417150418,71.7318949057894,
84.375652234997));
#216613=CARTESIAN_POINT('Ctrl Pts',(-27.8509640987074,71.364952415787,84.2637479714313));
#216614=CARTESIAN_POINT('Ctrl Pts',(-27.8282682830005,70.492268569434,83.9505537038313));
#216615=CARTESIAN_POINT('Ctrl Pts',(-27.8150795458088,69.9937130697508,
83.7318272038345));
#216616=CARTESIAN_POINT('Ctrl Pts',(-27.7832572038282,68.8435533450949,
83.1296754073216));
#216617=CARTESIAN_POINT('Ctrl Pts',(-27.7645118776768,68.2101260901553,
82.7166516247409));
#216618=CARTESIAN_POINT('Ctrl Pts',(-27.7245009698029,66.9341789384272,
81.6988558809098));
#216619=CARTESIAN_POINT('Ctrl Pts',(-27.7032793625638,66.3110197248183,
81.0769319392354));
#216620=CARTESIAN_POINT('Ctrl Pts',(-27.6722362673775,65.5243560504484,
80.0947421788309));
#216621=CARTESIAN_POINT('Ctrl Pts',(-27.6628149603627,65.3008445051999,
79.7863065048586));
#216622=CARTESIAN_POINT('Ctrl Pts',(-27.6342006950588,64.6641157117326,
78.8120432954197));
#216623=CARTESIAN_POINT('Ctrl Pts',(-27.615329973039,64.3017571268858,78.115547465555));
#216624=CARTESIAN_POINT('Ctrl Pts',(-27.5777488947944,63.7331080256035,
76.694229870837));
#216625=CARTESIAN_POINT('Ctrl Pts',(-27.5592275305226,63.5217585243477,
75.9753180463411));
#216626=CARTESIAN_POINT('Ctrl Pts',(-27.5228483102149,63.2377878973354,
74.5088659335672));
#216627=CARTESIAN_POINT('Ctrl Pts',(-27.5047697867643,63.1655005946628,
73.7646740156392));
#216628=CARTESIAN_POINT('Ctrl Pts',(-27.4770681652961,63.1628123262026,
72.6379771073962));
#216629=CARTESIAN_POINT('Ctrl Pts',(-27.4676780097333,63.1802633466293,
72.2574861405776));
#216630=CARTESIAN_POINT('Ctrl Pts',(-27.4391622788875,63.289501810978,71.0994279551725));
#216631=CARTESIAN_POINT('Ctrl Pts',(-27.4203808244055,63.440046697084,70.3295595189917));
#216632=CARTESIAN_POINT('Ctrl Pts',(-27.3916342990449,63.7787757506774,
69.2033762014802));
#216633=CARTESIAN_POINT('Ctrl Pts',(-27.3819721225719,63.9107637104782,
68.832656384932));
#216634=CARTESIAN_POINT('Ctrl Pts',(-27.3723203524304,64.0608503540383,
68.4693880462876));
#216635=CARTESIAN_POINT('Origin',(-33.5526503323277,75.000050506625,72.9851176492631));
#216636=CARTESIAN_POINT('',(-37.9576288901553,64.0574429649795,68.4641091549305));
#216637=CARTESIAN_POINT('',(-38.2588681851947,64.0574481338172,68.4640966443434));
#216638=CARTESIAN_POINT('',(-33.5526503323277,64.0574429649796,68.4641091549303));
#216639=CARTESIAN_POINT('',(-37.9576293742551,64.0574354028926,68.4641274581798));
#216640=CARTESIAN_POINT('Ctrl Pts',(-37.9576288901553,64.0574429649794,
68.4641091549307));
#216641=CARTESIAN_POINT('Ctrl Pts',(-37.9576291329798,64.0574391718279,
68.4641183358399));
#216642=CARTESIAN_POINT('Ctrl Pts',(-37.9576293758043,64.0574353786878,
68.4641275167543));
#216643=CARTESIAN_POINT('Ctrl Pts',(-37.9576296186288,64.0574315855591,
68.4641366976736));
#216644=CARTESIAN_POINT('',(-38.418062421717,70.6974291912148,84.0154429842386));
#216645=CARTESIAN_POINT('Ctrl Pts',(-37.9576293742551,64.0574354028926,
68.4641274581798));
#216646=CARTESIAN_POINT('Ctrl Pts',(-37.9743923970413,63.7955819506003,
69.0979181590909));
#216647=CARTESIAN_POINT('Ctrl Pts',(-37.9910143370797,63.5892858234739,
69.753262138451));
#216648=CARTESIAN_POINT('Ctrl Pts',(-38.0246878629418,63.2931806340481,
71.0890404407701));
#216649=CARTESIAN_POINT('Ctrl Pts',(-38.0416261579981,63.2033680661301,
71.7668394361827));
#216650=CARTESIAN_POINT('Ctrl Pts',(-38.069412644704,63.1518376883327,72.9028136644737));
#216651=CARTESIAN_POINT('Ctrl Pts',(-38.0804609656725,63.1574159035511,
73.3578466686248));
#216652=CARTESIAN_POINT('Ctrl Pts',(-38.1107350192916,63.2436885873193,
74.5909878341748));
#216653=CARTESIAN_POINT('Ctrl Pts',(-38.1301458598497,63.3752737739155,
75.3632308490525));
#216654=CARTESIAN_POINT('Ctrl Pts',(-38.1586472136151,63.6827161611728,
76.484141368582));
#216655=CARTESIAN_POINT('Ctrl Pts',(-38.1679026268872,63.8011177859933,
76.8463520341654));
#216656=CARTESIAN_POINT('Ctrl Pts',(-38.1865718759954,64.0736906924759,
77.5614275400821));
#216657=CARTESIAN_POINT('Ctrl Pts',(-38.1959758912443,64.2280236950087,
77.9137470663033));
#216658=CARTESIAN_POINT('Ctrl Pts',(-38.2228550046262,64.7144503548113,
78.8916927172907));
#216659=CARTESIAN_POINT('Ctrl Pts',(-38.2403936753872,65.085880789799,79.4959123706368));
#216660=CARTESIAN_POINT('Ctrl Pts',(-38.2709383733594,65.8347216109281,
80.5000150089951));
#216661=CARTESIAN_POINT('Ctrl Pts',(-38.2841616948544,66.1901443631909,
80.9137044981226));
#216662=CARTESIAN_POINT('Ctrl Pts',(-38.3176332553364,67.1486407712281,
81.8849868311498));
#216663=CARTESIAN_POINT('Ctrl Pts',(-38.3379297371556,67.7835553047492,
82.4071404556692));
#216664=CARTESIAN_POINT('Ctrl Pts',(-38.3680731510726,68.8168416866319,
83.0907477428116));
#216665=CARTESIAN_POINT('Ctrl Pts',(-38.3782385943951,69.178411869877,83.3032741798193));
#216666=CARTESIAN_POINT('Ctrl Pts',(-38.3987282947051,69.9231681713914,
83.6894003576084));
#216667=CARTESIAN_POINT('Ctrl Pts',(-38.4090386083825,70.3058599943613,
83.8626621801093));
#216668=CARTESIAN_POINT('Ctrl Pts',(-38.4193726539769,70.6969410188162,
84.0152321705287));
#216669=CARTESIAN_POINT('',(-38.717056908316,70.6974160226281,84.0154504430313));
#216670=CARTESIAN_POINT('',(-38.4175364832709,70.69729039136,84.0153684626757));
#216671=CARTESIAN_POINT('Ctrl Pts',(-38.2588685144218,64.0574429649797,
68.4641091549301));
#216672=CARTESIAN_POINT('Ctrl Pts',(-38.2753921140801,63.7980242826514,
69.0920037570411));
#216673=CARTESIAN_POINT('Ctrl Pts',(-38.2919909110401,63.5931278905779,
69.7410687161469));
#216674=CARTESIAN_POINT('Ctrl Pts',(-38.3247086479941,63.2978613845077,
71.0629606633982));
#216675=CARTESIAN_POINT('Ctrl Pts',(-38.3408123281424,63.2073159003245,
71.7331880602663));
#216676=CARTESIAN_POINT('Ctrl Pts',(-38.3681764716619,63.152435191933,72.8567104434083));
#216677=CARTESIAN_POINT('Ctrl Pts',(-38.3791668041158,63.1561079854806,
73.3068378553902));
#216678=CARTESIAN_POINT('Ctrl Pts',(-38.404419780308,63.2237743787431,74.3443579761159));
#216679=CARTESIAN_POINT('Ctrl Pts',(-38.4185812414995,63.3061147155748,
74.9293606886987));
#216680=CARTESIAN_POINT('Ctrl Pts',(-38.4507641769266,63.5907017532673,
76.2354439569314));
#216681=CARTESIAN_POINT('Ctrl Pts',(-38.4690337585594,63.818367341293,76.948425810389));
#216682=CARTESIAN_POINT('Ctrl Pts',(-38.5056409803773,64.4099354287515,
78.3336123336521));
#216683=CARTESIAN_POINT('Ctrl Pts',(-38.5237690303283,64.7747131400765,
79.0017114320047));
#216684=CARTESIAN_POINT('Ctrl Pts',(-38.5602504821622,65.619694371161,80.2477433922699));
#216685=CARTESIAN_POINT('Ctrl Pts',(-38.5785684555972,66.0958665941443,
80.8242712373352));
#216686=CARTESIAN_POINT('Ctrl Pts',(-38.6162190079843,67.1937976489437,
81.9235023376853));
#216687=CARTESIAN_POINT('Ctrl Pts',(-38.6355332715921,67.821437222446,82.4349754727852));
#216688=CARTESIAN_POINT('Ctrl Pts',(-38.6653949765358,68.8416573233498,
83.1056540434989));
#216689=CARTESIAN_POINT('Ctrl Pts',(-38.6755171178592,69.1987422076271,
83.3144877599833));
#216690=CARTESIAN_POINT('Ctrl Pts',(-38.6956648674305,69.9338189535861,
83.6942191651615));
#216691=CARTESIAN_POINT('Ctrl Pts',(-38.7056764744093,70.311333866345,83.8648002743078));
#216692=CARTESIAN_POINT('Ctrl Pts',(-38.7156810426871,70.6970057304839,
84.0152574158675));
#216693=CARTESIAN_POINT('Origin',(-33.5526503323277,75.000050506625,72.9851176492631));
#216694=CARTESIAN_POINT('',(-36.4450710296185,64.0574429649796,68.4641091549303));
#216695=CARTESIAN_POINT('Ctrl Pts',(-38.2588681851947,64.0574481338172,
68.4640966443434));
#216696=CARTESIAN_POINT('Ctrl Pts',(-38.2414434766608,64.3310149227641,
67.8019602396254));
#216697=CARTESIAN_POINT('Ctrl Pts',(-38.2243669723514,64.6641105528954,
67.1660294946634));
#216698=CARTESIAN_POINT('Ctrl Pts',(-38.1901425424151,65.4307058494362,
65.9784220822238));
#216699=CARTESIAN_POINT('Ctrl Pts',(-38.1730504638907,65.8597525886812,
65.4272684079564));
#216700=CARTESIAN_POINT('Ctrl Pts',(-38.1448445435794,66.6516037811045,
64.5768018527136));
#216701=CARTESIAN_POINT('Ctrl Pts',(-38.1336955927266,66.9881920041458,
64.2554863627001));
#216702=CARTESIAN_POINT('Ctrl Pts',(-38.1005010922852,68.0368132134697,
63.3663092421297));
#216703=CARTESIAN_POINT('Ctrl Pts',(-38.0781641925283,68.7963532967956,
62.8597893706182));
#216704=CARTESIAN_POINT('Ctrl Pts',(-38.0375951524959,70.2844060093473,
62.0982906842396));
#216705=CARTESIAN_POINT('Ctrl Pts',(-38.019354404517,70.9943439608194,61.8175473993704));
#216706=CARTESIAN_POINT('Ctrl Pts',(-37.9853984113513,72.3315569437106,
61.4328033878864));
#216707=CARTESIAN_POINT('Ctrl Pts',(-37.9698933723247,72.9497326310281,
61.307231540618));
#216708=CARTESIAN_POINT('Ctrl Pts',(-37.9453930639585,73.9518904771438,
61.1857232957817));
#216709=CARTESIAN_POINT('Ctrl Pts',(-37.9362344946197,74.3308063654,61.158179777539));
#216710=CARTESIAN_POINT('Ctrl Pts',(-37.9052180248771,75.6095443451553,
61.1268859598937));
#216711=CARTESIAN_POINT('Ctrl Pts',(-37.8830430633134,76.5082777725493,
61.2074109640022));
#216712=CARTESIAN_POINT('Ctrl Pts',(-37.8424912106608,78.1373424093565,
61.5430432053088));
#216713=CARTESIAN_POINT('Ctrl Pts',(-37.8241156632569,78.8688244084466,
61.7692243491527));
#216714=CARTESIAN_POINT('Ctrl Pts',(-37.7960651734842,79.9243127389037,
62.2112349365072));
#216715=CARTESIAN_POINT('Ctrl Pts',(-37.7866917729287,80.2679321408877,
62.3750125899686));
#216716=CARTESIAN_POINT('Ctrl Pts',(-37.7589614148258,81.2610901329231,
62.9085355290734));
#216717=CARTESIAN_POINT('Ctrl Pts',(-37.7409544483602,81.8841843457121,
63.3235014855631));
#216718=CARTESIAN_POINT('Ctrl Pts',(-37.7036161430274,83.0709458880184,
64.2872940121883));
#216719=CARTESIAN_POINT('Ctrl Pts',(-37.6842369621448,83.6275561640151,
64.8390986245063));
#216720=CARTESIAN_POINT('Ctrl Pts',(-37.6463538210091,84.6135950831142,
66.0319626834408));
#216721=CARTESIAN_POINT('Ctrl Pts',(-37.6278611249987,85.0430814331657,
66.6681453231041));
#216722=CARTESIAN_POINT('Ctrl Pts',(-37.5996702665547,85.5893278172295,
67.6755133465216));
#216723=CARTESIAN_POINT('Ctrl Pts',(-37.590272072703,85.7543378558918,68.0182278249807));
#216724=CARTESIAN_POINT('Ctrl Pts',(-37.5624481356148,86.1940422193922,
69.0565773840484));
#216725=CARTESIAN_POINT('Ctrl Pts',(-37.5443772977862,86.419676216308,69.7709258240512));
#216726=CARTESIAN_POINT('Ctrl Pts',(-37.5069384910856,86.7403526451989,
71.2657909721727));
#216727=CARTESIAN_POINT('Ctrl Pts',(-37.4875270028055,86.8282110558048,
72.0441663747342));
#216728=CARTESIAN_POINT('Ctrl Pts',(-37.4495750678847,86.8490780878975,
73.5918578648581));
#216729=CARTESIAN_POINT('Ctrl Pts',(-37.4310387646194,86.7849732901166,
74.35741132429));
#216730=CARTESIAN_POINT('Ctrl Pts',(-37.4028147437794,86.579152016589,75.4848619131025));
#216731=CARTESIAN_POINT('Ctrl Pts',(-37.3934213460348,86.4930472056369,
75.8548457269552));
#216732=CARTESIAN_POINT('Ctrl Pts',(-37.3655903757164,86.1850285228373,
76.9392906385991));
#216733=CARTESIAN_POINT('Ctrl Pts',(-37.3475139631943,85.9130691799396,
77.6375624088148));
#216734=CARTESIAN_POINT('Ctrl Pts',(-37.310072347362,85.225841874519,79.0037821457513));
#216735=CARTESIAN_POINT('Ctrl Pts',(-37.2906678380084,84.8063176271644,
79.6655555737842));
#216736=CARTESIAN_POINT('Ctrl Pts',(-37.2527790121884,83.8528030073251,
80.8841842070412));
#216737=CARTESIAN_POINT('Ctrl Pts',(-37.2342874438966,83.3235642099088,
81.4400337256653));
#216738=CARTESIAN_POINT('Ctrl Pts',(-37.2061467389023,82.4575542992148,
82.1888991369763));
#216739=CARTESIAN_POINT('Ctrl Pts',(-37.1967849130386,82.1589870568592,
82.4229978799163));
#216740=CARTESIAN_POINT('Ctrl Pts',(-37.1690316885729,81.2398185526467,
83.0749419796226));
#216741=CARTESIAN_POINT('Ctrl Pts',(-37.151006461953,80.5903269559619,83.4487724206279));
#216742=CARTESIAN_POINT('Ctrl Pts',(-37.1136623142814,79.1981706352352,
84.0832158447184));
#216743=CARTESIAN_POINT('Ctrl Pts',(-37.0943072151199,78.4560178963457,
84.3362533233397));
#216744=CARTESIAN_POINT('Ctrl Pts',(-37.0565881341238,76.9503097399315,
84.6881302251893));
#216745=CARTESIAN_POINT('Ctrl Pts',(-37.0382056349772,76.1911765655033,
84.7895761321428));
#216746=CARTESIAN_POINT('Ctrl Pts',(-37.0102222952616,75.0488340970667,
84.8308524154469));
#216747=CARTESIAN_POINT('Ctrl Pts',(-37.0009036630239,74.6696514374755,
84.8263442654468));
#216748=CARTESIAN_POINT('Ctrl Pts',(-36.9732759310988,73.5450728746751,
84.7589078589771));
#216749=CARTESIAN_POINT('Ctrl Pts',(-36.9553346668574,72.804721093565,84.643574932408));
#216750=CARTESIAN_POINT('Ctrl Pts',(-36.9182469519714,71.3257018042379,
84.2672040914431));
#216751=CARTESIAN_POINT('Ctrl Pts',(-36.8990684764574,70.5919789919822,
84.0012518956182));
#216752=CARTESIAN_POINT('Ctrl Pts',(-36.8616582722482,69.2024366261997,
83.3363644730011));
#216753=CARTESIAN_POINT('Ctrl Pts',(-36.8434135515956,68.5485245096775,
82.9419473064971));
#216754=CARTESIAN_POINT('Ctrl Pts',(-36.8155999070953,67.6325819179565,
82.2611353472256));
#216755=CARTESIAN_POINT('Ctrl Pts',(-36.8063125882316,67.3391630212681,
82.0203210204782));
#216756=CARTESIAN_POINT('Ctrl Pts',(-36.7788002724731,66.5036590832524,
81.2646004878822));
#216757=CARTESIAN_POINT('Ctrl Pts',(-36.7609404523299,65.9981986920098,
80.7120296317288));
#216758=CARTESIAN_POINT('Ctrl Pts',(-36.7240649617963,65.0806505347689,
79.4957542552416));
#216759=CARTESIAN_POINT('Ctrl Pts',(-36.7050131040977,64.6751964958442,
78.8315069658785));
#216760=CARTESIAN_POINT('Ctrl Pts',(-36.6678205147483,64.0073444470835,
77.4480743136396));
#216761=CARTESIAN_POINT('Ctrl Pts',(-36.6496859095303,63.7436413231345,
76.7335610705654));
#216762=CARTESIAN_POINT('Ctrl Pts',(-36.6219871628855,63.4534983234491,
75.6311978500145));
#216763=CARTESIAN_POINT('Ctrl Pts',(-36.6127084198458,63.3745175967954,
75.2592309883459));
#216764=CARTESIAN_POINT('Ctrl Pts',(-36.5852547483898,63.1938055523443,
74.1471221349221));
#216765=CARTESIAN_POINT('Ctrl Pts',(-36.5674386766604,63.1440321801278,
73.4004552593166));
#216766=CARTESIAN_POINT('Ctrl Pts',(-36.5304558753239,63.1868329889988,
71.8702137011023));
#216767=CARTESIAN_POINT('Ctrl Pts',(-36.5112359744591,63.2865808289669,
71.090456946076));
#216768=CARTESIAN_POINT('Ctrl Pts',(-36.4830518847883,63.5481892516628,
69.9552594336278));
#216769=CARTESIAN_POINT('Ctrl Pts',(-36.4739208179995,63.6515484448178,
69.5885503747416));
#216770=CARTESIAN_POINT('Ctrl Pts',(-36.4582052209673,63.8586852775821,
68.9696380730014));
#216771=CARTESIAN_POINT('Ctrl Pts',(-36.451650075586,63.9537685944047,68.7150416516842));
#216772=CARTESIAN_POINT('Ctrl Pts',(-36.4450710296185,64.0574429649796,
68.4641091549303));
#216773=CARTESIAN_POINT('',(-36.143425535889,64.0574429649796,68.4641091549303));
#216774=CARTESIAN_POINT('',(-33.5526503323277,64.0574429649796,68.4641091549303));
#216775=CARTESIAN_POINT('Ctrl Pts',(-36.143425535889,64.0574429649796,68.4641091549303));
#216776=CARTESIAN_POINT('Ctrl Pts',(-36.150344663908,63.949728708768,68.7248197538689));
#216777=CARTESIAN_POINT('Ctrl Pts',(-36.157295342917,63.8512897815639,68.9894811601397));
#216778=CARTESIAN_POINT('Ctrl Pts',(-36.1736752316992,63.6424020128784,
69.6192352301631));
#216779=CARTESIAN_POINT('Ctrl Pts',(-36.1831080458738,63.5399756356306,
69.9864465986742));
#216780=CARTESIAN_POINT('Ctrl Pts',(-36.2108803965733,63.289093886627,71.0889039027289));
#216781=CARTESIAN_POINT('Ctrl Pts',(-36.2289847357361,63.1925500483805,
71.8340004654652));
#216782=CARTESIAN_POINT('Ctrl Pts',(-36.2657906428265,63.1417460476561,
73.3297640466191));
#216783=CARTESIAN_POINT('Ctrl Pts',(-36.2843345525679,63.1870974288601,
74.0770488854905));
#216784=CARTESIAN_POINT('Ctrl Pts',(-36.3118251489354,63.3610984532145,
75.1893089803292));
#216785=CARTESIAN_POINT('Ctrl Pts',(-36.3210376246501,63.4375713261465,
75.5605282235205));
#216786=CARTESIAN_POINT('Ctrl Pts',(-36.3489337273685,63.7210228696664,
76.6653419480273));
#216787=CARTESIAN_POINT('Ctrl Pts',(-36.3678039581695,63.9811134418178,
77.3832454842242));
#216788=CARTESIAN_POINT('Ctrl Pts',(-36.4058033435647,64.6448449919314,
78.7785158191203));
#216789=CARTESIAN_POINT('Ctrl Pts',(-36.4246857004833,65.0506980060946,
79.4507291466379));
#216790=CARTESIAN_POINT('Ctrl Pts',(-36.4622871396387,65.9677741190266,
80.6764745687496));
#216791=CARTESIAN_POINT('Ctrl Pts',(-36.4808155600896,66.4712811169162,
81.2312737195149));
#216792=CARTESIAN_POINT('Ctrl Pts',(-36.5172166971965,67.5751281626403,
82.2375453080713));
#216793=CARTESIAN_POINT('Ctrl Pts',(-36.535310990023,68.1728120791836,82.6869578644967));
#216794=CARTESIAN_POINT('Ctrl Pts',(-36.5630353317565,69.1332668695483,
83.2761782650808));
#216795=CARTESIAN_POINT('Ctrl Pts',(-36.5724321849271,69.4671444690562,
83.4594686865642));
#216796=CARTESIAN_POINT('Ctrl Pts',(-36.6009705412535,70.5126686807691,
83.9694738677818));
#216797=CARTESIAN_POINT('Ctrl Pts',(-36.619769591115,71.2483574496679,84.2420035092752));
#216798=CARTESIAN_POINT('Ctrl Pts',(-36.6572285748738,72.7297284296824,
84.6292624832212));
#216799=CARTESIAN_POINT('Ctrl Pts',(-36.6757180584941,73.4702456101325,
84.7494781144531));
#216800=CARTESIAN_POINT('Ctrl Pts',(-36.7119578321393,74.9596528302929,
84.8481817928625));
#216801=CARTESIAN_POINT('Ctrl Pts',(-36.7299152908744,75.7051514321559,
84.8272777263948));
#216802=CARTESIAN_POINT('Ctrl Pts',(-36.75746172588,76.8214862152428,84.6901335000161));
#216803=CARTESIAN_POINT('Ctrl Pts',(-36.7668154143757,77.1967758641369,
84.6255395369988));
#216804=CARTESIAN_POINT('Ctrl Pts',(-36.7952297270275,78.3317958994633,
84.3733289843863));
#216805=CARTESIAN_POINT('Ctrl Pts',(-36.8139300780076,79.0766036901995,
84.1284385623949));
#216806=CARTESIAN_POINT('Ctrl Pts',(-36.8512270455754,80.4775485634038,
83.5084036045176));
#216807=CARTESIAN_POINT('Ctrl Pts',(-36.869675612657,81.1329102440116,83.1404399745297));
#216808=CARTESIAN_POINT('Ctrl Pts',(-36.9067267671718,82.3918362796064,
82.2670205758651));
#216809=CARTESIAN_POINT('Ctrl Pts',(-36.9255158012893,82.9888378618979,
81.7584577091205));
#216810=CARTESIAN_POINT('Ctrl Pts',(-36.9538947456751,83.7952725063491,
80.9204296069613));
#216811=CARTESIAN_POINT('Ctrl Pts',(-36.963214092309,84.0458597771048,80.6335449786799));
#216812=CARTESIAN_POINT('Ctrl Pts',(-36.9914822902786,84.7674231956479,
79.7222961302464));
#216813=CARTESIAN_POINT('Ctrl Pts',(-37.0101030569021,85.1907823934553,
79.0629569003044));
#216814=CARTESIAN_POINT('Ctrl Pts',(-37.0472576464522,85.8864387837798,
77.6997198682105));
#216815=CARTESIAN_POINT('Ctrl Pts',(-37.065612430509,86.1627648953464,77.0019248131487));
#216816=CARTESIAN_POINT('Ctrl Pts',(-37.1016656105856,86.579429173952,75.5651215855737));
#216817=CARTESIAN_POINT('Ctrl Pts',(-37.1195806184897,86.7191342402651,
74.8294348117883));
#216818=CARTESIAN_POINT('Ctrl Pts',(-37.1470332023142,86.8239323455018,
73.7067268535619));
#216819=CARTESIAN_POINT('Ctrl Pts',(-37.1563288769829,86.8410126474363,
73.3264636012985));
#216820=CARTESIAN_POINT('Ctrl Pts',(-37.1919423809732,86.8361742115752,
71.8605275850765));
#216821=CARTESIAN_POINT('Ctrl Pts',(-37.2177409034923,86.6833223747396,
70.7806478277577));
#216822=CARTESIAN_POINT('Ctrl Pts',(-37.2535315604924,86.2806834306116,
69.3693936270167));
#216823=CARTESIAN_POINT('Ctrl Pts',(-37.2628531615979,86.1581434925881,
69.0072912123014));
#216824=CARTESIAN_POINT('Ctrl Pts',(-37.2852523240675,85.8188085323026,
68.1444799016979));
#216825=CARTESIAN_POINT('Ctrl Pts',(-37.2982983178231,85.5845126000387,
67.6515950853675));
#216826=CARTESIAN_POINT('Ctrl Pts',(-37.3298555333421,84.9447047871049,
66.5151714252758));
#216827=CARTESIAN_POINT('Ctrl Pts',(-37.3484845848829,84.5095695974514,
65.8910783032959));
#216828=CARTESIAN_POINT('Ctrl Pts',(-37.3891037638151,83.422752591122,64.6136645209313));
#216829=CARTESIAN_POINT('Ctrl Pts',(-37.4110587849797,82.7484795689489,
63.9859514052492));
#216830=CARTESIAN_POINT('Ctrl Pts',(-37.4427893467416,81.7016955582058,
63.2171591033633));
#216831=CARTESIAN_POINT('Ctrl Pts',(-37.4521155254852,81.3842235651512,
63.0067713299031));
#216832=CARTESIAN_POINT('Ctrl Pts',(-37.4813623614136,80.3502700995172,
62.3911482571134));
#216833=CARTESIAN_POINT('Ctrl Pts',(-37.5010298289139,79.6014209793702,
62.0450794621067));
#216834=CARTESIAN_POINT('Ctrl Pts',(-37.5393383871761,78.1164497815894,
61.5384950013363));
#216835=CARTESIAN_POINT('Ctrl Pts',(-37.5576437284937,77.3889305276865,
61.3648605223285));
#216836=CARTESIAN_POINT('Ctrl Pts',(-37.5941044591884,75.8967514857712,
61.1548764318305));
#216837=CARTESIAN_POINT('Ctrl Pts',(-37.6125360809817,75.1351187113621,
61.1217105030284));
#216838=CARTESIAN_POINT('Ctrl Pts',(-37.6405703393137,73.994637819479,61.1819464044539));
#216839=CARTESIAN_POINT('Ctrl Pts',(-37.6499529261285,73.6148805630276,
61.2204666865765));
#216840=CARTESIAN_POINT('Ctrl Pts',(-37.6818356456923,72.3210422946476,
61.4152303066326));
#216841=CARTESIAN_POINT('Ctrl Pts',(-37.7041476426852,71.4238047089491,
61.6603725433316));
#216842=CARTESIAN_POINT('Ctrl Pts',(-37.7363127895092,70.211192631959,62.1503529944448));
#216843=CARTESIAN_POINT('Ctrl Pts',(-37.7457068258623,69.8650992012847,
62.3100269910231));
#216844=CARTESIAN_POINT('Ctrl Pts',(-37.7748819757287,68.8071456430532,
62.8614988235704));
#216845=CARTESIAN_POINT('Ctrl Pts',(-37.7944363211069,68.1275159740027,
63.3099945510022));
#216846=CARTESIAN_POINT('Ctrl Pts',(-37.8262409401161,67.1261775375445,
64.1299109310361));
#216847=CARTESIAN_POINT('Ctrl Pts',(-37.8381647281714,66.7721994428131,
64.4578069790688));
#216848=CARTESIAN_POINT('Ctrl Pts',(-37.8678433035642,65.9370428220467,
65.3319809651629));
#216849=CARTESIAN_POINT('Ctrl Pts',(-37.8853680887045,65.4843604535277,
65.9027271549346));
#216850=CARTESIAN_POINT('Ctrl Pts',(-37.921291353889,64.6836765487467,67.1288042814053));
#216851=CARTESIAN_POINT('Ctrl Pts',(-37.9396026305779,64.3390303884866,
67.7825575347635));
#216852=CARTESIAN_POINT('Ctrl Pts',(-37.9576288901553,64.0574429649794,
68.4641091549307));
#216853=CARTESIAN_POINT('Origin',(-33.5526503323277,75.000050506625,72.9851176492631));
#216854=CARTESIAN_POINT('',(-34.329622639475,64.0574429649796,68.4641091549303));
#216855=CARTESIAN_POINT('',(-34.6308727569695,64.0574429676145,68.4641091485529));
#216856=CARTESIAN_POINT('',(-33.5526503323277,64.0574429649796,68.4641091549303));
#216857=CARTESIAN_POINT('Ctrl Pts',(-34.329622639475,64.0574429649796,68.4641091549303));
#216858=CARTESIAN_POINT('Ctrl Pts',(-34.3328410372056,64.007573846542,68.5848119123337));
#216859=CARTESIAN_POINT('Ctrl Pts',(-34.3360540786868,63.959688302845,68.7063725776957));
#216860=CARTESIAN_POINT('Ctrl Pts',(-34.3580359830751,63.6448520668864,
69.5461309260396));
#216861=CARTESIAN_POINT('Ctrl Pts',(-34.376557966046,63.44616071442,70.2879342041745));
#216862=CARTESIAN_POINT('Ctrl Pts',(-34.4047790580826,63.2582236639502,
71.4185685693466));
#216863=CARTESIAN_POINT('Ctrl Pts',(-34.4141806967683,63.2139971953326,
71.7962021308897));
#216864=CARTESIAN_POINT('Ctrl Pts',(-34.4420214994181,63.1368760532764,
72.9211034112473));
#216865=CARTESIAN_POINT('Ctrl Pts',(-34.4601026172894,63.1564931489113,
73.6700676863727));
#216866=CARTESIAN_POINT('Ctrl Pts',(-34.4975535582399,63.3407866732681,
75.1879448697782));
#216867=CARTESIAN_POINT('Ctrl Pts',(-34.5169664948619,63.5115530869257,
75.9524904167847));
#216868=CARTESIAN_POINT('Ctrl Pts',(-34.5549000929086,63.9963963469406,
77.4220724239963));
#216869=CARTESIAN_POINT('Ctrl Pts',(-34.5734177476563,64.3064317654138,
78.1245240046365));
#216870=CARTESIAN_POINT('Ctrl Pts',(-34.6016076709931,64.8682642371642,
79.1227957722569));
#216871=CARTESIAN_POINT('Ctrl Pts',(-34.6109892258484,65.0701790035698,
79.4443619490049));
#216872=CARTESIAN_POINT('Ctrl Pts',(-34.6387895248276,65.7147305456016,
80.3690188391609));
#216873=CARTESIAN_POINT('Ctrl Pts',(-34.6568442825143,66.199410787854,80.9404872681069));
#216874=CARTESIAN_POINT('Ctrl Pts',(-34.6936647548305,67.2776918025048,
81.9918041354446));
#216875=CARTESIAN_POINT('Ctrl Pts',(-34.7124516774763,67.8702515653957,
82.4677956902649));
#216876=CARTESIAN_POINT('Ctrl Pts',(-34.7496662449242,69.1415892072909,
83.302081586579));
#216877=CARTESIAN_POINT('Ctrl Pts',(-34.7680254416173,69.8178417682874,
83.657794692478));
#216878=CARTESIAN_POINT('Ctrl Pts',(-34.7960437038153,70.8758878011957,
84.0899040321921));
#216879=CARTESIAN_POINT('Ctrl Pts',(-34.8054165914355,71.2349247367758,
84.2167170773129));
#216880=CARTESIAN_POINT('Ctrl Pts',(-34.8331421595484,72.3150444718224,
84.5405946628289));
#216881=CARTESIAN_POINT('Ctrl Pts',(-34.8511315453349,73.0493501182373,
84.6869583952719));
#216882=CARTESIAN_POINT('Ctrl Pts',(-34.8854695763134,74.4528595272905,
84.8308497642501));
#216883=CARTESIAN_POINT('Ctrl Pts',(-34.9017898275013,75.1177068099017,
84.8428972389196));
#216884=CARTESIAN_POINT('Ctrl Pts',(-34.936406968855,76.528197800239,84.7497731105241));
#216885=CARTESIAN_POINT('Ctrl Pts',(-34.9543702819887,77.2699683015172,
84.6294221197));
#216886=CARTESIAN_POINT('Ctrl Pts',(-34.9898344684854,78.6803005161217,
84.2606291027832));
#216887=CARTESIAN_POINT('Ctrl Pts',(-35.0072655248959,79.3477930374311,
84.0204485537004));
#216888=CARTESIAN_POINT('Ctrl Pts',(-35.0429456340828,80.678985892876,83.4018063075007));
#216889=CARTESIAN_POINT('Ctrl Pts',(-35.0611283723938,81.3357223847079,
83.0159192206579));
#216890=CARTESIAN_POINT('Ctrl Pts',(-35.0958873047512,82.4910163575538,
82.1780881374089));
#216891=CARTESIAN_POINT('Ctrl Pts',(-35.1122714837876,82.9970305716071,
81.7414635134517));
#216892=CARTESIAN_POINT('Ctrl Pts',(-35.1469067087876,83.9992025561383,
80.7170089785071));
#216893=CARTESIAN_POINT('Ctrl Pts',(-35.1652695219503,84.480438013047,80.1187797735805));
#216894=CARTESIAN_POINT('Ctrl Pts',(-35.193204737113,85.1091767267621,79.1601089106799));
#216895=CARTESIAN_POINT('Ctrl Pts',(-35.2025108666628,85.3023859788698,
78.8320684461682));
#216896=CARTESIAN_POINT('Ctrl Pts',(-35.2263321118681,85.7580152097419,
77.9655398777807));
#216897=CARTESIAN_POINT('Ctrl Pts',(-35.2406388975228,85.9959943942473,
77.4154256306083));
#216898=CARTESIAN_POINT('Ctrl Pts',(-35.2736399963111,86.4423444486803,
76.1228501451394));
#216899=CARTESIAN_POINT('Ctrl Pts',(-35.2924354339417,86.6219276736402,
75.3732997522042));
#216900=CARTESIAN_POINT('Ctrl Pts',(-35.3300841136658,86.834912514404,73.8376535630978));
#216901=CARTESIAN_POINT('Ctrl Pts',(-35.3486765129286,86.8653741790135,
73.0549259568729));
#216902=CARTESIAN_POINT('Ctrl Pts',(-35.3857942940093,86.7735803233313,
71.5273709295168));
#216903=CARTESIAN_POINT('Ctrl Pts',(-35.4041420580473,86.6578322326881,
70.7857625520058));
#216904=CARTESIAN_POINT('Ctrl Pts',(-35.4401939098107,86.2882005631754,
69.3359748366212));
#216905=CARTESIAN_POINT('Ctrl Pts',(-35.4581130644233,86.0354513284752,
68.6309814524176));
#216906=CARTESIAN_POINT('Ctrl Pts',(-35.4855759339169,85.556399636919,67.6103399887257));
#216907=CARTESIAN_POINT('Ctrl Pts',(-35.4948726091547,85.3783642430428,
67.2741329989908));
#216908=CARTESIAN_POINT('Ctrl Pts',(-35.531338005368,84.6135679832816,65.9841451450563));
#216909=CARTESIAN_POINT('Ctrl Pts',(-35.5579864562403,83.908981791799,65.1070292498714));
#216910=CARTESIAN_POINT('Ctrl Pts',(-35.5946951251752,82.8122259131197,
64.0802461994236));
#216911=CARTESIAN_POINT('Ctrl Pts',(-35.6040421534392,82.5201421013164,
63.8322467533819));
#216912=CARTESIAN_POINT('Ctrl Pts',(-35.6295659956507,81.6833788311474,
63.1889136151298));
#216913=CARTESIAN_POINT('Ctrl Pts',(-35.6457034022072,81.1162452310444,
62.8251642144548));
#216914=CARTESIAN_POINT('Ctrl Pts',(-35.680277594224,79.8609652453171,62.1634304279172));
#216915=CARTESIAN_POINT('Ctrl Pts',(-35.6986116870204,79.1691773955946,
61.8785522175689));
#216916=CARTESIAN_POINT('Ctrl Pts',(-35.7258814921413,78.0907288638883,
61.5495118547579));
#216917=CARTESIAN_POINT('Ctrl Pts',(-35.735072873367,77.721115173045,61.4559728680872));
#216918=CARTESIAN_POINT('Ctrl Pts',(-35.7628238764255,76.600692547838,61.2293156692559));
#216919=CARTESIAN_POINT('Ctrl Pts',(-35.7815886916175,75.8409082877967,
61.1506814660122));
#216920=CARTESIAN_POINT('Ctrl Pts',(-35.8211037742345,74.2212846613405,
61.139900525995));
#216921=CARTESIAN_POINT('Ctrl Pts',(-35.8416699054654,73.3656228487008,
61.2273840662669));
#216922=CARTESIAN_POINT('Ctrl Pts',(-35.8810222115305,71.7960163506922,
61.5626411689096));
#216923=CARTESIAN_POINT('Ctrl Pts',(-35.899392301876,71.0815089746368,61.7876248417063));
#216924=CARTESIAN_POINT('Ctrl Pts',(-35.9360511252781,69.6906469837769,
62.3751354523281));
#216925=CARTESIAN_POINT('Ctrl Pts',(-35.9546215154439,69.0185986053835,
62.7389616667079));
#216926=CARTESIAN_POINT('Ctrl Pts',(-35.98283479605,68.0687604892494,63.3786674373421));
#216927=CARTESIAN_POINT('Ctrl Pts',(-35.9922707319748,67.7618576907462,
63.6077387753892));
#216928=CARTESIAN_POINT('Ctrl Pts',(-36.0150469978111,67.0422585983395,
64.2012535376619));
#216929=CARTESIAN_POINT('Ctrl Pts',(-36.0283551584318,66.6428322592933,
64.5803793674515));
#216930=CARTESIAN_POINT('Ctrl Pts',(-36.0602688669262,65.7615479882361,
65.5420463597641));
#216931=CARTESIAN_POINT('Ctrl Pts',(-36.0789854907851,65.3062029861294,
66.1456327275155));
#216932=CARTESIAN_POINT('Ctrl Pts',(-36.1128442950801,64.5825234260087,
67.3238345517627));
#216933=CARTESIAN_POINT('Ctrl Pts',(-36.1280349982047,64.2970367858784,
67.884198465803));
#216934=CARTESIAN_POINT('Ctrl Pts',(-36.143425535889,64.0574429649796,68.4641091549303));
#216935=CARTESIAN_POINT('Ctrl Pts',(-36.4450710296185,64.0574429649796,
68.4641091549303));
#216936=CARTESIAN_POINT('Ctrl Pts',(-36.4298164832544,64.2978281972046,
67.8822829410793));
#216937=CARTESIAN_POINT('Ctrl Pts',(-36.4143869921359,64.5844003708168,
67.320155813866));
#216938=CARTESIAN_POINT('Ctrl Pts',(-36.3898142487375,65.1146479711371,
66.457880202735));
#216939=CARTESIAN_POINT('Ctrl Pts',(-36.3806431374805,65.3303077109132,
66.1424509966232));
#216940=CARTESIAN_POINT('Ctrl Pts',(-36.3531792325554,66.0185791796317,
65.2334495843888));
#216941=CARTESIAN_POINT('Ctrl Pts',(-36.3347698949052,66.5333448401378,
64.6742772282592));
#216942=CARTESIAN_POINT('Ctrl Pts',(-36.2980088765867,67.6540259236155,
63.6698862256385));
#216943=CARTESIAN_POINT('Ctrl Pts',(-36.280101406125,68.2559115284866,63.2252915191186));
#216944=CARTESIAN_POINT('Ctrl Pts',(-36.2423773112362,69.5916712184815,
62.4215255838452));
#216945=CARTESIAN_POINT('Ctrl Pts',(-36.2224209560955,70.3289509845132,
62.0754496513156));
#216946=CARTESIAN_POINT('Ctrl Pts',(-36.1841980023478,71.8123473356619,
61.5573109545676));
#216947=CARTESIAN_POINT('Ctrl Pts',(-36.1660256681261,72.5512763520278,
61.3765117920296));
#216948=CARTESIAN_POINT('Ctrl Pts',(-36.1346419626985,73.82391954092,61.1921293544449));
#216949=CARTESIAN_POINT('Ctrl Pts',(-36.1216763190792,74.3498884554293,
61.151473079505));
#216950=CARTESIAN_POINT('Ctrl Pts',(-36.0994659201618,75.2587981889374,
61.1420117351625));
#216951=CARTESIAN_POINT('Ctrl Pts',(-36.0902316936128,75.6407534126919,
61.1565248247328));
#216952=CARTESIAN_POINT('Ctrl Pts',(-36.0624859131522,76.7817823975121,
61.2553171806789));
#216953=CARTESIAN_POINT('Ctrl Pts',(-36.0438624321168,77.534077001011,61.3945401981191));
#216954=CARTESIAN_POINT('Ctrl Pts',(-36.0067408999156,78.9853669007069,
61.8112676918779));
#216955=CARTESIAN_POINT('Ctrl Pts',(-35.988694344898,79.6819222076254,62.0847621186578));
#216956=CARTESIAN_POINT('Ctrl Pts',(-35.9528381109727,80.9957693853785,
62.749953381127));
#216957=CARTESIAN_POINT('Ctrl Pts',(-35.9349493439011,81.6119380123203,
63.1367591984324));
#216958=CARTESIAN_POINT('Ctrl Pts',(-35.907678042527,82.4933009343184,63.8102467212397));
#216959=CARTESIAN_POINT('Ctrl Pts',(-35.8983499566447,82.7863426510017,
64.0575920235313));
#216960=CARTESIAN_POINT('Ctrl Pts',(-35.8614700593617,83.8961440396948,
65.0906122161347));
#216961=CARTESIAN_POINT('Ctrl Pts',(-35.8334895166668,84.6103459856919,
65.9775571670355));
#216962=CARTESIAN_POINT('Ctrl Pts',(-35.7964986090976,85.3813316779486,
67.2795294806806));
#216963=CARTESIAN_POINT('Ctrl Pts',(-35.7872658099445,85.5591885265115,
67.6158215934341));
#216964=CARTESIAN_POINT('Ctrl Pts',(-35.7597598446311,86.0375647481716,
68.6363994632009));
#216965=CARTESIAN_POINT('Ctrl Pts',(-35.7413319462033,86.2898632650145,
69.341193146973));
#216966=CARTESIAN_POINT('Ctrl Pts',(-35.7044264898673,86.6588103655716,
70.7909149069742));
#216967=CARTESIAN_POINT('Ctrl Pts',(-35.6863309381048,86.7742450080173,
71.5326880315955));
#216968=CARTESIAN_POINT('Ctrl Pts',(-35.648818522624,86.8653410612362,73.0604102750672));
#216969=CARTESIAN_POINT('Ctrl Pts',(-35.6293949578551,86.8345171836741,
73.8431304686555));
#216970=CARTESIAN_POINT('Ctrl Pts',(-35.5914248899701,86.6207960504798,
75.3788553687848));
#216971=CARTESIAN_POINT('Ctrl Pts',(-35.5728030752626,86.4408091712799,
76.1284841366248));
#216972=CARTESIAN_POINT('Ctrl Pts',(-35.5391741685667,85.9946680641214,
77.4183380945881));
#216973=CARTESIAN_POINT('Ctrl Pts',(-35.5243979477909,85.7577235077533,
77.9658340946686));
#216974=CARTESIAN_POINT('Ctrl Pts',(-35.5005313230928,85.3035724210339,
78.8299775913738));
#216975=CARTESIAN_POINT('Ctrl Pts',(-35.4912888580847,85.110428363515,79.1580595645729));
#216976=CARTESIAN_POINT('Ctrl Pts',(-35.4633045591508,84.4818599519238,
80.1168940152686));
#216977=CARTESIAN_POINT('Ctrl Pts',(-35.4443955308527,84.0007161641202,
80.7152502025691));
#216978=CARTESIAN_POINT('Ctrl Pts',(-35.4090375332272,82.9964579657966,
81.7422333759297));
#216979=CARTESIAN_POINT('Ctrl Pts',(-35.3928563160963,82.4878873656021,
82.1808725462551));
#216980=CARTESIAN_POINT('Ctrl Pts',(-35.3579265617688,81.3296222879418,
83.0197530690348));
#216981=CARTESIAN_POINT('Ctrl Pts',(-35.3391279751791,80.6728453803328,
83.405135571618));
#216982=CARTESIAN_POINT('Ctrl Pts',(-35.3033828774365,79.3481763536406,
84.0198277539064));
#216983=CARTESIAN_POINT('Ctrl Pts',(-35.2865212158438,78.6877362201186,
84.2577396147604));
#216984=CARTESIAN_POINT('Ctrl Pts',(-35.2510519203333,77.284704845737,84.626559331621));
#216985=CARTESIAN_POINT('Ctrl Pts',(-35.2325091256342,76.5427786576456,
84.7478897133586));
#216986=CARTESIAN_POINT('Ctrl Pts',(-35.1952623815698,75.0135616251408,
84.8507159279305));
#216987=CARTESIAN_POINT('Ctrl Pts',(-35.1763953294977,74.2294630684508,
84.8256751358169));
#216988=CARTESIAN_POINT('Ctrl Pts',(-35.1478966196537,73.0761780802292,
84.6737362045891));
#216989=CARTESIAN_POINT('Ctrl Pts',(-35.138539351106,72.7013848555789,84.6058415969981));
#216990=CARTESIAN_POINT('Ctrl Pts',(-35.1101296852693,71.5685208016559,
84.3436613971395));
#216991=CARTESIAN_POINT('Ctrl Pts',(-35.0914263267071,70.8258735601296,
84.0922397600767));
#216992=CARTESIAN_POINT('Ctrl Pts',(-35.054130075419,69.4309872081884,83.4601886701129));
#216993=CARTESIAN_POINT('Ctrl Pts',(-35.0356993205511,68.7794052416668,
83.0868580877431));
#216994=CARTESIAN_POINT('Ctrl Pts',(-34.9996002786209,67.560023159752,82.2252169376686));
#216995=CARTESIAN_POINT('Ctrl Pts',(-34.9817302608228,66.9943605823161,
81.7396804913581));
#216996=CARTESIAN_POINT('Ctrl Pts',(-34.9543056214923,66.2138359483376,
80.9303940226674));
#216997=CARTESIAN_POINT('Ctrl Pts',(-34.9449898578565,65.9630283097317,
80.643917330957));
#216998=CARTESIAN_POINT('Ctrl Pts',(-34.907689131715,65.0106648544754,79.4440609710513));
#216999=CARTESIAN_POINT('Ctrl Pts',(-34.8802940945988,64.4302316129435,
78.4426538658593));
#217000=CARTESIAN_POINT('Ctrl Pts',(-34.8428433081152,63.8613744289818,
77.017131525699));
#217001=CARTESIAN_POINT('Ctrl Pts',(-34.8335088458404,63.7366295916944,
76.6542583158344));
#217002=CARTESIAN_POINT('Ctrl Pts',(-34.8068931854123,63.4289538650965,
75.5944183497892));
#217003=CARTESIAN_POINT('Ctrl Pts',(-34.7896486514922,63.2917027200569,
74.8859911727886));
#217004=CARTESIAN_POINT('Ctrl Pts',(-34.7539743461902,63.1449742572066,
73.4265644299001));
#217005=CARTESIAN_POINT('Ctrl Pts',(-34.7357712603519,63.14072784864,72.6782228425266));
#217006=CARTESIAN_POINT('Ctrl Pts',(-34.6994034392337,63.2748858221362,
71.1723406594849));
#217007=CARTESIAN_POINT('Ctrl Pts',(-34.6809565209563,63.4165059879159,
70.418575997231));
#217008=CARTESIAN_POINT('Ctrl Pts',(-34.6529840677361,63.736348649039,69.3170045548025));
#217009=CARTESIAN_POINT('Ctrl Pts',(-34.6436639930778,63.8605228427577,
68.9556065871905));
#217010=CARTESIAN_POINT('Ctrl Pts',(-34.633246674525,64.0201624213107,68.5551452692357));
#217011=CARTESIAN_POINT('Ctrl Pts',(-34.6320592341848,64.0386618588475,
68.5095667720041));
#217012=CARTESIAN_POINT('Ctrl Pts',(-34.6308727569695,64.0574429702493,
68.4641091421755));
#217013=CARTESIAN_POINT('Origin',(-33.5526503323277,75.000050506625,72.9851176492631));
#217014=CARTESIAN_POINT('',(-32.5154663289944,64.0574429734778,68.4641091343612));
#217015=CARTESIAN_POINT('',(-32.8170317113719,64.0574429575879,68.464109172821));
#217016=CARTESIAN_POINT('',(-33.5526503323277,64.0574429649796,68.4641091549303));
#217017=CARTESIAN_POINT('Ctrl Pts',(-32.5154663295374,64.0574429734829,
68.464109134349));
#217018=CARTESIAN_POINT('Ctrl Pts',(-32.5181729121248,64.0151117273703,
68.5665672940872));
#217019=CARTESIAN_POINT('Ctrl Pts',(-32.5208831491634,63.9742087564226,
68.6696459656842));
#217020=CARTESIAN_POINT('Ctrl Pts',(-32.5365378811924,63.7466884692259,
69.2673902923806));
#217021=CARTESIAN_POINT('Ctrl Pts',(-32.549578617579,63.5919310328918,69.773504390183));
#217022=CARTESIAN_POINT('Ctrl Pts',(-32.579679363895,63.3144198391241,70.9598095435459));
#217023=CARTESIAN_POINT('Ctrl Pts',(-32.5964491857621,63.2163023712604,
71.6438046500751));
#217024=CARTESIAN_POINT('Ctrl Pts',(-32.631509007593,63.1371761708274,73.0769936812608));
#217025=CARTESIAN_POINT('Ctrl Pts',(-32.6499211125506,63.1665014507285,
73.8237672795319));
#217026=CARTESIAN_POINT('Ctrl Pts',(-32.6868111493593,63.3657179440685,
75.3054641047265));
#217027=CARTESIAN_POINT('Ctrl Pts',(-32.704912584929,63.5358507142816,76.0369737902692));
#217028=CARTESIAN_POINT('Ctrl Pts',(-32.7424335552352,64.0223432761175,
77.4885615806854));
#217029=CARTESIAN_POINT('Ctrl Pts',(-32.7618527034778,64.3434846941796,
78.2032273020582));
#217030=CARTESIAN_POINT('Ctrl Pts',(-32.7902853281375,64.9222311547592,
79.2110793253665));
#217031=CARTESIAN_POINT('Ctrl Pts',(-32.7995280327456,65.1275708077361,
79.5318104969169));
#217032=CARTESIAN_POINT('Ctrl Pts',(-32.8270447993044,65.7808975055577,
80.4514493787191));
#217033=CARTESIAN_POINT('Ctrl Pts',(-32.8454615668622,66.2705269994198,
81.0184419426092));
#217034=CARTESIAN_POINT('Ctrl Pts',(-32.8823126578241,67.3507853437362,
82.0531381278404));
#217035=CARTESIAN_POINT('Ctrl Pts',(-32.9003564060052,67.9391100175202,
82.5183948234867));
#217036=CARTESIAN_POINT('Ctrl Pts',(-32.937754045335,69.2239768130503,83.3499035028791));
#217037=CARTESIAN_POINT('Ctrl Pts',(-32.9571254053667,69.9210371542342,
83.7087100909432));
#217038=CARTESIAN_POINT('Ctrl Pts',(-32.9854965318043,71.0025491703065,
84.1361355379897));
#217039=CARTESIAN_POINT('Ctrl Pts',(-32.9947127388147,71.3632804886609,
84.2589422831795));
#217040=CARTESIAN_POINT('Ctrl Pts',(-33.0229841396186,72.4814353237562,
84.5803407223701));
#217041=CARTESIAN_POINT('Ctrl Pts',(-33.0421997928277,73.2531524578813,
84.7214268900956));
#217042=CARTESIAN_POINT('Ctrl Pts',(-33.079761918093,74.7797659180713,84.8465205931168));
#217043=CARTESIAN_POINT('Ctrl Pts',(-33.097734005379,75.530535854426,84.8366994644064));
#217044=CARTESIAN_POINT('Ctrl Pts',(-33.1350187928347,77.0532501055069,
84.671725927166));
#217045=CARTESIAN_POINT('Ctrl Pts',(-33.1543180996902,77.8209021711521,
84.5105347740466));
#217046=CARTESIAN_POINT('Ctrl Pts',(-33.1825366520723,78.9298947516434,
84.1601488792891));
#217047=CARTESIAN_POINT('Ctrl Pts',(-33.1917039029207,79.2870294189683,
84.0280706730773));
#217048=CARTESIAN_POINT('Ctrl Pts',(-33.2189310943116,80.3222906557612,
83.5873983550509));
#217049=CARTESIAN_POINT('Ctrl Pts',(-33.2371330852797,80.9783622071833,
83.2317939049514));
#217050=CARTESIAN_POINT('Ctrl Pts',(-33.2735865072273,82.2177414112091,
82.4002377705987));
#217051=CARTESIAN_POINT('Ctrl Pts',(-33.2914584980292,82.7979302921072,
81.9256221588403));
#217052=CARTESIAN_POINT('Ctrl Pts',(-33.3285584788554,83.8859759922063,
80.8485587565301));
#217053=CARTESIAN_POINT('Ctrl Pts',(-33.3477954987094,84.3864667553391,
80.2438067442845));
#217054=CARTESIAN_POINT('Ctrl Pts',(-33.375940413939,85.0360006307987,79.2783442208956));
#217055=CARTESIAN_POINT('Ctrl Pts',(-33.385074286717,85.2330777568063,78.9525417070216));
#217056=CARTESIAN_POINT('Ctrl Pts',(-33.4131447479665,85.7869973736596,
77.9284216256599));
#217057=CARTESIAN_POINT('Ctrl Pts',(-33.4322515290968,86.0904964452474,
77.2037041466068));
#217058=CARTESIAN_POINT('Ctrl Pts',(-33.4695410162937,86.5393933668118,
75.7389505218033));
#217059=CARTESIAN_POINT('Ctrl Pts',(-33.487364085763,86.6903275967785,75.0043876740146));
#217060=CARTESIAN_POINT('Ctrl Pts',(-33.5224532382719,86.8465419363969,
73.5626496562674));
#217061=CARTESIAN_POINT('Ctrl Pts',(-33.5396495134092,86.8599451966265,
72.8594514775075));
#217062=CARTESIAN_POINT('Ctrl Pts',(-33.565887804923,86.7843782309649,71.778784663845));
#217063=CARTESIAN_POINT('Ctrl Pts',(-33.5750332280944,86.73940968495,71.3998521049431));
#217064=CARTESIAN_POINT('Ctrl Pts',(-33.6083582939631,86.5100341266544,
70.0343597228469));
#217065=CARTESIAN_POINT('Ctrl Pts',(-33.6329069538302,86.2187538866895,
69.0700985762561));
#217066=CARTESIAN_POINT('Ctrl Pts',(-33.6663560913667,85.6542549138643,
67.8070208840266));
#217067=CARTESIAN_POINT('Ctrl Pts',(-33.6754781943835,85.4824747305474,
67.4675510614521));
#217068=CARTESIAN_POINT('Ctrl Pts',(-33.7059599048676,84.8577672717057,
66.3678727109917));
#217069=CARTESIAN_POINT('Ctrl Pts',(-33.7275935580915,84.3360734543789,
65.6501900329925));
#217070=CARTESIAN_POINT('Ctrl Pts',(-33.7583452584903,83.4819053646819,
64.7156600258739));
#217071=CARTESIAN_POINT('Ctrl Pts',(-33.7675165202791,83.2109939507754,
64.4466049123596));
#217072=CARTESIAN_POINT('Ctrl Pts',(-33.7949968365743,82.3644640973078,
63.6834863394994));
#217073=CARTESIAN_POINT('Ctrl Pts',(-33.8134263206609,81.753910678644,63.231129058799));
#217074=CARTESIAN_POINT('Ctrl Pts',(-33.8502170881033,80.4648078685701,
62.4554617362716));
#217075=CARTESIAN_POINT('Ctrl Pts',(-33.8681357565689,79.7903400725302,
62.1319911260003));
#217076=CARTESIAN_POINT('Ctrl Pts',(-33.9059310831589,78.3266623695969,
61.5932198606606));
#217077=CARTESIAN_POINT('Ctrl Pts',(-33.9259438579676,77.5364847044871,
61.3916640367638));
#217078=CARTESIAN_POINT('Ctrl Pts',(-33.9642674962904,75.9797414048656,
61.1614753622317));
#217079=CARTESIAN_POINT('Ctrl Pts',(-33.9825032037852,75.2186007557229,
61.1229696714893));
#217080=CARTESIAN_POINT('Ctrl Pts',(-34.0173183225318,73.7958921329189,
61.1880475000727));
#217081=CARTESIAN_POINT('Ctrl Pts',(-34.0337048314021,73.1364687683759,
61.2741002085176));
#217082=CARTESIAN_POINT('Ctrl Pts',(-34.0590875503143,72.1166259704857,
61.4955458017704));
#217083=CARTESIAN_POINT('Ctrl Pts',(-34.0682707776253,71.7496017886559,
61.5939376434187));
#217084=CARTESIAN_POINT('Ctrl Pts',(-34.0991154901616,70.5413725129401,
61.9810002693125));
#217085=CARTESIAN_POINT('Ctrl Pts',(-34.1210858444369,69.7280402850099,
62.3466826066562));
#217086=CARTESIAN_POINT('Ctrl Pts',(-34.1615021363173,68.305357747163,63.1899008655832));
#217087=CARTESIAN_POINT('Ctrl Pts',(-34.1799418633589,67.6867226182865,
63.642718364941));
#217088=CARTESIAN_POINT('Ctrl Pts',(-34.2080746303714,66.8322966292095,
64.4053344248759));
#217089=CARTESIAN_POINT('Ctrl Pts',(-34.2174662619616,66.5608694509396,
64.6721695712479));
#217090=CARTESIAN_POINT('Ctrl Pts',(-34.2452567103186,65.7957700539853,
65.5004862202017));
#217091=CARTESIAN_POINT('Ctrl Pts',(-34.2633034374738,65.3418771370186,
66.0961282641829));
#217092=CARTESIAN_POINT('Ctrl Pts',(-34.2975051576547,64.6033398053979,
67.2831729386068));
#217093=CARTESIAN_POINT('Ctrl Pts',(-34.313594856828,64.3057936841928,67.8630033493468));
#217094=CARTESIAN_POINT('Ctrl Pts',(-34.329622639475,64.0574429649796,68.4641091549303));
#217095=CARTESIAN_POINT('Ctrl Pts',(-34.6308727569695,64.0574429702493,
68.4641091421755));
#217096=CARTESIAN_POINT('Ctrl Pts',(-34.6193506401723,64.2398300876496,
68.0226610355699));
#217097=CARTESIAN_POINT('Ctrl Pts',(-34.6079014722085,64.4487809430319,
67.592612006747));
#217098=CARTESIAN_POINT('Ctrl Pts',(-34.5779305593184,65.0568883265986,
66.5125636986354));
#217099=CARTESIAN_POINT('Ctrl Pts',(-34.5592481834225,65.4937954843009,
65.8864181927348));
#217100=CARTESIAN_POINT('Ctrl Pts',(-34.5206541293554,66.5263201696141,
64.6745489590068));
#217101=CARTESIAN_POINT('Ctrl Pts',(-34.5008291531671,67.1298312075825,
64.1009004570284));
#217102=CARTESIAN_POINT('Ctrl Pts',(-34.4623803983329,68.3806459718267,
63.1402533099441));
#217103=CARTESIAN_POINT('Ctrl Pts',(-34.4441274855894,69.0146291071383,
62.7424319607719));
#217104=CARTESIAN_POINT('Ctrl Pts',(-34.4076471356524,70.3649460481053,
62.0635538342914));
#217105=CARTESIAN_POINT('Ctrl Pts',(-34.3891373124602,71.0797066814955,
61.7870979475709));
#217106=CARTESIAN_POINT('Ctrl Pts',(-34.361049697777,72.1841649839589,61.4787284976003));
#217107=CARTESIAN_POINT('Ctrl Pts',(-34.3516820901783,72.5569814841759,
61.3938442480434));
#217108=CARTESIAN_POINT('Ctrl Pts',(-34.3290750741486,73.4737978033568,
61.2313052386171));
#217109=CARTESIAN_POINT('Ctrl Pts',(-34.3158686666609,74.0203569113405,
61.1731848870587));
#217110=CARTESIAN_POINT('Ctrl Pts',(-34.2834734697624,75.3509926791057,
61.1247050893187));
#217111=CARTESIAN_POINT('Ctrl Pts',(-34.2641519258276,76.1339124276137,
61.1738137005168));
#217112=CARTESIAN_POINT('Ctrl Pts',(-34.2320953030451,77.4337737282657,
61.3858563006051));
#217113=CARTESIAN_POINT('Ctrl Pts',(-34.2192063958203,77.9548729189376,
61.5075352063339));
#217114=CARTESIAN_POINT('Ctrl Pts',(-34.1877149343325,79.1903685337703,
61.8857772318997));
#217115=CARTESIAN_POINT('Ctrl Pts',(-34.1689842424272,79.8918123264443,
62.1765664425843));
#217116=CARTESIAN_POINT('Ctrl Pts',(-34.1298563763896,81.3052055716951,
62.9284557091413));
#217117=CARTESIAN_POINT('Ctrl Pts',(-34.1095450191903,82.0053176642944,
63.4029638858185));
#217118=CARTESIAN_POINT('Ctrl Pts',(-34.0794691806072,82.9387301685167,
64.1929868762098));
#217119=CARTESIAN_POINT('Ctrl Pts',(-34.0700949349339,83.2164475033996,
64.4519460101014));
#217120=CARTESIAN_POINT('Ctrl Pts',(-34.0432571153324,83.9776754969654,
65.2334338957908));
#217121=CARTESIAN_POINT('Ctrl Pts',(-34.0260979218382,84.4271560318671,
65.7867821930574));
#217122=CARTESIAN_POINT('Ctrl Pts',(-33.9902141916365,85.2453578099986,
67.0032125914499));
#217123=CARTESIAN_POINT('Ctrl Pts',(-33.971485421099,85.6056659337077,67.6681236254943));
#217124=CARTESIAN_POINT('Ctrl Pts',(-33.9310885358196,86.2493577911117,
69.1860501125651));
#217125=CARTESIAN_POINT('Ctrl Pts',(-33.9094673704172,86.504082512686,70.0462259006034));
#217126=CARTESIAN_POINT('Ctrl Pts',(-33.8779950886871,86.7257156345537,
71.3017110821659));
#217127=CARTESIAN_POINT('Ctrl Pts',(-33.868568337302,86.7737742760017,71.6795491385107));
#217128=CARTESIAN_POINT('Ctrl Pts',(-33.8399302810624,86.8648663597095,
72.840585655259));
#217129=CARTESIAN_POINT('Ctrl Pts',(-33.8210113908767,86.8484111579152,
73.6262878470836));
#217130=CARTESIAN_POINT('Ctrl Pts',(-33.7833517897833,86.6648866794568,
75.1460293063073));
#217131=CARTESIAN_POINT('Ctrl Pts',(-33.7648218705852,86.505394820169,75.877349237697));
#217132=CARTESIAN_POINT('Ctrl Pts',(-33.7373298193746,86.1625685956945,
76.9502656360633));
#217133=CARTESIAN_POINT('Ctrl Pts',(-33.7281000292353,86.029741952418,77.3060105257016));
#217134=CARTESIAN_POINT('Ctrl Pts',(-33.7002071108271,85.5799844689137,
78.3539206464976));
#217135=CARTESIAN_POINT('Ctrl Pts',(-33.6813557955547,85.2132155957022,
79.0225255863));
#217136=CARTESIAN_POINT('Ctrl Pts',(-33.6434139597103,84.3437376786615,
80.298767790114));
#217137=CARTESIAN_POINT('Ctrl Pts',(-33.6245326779248,83.839452988894,80.9008574845915));
#217138=CARTESIAN_POINT('Ctrl Pts',(-33.5869398969987,82.7451952932646,
81.9712951127391));
#217139=CARTESIAN_POINT('Ctrl Pts',(-33.5684366827239,82.1627019208074,
82.4421302754121));
#217140=CARTESIAN_POINT('Ctrl Pts',(-33.5410082140205,81.2235877113892,
83.0643827435643));
#217141=CARTESIAN_POINT('Ctrl Pts',(-33.5318099532505,80.8975668381295,
83.2585446022429));
#217142=CARTESIAN_POINT('Ctrl Pts',(-33.5039667727631,79.8898322658712,
83.7948991041462));
#217143=CARTESIAN_POINT('Ctrl Pts',(-33.4851369145628,79.1838554156084,
84.0872392962354));
#217144=CARTESIAN_POINT('Ctrl Pts',(-33.4473067828707,77.7059728835576,
84.5380790248095));
#217145=CARTESIAN_POINT('Ctrl Pts',(-33.428512547838,76.9364408575445,84.6916683920248));
#217146=CARTESIAN_POINT('Ctrl Pts',(-33.3910778521779,75.413418711161,84.8412617073136));
#217147=CARTESIAN_POINT('Ctrl Pts',(-33.3726448406043,74.6641832111248,
84.8437106768532));
#217148=CARTESIAN_POINT('Ctrl Pts',(-33.3453309286786,73.5421528483799,
84.7409024508214));
#217149=CARTESIAN_POINT('Ctrl Pts',(-33.3361748620735,73.1664518874494,
84.6881881036387));
#217150=CARTESIAN_POINT('Ctrl Pts',(-33.3084116471317,72.0431375258176,
84.4751484011607));
#217151=CARTESIAN_POINT('Ctrl Pts',(-33.2896188289009,71.3078971471474,
84.260406225023));
#217152=CARTESIAN_POINT('Ctrl Pts',(-33.2519364919601,69.8724979234016,
83.6855842913801));
#217153=CARTESIAN_POINT('Ctrl Pts',(-33.2332449359375,69.1770860225593,
83.3236316694871));
#217154=CARTESIAN_POINT('Ctrl Pts',(-33.1959911246191,67.8966503931203,
82.4867395801037));
#217155=CARTESIAN_POINT('Ctrl Pts',(-33.1776373622461,67.3109885926469,
82.0193552701121));
#217156=CARTESIAN_POINT('Ctrl Pts',(-33.1504329688181,66.5004660851745,
81.236250341451));
#217157=CARTESIAN_POINT('Ctrl Pts',(-33.1413090959226,66.2404403303855,
80.9596618765858));
#217158=CARTESIAN_POINT('Ctrl Pts',(-33.1136152048845,65.4970972074817,
80.088659777109));
#217159=CARTESIAN_POINT('Ctrl Pts',(-33.0948548834083,65.0577201636671,
79.4594119749617));
#217160=CARTESIAN_POINT('Ctrl Pts',(-33.05728867943,64.2988546805018,78.1110729050898));
#217161=CARTESIAN_POINT('Ctrl Pts',(-33.0386700448582,63.9839043482313,
77.3936932620491));
#217162=CARTESIAN_POINT('Ctrl Pts',(-33.0015376640987,63.5105141099323,
75.939701665667));
#217163=CARTESIAN_POINT('Ctrl Pts',(-32.9832353344142,63.3469230480352,
75.2085481391496));
#217164=CARTESIAN_POINT('Ctrl Pts',(-32.9560847934007,63.2058233670797,
74.0899686808031));
#217165=CARTESIAN_POINT('Ctrl Pts',(-32.9469683983006,63.1764477566845,
73.7110016473863));
#217166=CARTESIAN_POINT('Ctrl Pts',(-32.9193010016226,63.1429395431197,
72.5654118244789));
#217167=CARTESIAN_POINT('Ctrl Pts',(-32.9005529512463,63.19493406089,71.7991808816112));
#217168=CARTESIAN_POINT('Ctrl Pts',(-32.8630215230713,63.4487474520803,
70.2725148116573));
#217169=CARTESIAN_POINT('Ctrl Pts',(-32.8444150532531,63.65290510332,69.5162398468281));
#217170=CARTESIAN_POINT('Ctrl Pts',(-32.8226405863238,63.9709778019663,
68.6777948318023));
#217171=CARTESIAN_POINT('Ctrl Pts',(-32.8198374151532,64.0134385958395,
68.5706169273563));
#217172=CARTESIAN_POINT('Ctrl Pts',(-32.8170317109009,64.0574429575835,
68.4641091728316));
#217173=CARTESIAN_POINT('Origin',(-64.067537349647,66.6819786653733,69.5522455184007));
#217174=CARTESIAN_POINT('',(-63.567539947994,57.2086765902407,65.6382900020344));
#217175=CARTESIAN_POINT('',(-64.083662457183,57.6856885892254,65.8353741883268));
#217176=CARTESIAN_POINT('',(-64.067537349647,57.6707866405467,65.8292137334027));
#217177=CARTESIAN_POINT('',(-63.5675399484425,56.5589377686512,71.1605188170944));
#217178=CARTESIAN_POINT('Origin',(-63.5675399484425,66.6819786653733,69.5522455184007));
#217179=CARTESIAN_POINT('',(-63.5676514812564,56.5602242475556,71.1683725272604));
#217180=CARTESIAN_POINT('Ctrl Pts',(-63.5675399484425,56.5589377686512,
71.1605188170944));
#217181=CARTESIAN_POINT('Ctrl Pts',(-63.5675771260471,56.5593540010166,
71.1631387308002));
#217182=CARTESIAN_POINT('Ctrl Pts',(-63.5676143036518,56.5597712504601,
71.1657584829202));
#217183=CARTESIAN_POINT('Ctrl Pts',(-63.5676514812564,56.5601895168558,
71.1683780726648));
#217184=CARTESIAN_POINT('',(-64.0597104235077,75.7004037793539,73.2782678282931));
#217185=CARTESIAN_POINT('Ctrl Pts',(-64.0597104235077,75.7004037793539,
73.2782678282931));
#217186=CARTESIAN_POINT('Ctrl Pts',(-64.0451218652925,75.4260421514271,
73.9805348271195));
#217187=CARTESIAN_POINT('Ctrl Pts',(-64.0303356772116,75.0709760863526,
74.649533020937));
#217188=CARTESIAN_POINT('Ctrl Pts',(-64.0010809330892,74.2154841558898,
75.8907572272977));
#217189=CARTESIAN_POINT('Ctrl Pts',(-63.986792125037,73.7171648123145,76.4599526620535));
#217190=CARTESIAN_POINT('Ctrl Pts',(-63.9624118992683,72.784481500054,77.3072526411669));
#217191=CARTESIAN_POINT('Ctrl Pts',(-63.9525239575833,72.383059953084,77.6190644691922));
#217192=CARTESIAN_POINT('Ctrl Pts',(-63.9304794831545,71.4249343683092,
78.2509947667965));
#217193=CARTESIAN_POINT('Ctrl Pts',(-63.9183841578928,70.8568051209136,
78.5508027796505));
#217194=CARTESIAN_POINT('Ctrl Pts',(-63.8936864137596,69.6653511567733,
79.0391399714275));
#217195=CARTESIAN_POINT('Ctrl Pts',(-63.88113511846,69.0430516921984,79.225797709248));
#217196=CARTESIAN_POINT('Ctrl Pts',(-63.856575596689,67.7745311760812,79.4740442805028));
#217197=CARTESIAN_POINT('Ctrl Pts',(-63.8444614159778,67.1311833028043,
79.5360061975211));
#217198=CARTESIAN_POINT('Ctrl Pts',(-63.8259893536362,66.1629495894997,
79.5355609346259));
#217199=CARTESIAN_POINT('Ctrl Pts',(-63.8197844751296,65.8391438196649,
79.5196743975064));
#217200=CARTESIAN_POINT('Ctrl Pts',(-63.8012616880293,64.8742259690284,
79.4251632815208));
#217201=CARTESIAN_POINT('Ctrl Pts',(-63.7892155220506,64.2400125908015,
79.3000344343668));
#217202=CARTESIAN_POINT('Ctrl Pts',(-63.7646866488347,62.9915820917864,
78.9263816821826));
#217203=CARTESIAN_POINT('Ctrl Pts',(-63.7521500622743,62.3801658963736,
78.6758456951229));
#217204=CARTESIAN_POINT('Ctrl Pts',(-63.7273750610242,61.2237694438128,
78.0635093820407));
#217205=CARTESIAN_POINT('Ctrl Pts',(-63.7153700975349,60.680608334847,77.7044378425474));
#217206=CARTESIAN_POINT('Ctrl Pts',(-63.6918930293161,59.7055417620587,
76.9159481552167));
#217207=CARTESIAN_POINT('Ctrl Pts',(-63.6804420652402,59.2696957205743,
76.4937784653886));
#217208=CARTESIAN_POINT('Ctrl Pts',(-63.6520134359374,58.2816372967606,
75.3484072926961));
#217209=CARTESIAN_POINT('Ctrl Pts',(-63.6354546893578,57.784018645059,74.5842894596792));
#217210=CARTESIAN_POINT('Ctrl Pts',(-63.6099369967653,57.1974075459963,
73.353242818012));
#217211=CARTESIAN_POINT('Ctrl Pts',(-63.6013230942664,57.0283706254766,
72.9269478107908));
#217212=CARTESIAN_POINT('Ctrl Pts',(-63.5843894744831,56.7499095059732,
72.0578394046303));
#217213=CARTESIAN_POINT('Ctrl Pts',(-63.5760671502839,56.6402828854334,
71.6159185090166));
#217214=CARTESIAN_POINT('Ctrl Pts',(-63.5676866568907,56.560334274244,71.1683542085754));
#217215=CARTESIAN_POINT('',(-64.5675364832709,60.6333031659922,62.5539864962095));
#217216=CARTESIAN_POINT('Ctrl Pts',(-64.56753648372,60.6339090599576,62.5534304824221));
#217217=CARTESIAN_POINT('Ctrl Pts',(-64.5559053154294,61.0571436471093,
62.1723173071139));
#217218=CARTESIAN_POINT('Ctrl Pts',(-64.5443683788522,61.5150569575824,
61.8309194745767));
#217219=CARTESIAN_POINT('Ctrl Pts',(-64.5208921017017,62.4915898340133,
61.2336544858132));
#217220=CARTESIAN_POINT('Ctrl Pts',(-64.5090141235672,63.0095718878263,
60.9793895503546));
#217221=CARTESIAN_POINT('Ctrl Pts',(-64.4895980530763,63.9049898999737,
60.6390797274406));
#217222=CARTESIAN_POINT('Ctrl Pts',(-64.4819115658727,64.2699923360781,
60.5255089913027));
#217223=CARTESIAN_POINT('Ctrl Pts',(-64.4637503035837,65.1405602157676,
60.3120024769304));
#217224=CARTESIAN_POINT('Ctrl Pts',(-64.4532397072825,65.6498952088197,
60.2307861428219));
#217225=CARTESIAN_POINT('Ctrl Pts',(-64.430296409186,66.7729171495099,60.1455432302508));
#217226=CARTESIAN_POINT('Ctrl Pts',(-64.4181229662858,67.3853348297619,
60.1593209414688));
#217227=CARTESIAN_POINT('Ctrl Pts',(-64.393582019433,68.597723769527,60.3048983612714));
#217228=CARTESIAN_POINT('Ctrl Pts',(-64.3811840907539,69.1958603364025,
60.4364493233302));
#217229=CARTESIAN_POINT('Ctrl Pts',(-64.3626497400445,70.0696915604235,
60.7197347739203));
#217230=CARTESIAN_POINT('Ctrl Pts',(-64.3565059984246,70.3577414698788,
60.8290195178738));
#217231=CARTESIAN_POINT('Ctrl Pts',(-64.3381789619652,71.2014014411427,
61.1971140003167));
#217232=CARTESIAN_POINT('Ctrl Pts',(-64.3259769456409,71.7382300434053,
61.496240439733));
#217233=CARTESIAN_POINT('Ctrl Pts',(-64.3074536245922,72.4961532874526,
62.0201534087073));
#217234=CARTESIAN_POINT('Ctrl Pts',(-64.3012371111907,72.7414996271467,
62.2080285592825));
#217235=CARTESIAN_POINT('Ctrl Pts',(-64.2828087450528,73.4462001197079,
62.8043768560141));
#217236=CARTESIAN_POINT('Ctrl Pts',(-64.2707866092118,73.8757217919052,
63.246099592049));
#217237=CARTESIAN_POINT('Ctrl Pts',(-64.2461815857642,74.6502677961469,
64.2130030553011));
#217238=CARTESIAN_POINT('Ctrl Pts',(-64.2336243377818,74.9927420587892,
64.7383397323999));
#217239=CARTESIAN_POINT('Ctrl Pts',(-64.2090209000687,75.5679416527631,
65.8442881461347));
#217240=CARTESIAN_POINT('Ctrl Pts',(-64.1969313758394,75.8004090675362,
66.4223889606875));
#217241=CARTESIAN_POINT('Ctrl Pts',(-64.1741708575269,76.1254665991152,
67.5280676131162));
#217242=CARTESIAN_POINT('Ctrl Pts',(-64.1635849873021,76.2330829292957,
68.0497086663742));
#217243=CARTESIAN_POINT('Ctrl Pts',(-64.1375350595926,76.3928321250279,
69.3669952652942));
#217244=CARTESIAN_POINT('Ctrl Pts',(-64.1221954863727,76.3904768158639,
70.1665095515024));
#217245=CARTESIAN_POINT('Ctrl Pts',(-64.0986553233582,76.24076456436,71.3543811017856));
#217246=CARTESIAN_POINT('Ctrl Pts',(-64.0907263636134,76.1658342115345,
71.7497160050923));
#217247=CARTESIAN_POINT('Ctrl Pts',(-64.0751169343179,75.9680327516169,
72.5260089561059));
#217248=CARTESIAN_POINT('Ctrl Pts',(-64.0674339216932,75.8456567580364,
72.9064724931336));
#217249=CARTESIAN_POINT('Ctrl Pts',(-64.0597104235077,75.7004037793539,
73.2782678282931));
#217250=CARTESIAN_POINT('',(-64.5675364836265,58.2049936507084,73.253721483482));
#217251=CARTESIAN_POINT('Origin',(-64.5675364832709,66.6819786653733,69.5522455184007));
#217252=CARTESIAN_POINT('Ctrl Pts',(-64.567536483719,58.2048719639793,73.2537614015209));
#217253=CARTESIAN_POINT('Ctrl Pts',(-64.5522519075793,58.0976217008117,
73.0463357077704));
#217254=CARTESIAN_POINT('Ctrl Pts',(-64.5369913991239,57.9980049358009,
72.8343190083415));
#217255=CARTESIAN_POINT('Ctrl Pts',(-64.521750391934,57.9063835252547,72.6182897831504));
#217256=CARTESIAN_POINT('Ctrl Pts',(-64.5065149014817,57.8147952786109,
72.4023387533513));
#217257=CARTESIAN_POINT('Ctrl Pts',(-64.4912988981798,57.731196741534,72.1823783236064));
#217258=CARTESIAN_POINT('Ctrl Pts',(-64.4760978205663,57.6559053051787,
71.9590140988971));
#217259=CARTESIAN_POINT('Ctrl Pts',(-64.4609038574466,57.5806491071448,
71.7357544143683));
#217260=CARTESIAN_POINT('Ctrl Pts',(-64.4457248060474,57.5136923598297,
71.5090943516252));
#217261=CARTESIAN_POINT('Ctrl Pts',(-64.4305561113083,57.4553059750096,
71.279663000753));
#217262=CARTESIAN_POINT('Ctrl Pts',(-64.4153929780724,57.3969409971777,
71.0503157693929));
#217263=CARTESIAN_POINT('Ctrl Pts',(-64.4002401939036,57.3471402054655,
70.8181995207373));
#217264=CARTESIAN_POINT('Ctrl Pts',(-64.38509320875,57.306126469134,70.5839634489254));
#217265=CARTESIAN_POINT('Ctrl Pts',(-64.369953184099,57.265131579868,70.3498350157477));
#217266=CARTESIAN_POINT('Ctrl Pts',(-64.3548189531347,57.23291575996,70.113588953228));
#217267=CARTESIAN_POINT('Ctrl Pts',(-64.3396859720749,57.2096524013204,
69.8758907034779));
#217268=CARTESIAN_POINT('Ctrl Pts',(-64.334832339477,57.2021910957531,69.799653247758));
#217269=CARTESIAN_POINT('Ctrl Pts',(-64.3299788354556,57.1956503379729,
69.7232665234063));
#217270=CARTESIAN_POINT('Ctrl Pts',(-64.3251253100958,57.190034755535,69.6467527948062));
#217271=CARTESIAN_POINT('Ctrl Pts',(-64.3100488689152,57.1725911466023,
69.4090792187472));
#217272=CARTESIAN_POINT('Ctrl Pts',(-64.2949725167308,57.1640786946212,
69.17018381911));
#217273=CARTESIAN_POINT('Ctrl Pts',(-64.2798981906767,57.1646082439414,
68.9307425222474));
#217274=CARTESIAN_POINT('Ctrl Pts',(-64.2648429722312,57.1651371220262,
68.6916047315291));
#217275=CARTESIAN_POINT('Ctrl Pts',(-64.2497897747828,57.1746851526237,
68.4519226836776));
#217276=CARTESIAN_POINT('Ctrl Pts',(-64.2347405281089,57.1933117377907,
68.2123797226737));
#217277=CARTESIAN_POINT('Ctrl Pts',(-64.2197180065408,57.211905245059,67.973262152462));
#217278=CARTESIAN_POINT('Ctrl Pts',(-64.2046994217278,57.2395451263782,
67.7342834363986));
#217279=CARTESIAN_POINT('Ctrl Pts',(-64.1896866931843,57.2762388962374,
67.4961293606103));
#217280=CARTESIAN_POINT('Ctrl Pts',(-64.1746906332512,57.3128919250582,
67.2582397069403));
#217281=CARTESIAN_POINT('Ctrl Pts',(-64.1597004165905,57.3585787693851,
67.0211731258154));
#217282=CARTESIAN_POINT('Ctrl Pts',(-64.1447179563303,57.4132549887369,
66.7856152711256));
#217283=CARTESIAN_POINT('Ctrl Pts',(-64.1297582205198,57.4678482786516,
66.5504146957163));
#217284=CARTESIAN_POINT('Ctrl Pts',(-64.1148062175988,57.5314036925399,
66.3167185364823));
#217285=CARTESIAN_POINT('Ctrl Pts',(-64.0998638520033,57.6038250600662,
66.0852075409195));
#217286=CARTESIAN_POINT('Ctrl Pts',(-64.0944699454783,57.629967780531,66.0016365252333));
#217287=CARTESIAN_POINT('Ctrl Pts',(-64.0890772947654,57.6572653071481,
65.9183502156667));
#217288=CARTESIAN_POINT('Ctrl Pts',(-64.0836859894461,57.6857114539578,
65.8353804738359));
#217289=CARTESIAN_POINT('Origin',(-64.067537349647,66.6819786653733,69.5522455184007));
#217290=CARTESIAN_POINT('',(-63.567539947994,63.4350769493012,59.8300991896842));
#217291=CARTESIAN_POINT('Ctrl Pts',(-64.0833825702184,57.6854166417086,
65.8352994300243));
#217292=CARTESIAN_POINT('Ctrl Pts',(-64.0619309619701,57.7965027550469,
65.510245884164));
#217293=CARTESIAN_POINT('Ctrl Pts',(-64.0405438036779,57.9246131816582,
65.1915387606867));
#217294=CARTESIAN_POINT('Ctrl Pts',(-63.9975780848989,58.2183872019184,
64.5599055048844));
#217295=CARTESIAN_POINT('Ctrl Pts',(-63.9760783705587,58.3845348618842,
64.2483770552226));
#217296=CARTESIAN_POINT('Ctrl Pts',(-63.911488627533,58.938083348327,63.3334815420054));
#217297=CARTESIAN_POINT('Ctrl Pts',(-63.8686493908154,59.3774255368191,
62.7604124769525));
#217298=CARTESIAN_POINT('Ctrl Pts',(-63.8038866668339,60.1101692074064,
61.9886376949769));
#217299=CARTESIAN_POINT('Ctrl Pts',(-63.782504051702,60.3658044398433,61.7463822267538));
#217300=CARTESIAN_POINT('Ctrl Pts',(-63.6782847466954,61.6850726855922,
60.6228146595963));
#217301=CARTESIAN_POINT('Ctrl Pts',(-63.6137547901267,62.7121484755578,
60.1202593968798));
#217302=CARTESIAN_POINT('Ctrl Pts',(-63.567539947994,63.4350769493012,59.8300991896842));
#217303=CARTESIAN_POINT('Origin',(-63.5675399484425,66.6819786653733,69.5522455184007));
#217304=CARTESIAN_POINT('Origin',(-33.9082782203809,71.5694543312839,71.5715374392096));
#217305=CARTESIAN_POINT('',(-48.5675364832709,63.3942272950246,68.1938899513175));
#217306=CARTESIAN_POINT('Origin',(-48.5675364832709,67.9391588995182,70.071657595992));
#217307=CARTESIAN_POINT('',(-38.5675364832709,65.8706796275105,69.2170521170417));
#217308=CARTESIAN_POINT('',(-32.6788877561441,67.3289754150603,69.8195563755258));
#217309=CARTESIAN_POINT('Origin',(-38.5675364832709,70.4156112320045,71.094819761716));
#217310=CARTESIAN_POINT('Origin',(-33.5526503323277,75.000050506625,72.9851176492631));
#217311=CARTESIAN_POINT('Ctrl Pts',(-32.8170317109009,64.0574429575835,
68.4641091728316));
#217312=CARTESIAN_POINT('Ctrl Pts',(-32.8004854807068,64.3169522406309,
67.8359952786588));
#217313=CARTESIAN_POINT('Ctrl Pts',(-32.7839014352646,64.6301458058209,
67.2311874179812));
#217314=CARTESIAN_POINT('Ctrl Pts',(-32.7577872560977,65.2098387558858,
66.3146217715989));
#217315=CARTESIAN_POINT('Ctrl Pts',(-32.7480640102422,65.4434037099935,
65.9840989579143));
#217316=CARTESIAN_POINT('Ctrl Pts',(-32.7284199955665,65.9448748761847,
65.3464375126087));
#217317=CARTESIAN_POINT('Ctrl Pts',(-32.7185111528489,66.2126356336371,
65.0398690125399));
#217318=CARTESIAN_POINT('Ctrl Pts',(-32.7085755548516,66.4956396733205,
64.7476924450699));
#217319=CARTESIAN_POINT('Ctrl Pts',(-32.405898694983,66.4955863073276,64.7477475410809));
#217320=CARTESIAN_POINT('Ctrl Pts',(-32.4157698035306,66.213348129375,65.0391372016825));
#217321=CARTESIAN_POINT('Ctrl Pts',(-32.4256531061311,65.9462722690278,
65.3448398996728));
#217322=CARTESIAN_POINT('Ctrl Pts',(-32.4455076405886,65.4459673773228,
65.9806621814781));
#217323=CARTESIAN_POINT('Ctrl Pts',(-32.4554650299131,65.2128843628617,
66.3102185355673));
#217324=CARTESIAN_POINT('Ctrl Pts',(-32.4822602035662,64.6321241580052,
67.2273710034534));
#217325=CARTESIAN_POINT('Ctrl Pts',(-32.4988212117524,64.3177744264465,
67.8340052739125));
#217326=CARTESIAN_POINT('Ctrl Pts',(-32.5154663295374,64.0574429734829,
68.464109134349));
#217327=CARTESIAN_POINT('Origin',(-27.5423496375577,75.0034579025039,72.9903965241317));
#217328=CARTESIAN_POINT('',(-26.6969350937309,85.8892594304089,68.3402735649357));
#217329=CARTESIAN_POINT('Ctrl Pts',(-27.3723203524304,64.0608503540383,
68.4693880462876));
#217330=CARTESIAN_POINT('Ctrl Pts',(-27.3636083508722,64.1963234386015,
68.1414902321119));
#217331=CARTESIAN_POINT('Ctrl Pts',(-27.3549286023609,64.3465425592909,
67.8196629334019));
#217332=CARTESIAN_POINT('Ctrl Pts',(-27.3282627997169,64.8558294458032,
66.8455262589266));
#217333=CARTESIAN_POINT('Ctrl Pts',(-27.3103235216662,65.2619469917959,
66.2201115322032));
#217334=CARTESIAN_POINT('Ctrl Pts',(-27.2828026355142,65.9604358332311,
65.3386795099181));
#217335=CARTESIAN_POINT('Ctrl Pts',(-27.2734567296289,66.2110529133169,
65.0519687314779));
#217336=CARTESIAN_POINT('Ctrl Pts',(-27.245066551039,67.0174939103502,64.2145128591131));
#217337=CARTESIAN_POINT('Ctrl Pts',(-27.2263832459524,67.6144245613412,
63.7063271980707));
#217338=CARTESIAN_POINT('Ctrl Pts',(-27.1891136084416,68.8734807525916,
62.8333216632523));
#217339=CARTESIAN_POINT('Ctrl Pts',(-27.1706736189322,69.5290999489451,
62.4654641131916));
#217340=CARTESIAN_POINT('Ctrl Pts',(-27.1336442139279,70.930533160993,61.8457387365238));
#217341=CARTESIAN_POINT('Ctrl Pts',(-27.114869717408,71.6755617429044,61.6010497180737));
#217342=CARTESIAN_POINT('Ctrl Pts',(-27.0865099410825,72.8108792767892,
61.3491906253156));
#217343=CARTESIAN_POINT('Ctrl Pts',(-27.0771965350934,73.1862592610267,
61.2847199112335));
#217344=CARTESIAN_POINT('Ctrl Pts',(-27.0489438087402,74.3398690787609,
61.1434269784995));
#217345=CARTESIAN_POINT('Ctrl Pts',(-27.0303330568264,75.1231517273981,
61.1254601993129));
#217346=CARTESIAN_POINT('Ctrl Pts',(-26.9931925794068,76.6492291764433,
61.2416734538101));
#217347=CARTESIAN_POINT('Ctrl Pts',(-26.9748402774108,77.3889104563919,
61.3692657145651));
#217348=CARTESIAN_POINT('Ctrl Pts',(-26.938795595598,78.8323833935359,61.7619711097928));
#217349=CARTESIAN_POINT('Ctrl Pts',(-26.9208878747678,79.5330222579624,
62.0258512466808));
#217350=CARTESIAN_POINT('Ctrl Pts',(-26.8941989674047,80.517902234919,62.507406217329));
#217351=CARTESIAN_POINT('Ctrl Pts',(-26.8856673209247,80.8247494306158,
62.6746441595046));
#217352=CARTESIAN_POINT('Ctrl Pts',(-26.8623096935396,81.6468353161753,
63.1710735303491));
#217353=CARTESIAN_POINT('Ctrl Pts',(-26.8477100682122,82.1446780906913,
63.5269646820952));
#217354=CARTESIAN_POINT('Ctrl Pts',(-26.8106405787466,83.3217913773637,
64.5144381125695));
#217355=CARTESIAN_POINT('Ctrl Pts',(-26.7879383785396,83.9585912266568,
65.1902600866419));
#217356=CARTESIAN_POINT('Ctrl Pts',(-26.7544742250297,84.7850437718349,
66.3035874355147));
#217357=CARTESIAN_POINT('Ctrl Pts',(-26.7434170636367,85.0380446815753,
66.6896103302929));
#217358=CARTESIAN_POINT('Ctrl Pts',(-26.7210007035527,85.5001575689806,
67.4934282204171));
#217359=CARTESIAN_POINT('Ctrl Pts',(-26.7096581122749,85.7083720127467,
67.9108125373918));
#217360=CARTESIAN_POINT('Ctrl Pts',(-26.6982749890421,85.8914418320366,
68.3393768975646));
#217361=CARTESIAN_POINT('',(-26.3969350937309,85.8892594304089,68.3402735649357));
#217362=CARTESIAN_POINT('Origin',(-26.5469350937305,96.4455563604996,63.8278257377735));
#217363=CARTESIAN_POINT('Ctrl Pts',(-26.3955978506944,85.8914161878377,
68.3393168652454));
#217364=CARTESIAN_POINT('Ctrl Pts',(-26.4069424532441,85.7082672857083,
67.9105739168034));
#217365=CARTESIAN_POINT('Ctrl Pts',(-26.4183060567836,85.4999541203497,
67.4930236579193));
#217366=CARTESIAN_POINT('Ctrl Pts',(-26.4411055617826,85.0376098948105,
66.6889042588434));
#217367=CARTESIAN_POINT('Ctrl Pts',(-26.4525195276528,84.784476428515,66.3027447677285));
#217368=CARTESIAN_POINT('Ctrl Pts',(-26.4866843036473,83.9575372610834,
65.1889978992038));
#217369=CARTESIAN_POINT('Ctrl Pts',(-26.5089624396364,83.3203257906962,
64.5129519255814));
#217370=CARTESIAN_POINT('Ctrl Pts',(-26.5468362097196,82.1423355604167,
63.5251696793379));
#217371=CARTESIAN_POINT('Ctrl Pts',(-26.5620028980466,81.6440422855065,
63.1691573508409));
#217372=CARTESIAN_POINT('Ctrl Pts',(-26.5854952714911,80.8212819763206,
62.672682604541));
#217373=CARTESIAN_POINT('Ctrl Pts',(-26.593993736307,80.5142317372497,62.5054706945374));
#217374=CARTESIAN_POINT('Ctrl Pts',(-26.6207668794961,79.5292371216922,
62.0243042286113));
#217375=CARTESIAN_POINT('Ctrl Pts',(-26.6392010159838,78.8287305938289,
61.7607422846029));
#217376=CARTESIAN_POINT('Ctrl Pts',(-26.6761140325086,77.3852967816935,
61.3685194934542));
#217377=CARTESIAN_POINT('Ctrl Pts',(-26.6942100883925,76.645497311909,61.2411459204877));
#217378=CARTESIAN_POINT('Ctrl Pts',(-26.7317170578095,75.1192896074915,
61.125421304211));
#217379=CARTESIAN_POINT('Ctrl Pts',(-26.7511351157852,74.3360036358257,
61.1436434746849));
#217380=CARTESIAN_POINT('Ctrl Pts',(-26.7795748988597,73.1824395779273,
61.2853138249492));
#217381=CARTESIAN_POINT('Ctrl Pts',(-26.7888184636904,72.8070891584055,
61.3499053790692));
#217382=CARTESIAN_POINT('Ctrl Pts',(-26.8171824107733,71.6718535410123,
61.6021333424868));
#217383=CARTESIAN_POINT('Ctrl Pts',(-26.8364701637274,70.9268972234152,
61.8470682365406));
#217384=CARTESIAN_POINT('Ctrl Pts',(-26.874194477388,69.5255826413186,62.4672877684926));
#217385=CARTESIAN_POINT('Ctrl Pts',(-26.8922652752125,68.8700062214772,
62.8354121921109));
#217386=CARTESIAN_POINT('Ctrl Pts',(-26.9297343577378,67.6111740793825,
63.7089150024354));
#217387=CARTESIAN_POINT('Ctrl Pts',(-26.9491080822801,67.0144189406217,
64.2173116018839));
#217388=CARTESIAN_POINT('Ctrl Pts',(-26.977436758888,66.2082763058487,65.0550456594374));
#217389=CARTESIAN_POINT('Ctrl Pts',(-26.986646521672,65.957766563227,65.3418357651074));
#217390=CARTESIAN_POINT('Ctrl Pts',(-27.0139829799489,65.259725731252,66.223332594727));
#217391=CARTESIAN_POINT('Ctrl Pts',(-27.032253517993,64.8539281411214,66.8486943828843));
#217392=CARTESIAN_POINT('Ctrl Pts',(-27.059181657337,64.3455656836393,67.8217560871422));
#217393=CARTESIAN_POINT('Ctrl Pts',(-27.0677840356311,64.1958829423296,
68.1425564084808));
#217394=CARTESIAN_POINT('Ctrl Pts',(-27.0763524848464,64.060850369775,68.4693880081986));
#217395=CARTESIAN_POINT('Origin',(-49.8209604129909,64.4114212759519,68.6141501690631));
#217396=CARTESIAN_POINT('',(-47.4206117411878,75.1063969238644,65.7294283639652));
#217397=CARTESIAN_POINT('',(-47.4206117411893,69.9514311215947,78.2064603659042));
#217398=CARTESIAN_POINT('Ctrl Pts',(-47.4206117411876,75.1063969238639,
65.7294283639681));
#217399=CARTESIAN_POINT('Ctrl Pts',(-47.4072073505217,75.4654570754911,
66.753376001073));
#217400=CARTESIAN_POINT('Ctrl Pts',(-47.3965597695574,75.6742150489095,
67.8789541701247));
#217401=CARTESIAN_POINT('Ctrl Pts',(-47.3802442358666,75.7060386894703,
70.3818352645528));
#217402=CARTESIAN_POINT('Ctrl Pts',(-47.3761425330335,75.4276871521554,
71.7610264219768));
#217403=CARTESIAN_POINT('Ctrl Pts',(-47.3761425330335,74.9319958756762,
72.9607930464209));
#217404=CARTESIAN_POINT('Ctrl Pts',(-47.3761425330335,74.436304599197,74.1605596708651));
#217405=CARTESIAN_POINT('Ctrl Pts',(-47.3802442358666,73.6600106712586,
75.3340227356814));
#217406=CARTESIAN_POINT('Ctrl Pts',(-47.3965597695574,71.8708611554573,
77.0845570904024));
#217407=CARTESIAN_POINT('Ctrl Pts',(-47.4072073505217,70.9285149405077,
77.7345491805734));
#217408=CARTESIAN_POINT('Ctrl Pts',(-47.4206117411876,69.9514311215941,
78.2064603659031));
#217409=CARTESIAN_POINT('',(-40.481003278332,71.6699920780342,78.9164948483173));
#217410=CARTESIAN_POINT('',(-47.4206117411909,69.9514311215961,78.2064603659048));
#217411=CARTESIAN_POINT('',(-40.5852420615047,77.1637469693094,67.7517760446659));
#217412=CARTESIAN_POINT('Ctrl Pts',(-40.4810032783342,71.6699920780332,
78.9164948483157));
#217413=CARTESIAN_POINT('Ctrl Pts',(-40.5698846854173,72.6193246413771,
78.4352946931042));
#217414=CARTESIAN_POINT('Ctrl Pts',(-40.6457193000517,73.5311457149865,
77.7824385307885));
#217415=CARTESIAN_POINT('Ctrl Pts',(-40.7675094263889,75.2904244826386,
76.022759538046));
#217416=CARTESIAN_POINT('Ctrl Pts',(-40.8007888323695,76.0625615407368,
74.838403107781));
#217417=CARTESIAN_POINT('Ctrl Pts',(-40.8007888323695,76.5603508765695,
73.6335583596984));
#217418=CARTESIAN_POINT('Ctrl Pts',(-40.8007888323695,77.056970474425,72.4315448346997));
#217419=CARTESIAN_POINT('Ctrl Pts',(-40.7676642501064,77.3459151424127,
71.0508555808169));
#217420=CARTESIAN_POINT('Ctrl Pts',(-40.668740252843,77.3442754006263,69.0254326994105));
#217421=CARTESIAN_POINT('Ctrl Pts',(-40.6299225890052,77.2825638962586,
68.3789914813538));
#217422=CARTESIAN_POINT('Ctrl Pts',(-40.5852420615047,77.1637469693094,
67.7517760446659));
#217423=CARTESIAN_POINT('',(-40.481003278332,76.8249578803026,66.4394628463787));
#217424=CARTESIAN_POINT('Ctrl Pts',(-40.5852420615047,77.1637469693094,
67.7517760446659));
#217425=CARTESIAN_POINT('Ctrl Pts',(-40.5532232597647,77.0786008029555,
67.3023031346758));
#217426=CARTESIAN_POINT('Ctrl Pts',(-40.5182082030455,76.9642837773573,
66.8626329204887));
#217427=CARTESIAN_POINT('Ctrl Pts',(-40.4810032783489,76.824957880356,66.4394628465471));
#217428=CARTESIAN_POINT('',(-47.4206117411909,75.1063969238651,65.7294283639647));
#217429=CARTESIAN_POINT('Origin',(-64.4265543961493,66.6762871555627,69.5530424137804));
#217430=CARTESIAN_POINT('',(-64.5675364832712,59.0462179431737,64.6166308207574));
#217431=CARTESIAN_POINT('Origin',(-64.5675364832709,66.6762871555627,69.5530424137804));
#217432=CARTESIAN_POINT('',(-63.7081759237673,75.0753993185238,73.0230612142441));
#217433=CARTESIAN_POINT('Ctrl Pts',(-64.5675364832717,59.046217943174,64.6166308207575));
#217434=CARTESIAN_POINT('Ctrl Pts',(-64.5460054318702,59.4140720830844,
64.0480492722603));
#217435=CARTESIAN_POINT('Ctrl Pts',(-64.5242151510805,59.844353182852,63.5223301109439));
#217436=CARTESIAN_POINT('Ctrl Pts',(-64.4802433842163,60.8230886227947,
62.5671481746462));
#217437=CARTESIAN_POINT('Ctrl Pts',(-64.4585326795741,61.3704534354962,
62.1428615462339));
#217438=CARTESIAN_POINT('Ctrl Pts',(-64.4216367999338,62.3527328725573,
61.5465778287498));
#217439=CARTESIAN_POINT('Ctrl Pts',(-64.4067804331069,62.7623749275686,
61.3385500692314));
#217440=CARTESIAN_POINT('Ctrl Pts',(-64.3730365308062,63.7305523780891,
60.9358123869345));
#217441=CARTESIAN_POINT('Ctrl Pts',(-64.3544190590795,64.2958995002949,
60.7628340472615));
#217442=CARTESIAN_POINT('Ctrl Pts',(-64.3166439831112,65.4503787733972,
60.529236790111));
#217443=CARTESIAN_POINT('Ctrl Pts',(-64.2975574490637,66.0367054215919,
60.4688337160353));
#217444=CARTESIAN_POINT('Ctrl Pts',(-64.2597495591603,67.2149662863187,
60.4621504002003));
#217445=CARTESIAN_POINT('Ctrl Pts',(-64.241099252248,67.8041172201248,60.5163118771831));
#217446=CARTESIAN_POINT('Ctrl Pts',(-64.2031978910308,68.9629880021758,
60.7380099725469));
#217447=CARTESIAN_POINT('Ctrl Pts',(-64.184061183931,69.5299767860601,60.9049062666254));
#217448=CARTESIAN_POINT('Ctrl Pts',(-64.1557944571638,70.3503120297366,
61.2359124218975));
#217449=CARTESIAN_POINT('Ctrl Pts',(-64.1464291167281,70.6182984868461,
61.3595292794476));
#217450=CARTESIAN_POINT('Ctrl Pts',(-64.1276217352215,71.1414282045385,
61.6324545404921));
#217451=CARTESIAN_POINT('Ctrl Pts',(-64.1181904779768,71.3962528025367,
61.781612700772));
#217452=CARTESIAN_POINT('Ctrl Pts',(-64.0897741094686,72.136961432337,62.2650675446127));
#217453=CARTESIAN_POINT('Ctrl Pts',(-64.0707214808187,72.5980472818162,
62.6344941894086));
#217454=CARTESIAN_POINT('Ctrl Pts',(-64.0332160558767,73.4422542529727,
63.4575197792183));
#217455=CARTESIAN_POINT('Ctrl Pts',(-64.014559870328,73.8233529525379,63.909182428562));
#217456=CARTESIAN_POINT('Ctrl Pts',(-63.9767300455895,74.4926660386445,
64.8799364829341));
#217457=CARTESIAN_POINT('Ctrl Pts',(-63.9578042896901,74.7792988665418,
65.3967325233348));
#217458=CARTESIAN_POINT('Ctrl Pts',(-63.9297910614553,75.1312269161829,
66.2083219024603));
#217459=CARTESIAN_POINT('Ctrl Pts',(-63.9204656552382,75.2353509543835,
66.4845593731602));
#217460=CARTESIAN_POINT('Ctrl Pts',(-63.8941532883585,75.4893852620833,
67.2727750529987));
#217461=CARTESIAN_POINT('Ctrl Pts',(-63.877060576949,75.6079511899779,67.7935855420381));
#217462=CARTESIAN_POINT('Ctrl Pts',(-63.8344751232092,75.7886203399767,
69.1147594772785));
#217463=CARTESIAN_POINT('Ctrl Pts',(-63.8095863687707,75.7918272774603,
69.918609411374));
#217464=CARTESIAN_POINT('Ctrl Pts',(-63.7713711901292,75.6386878668021,
71.1091500668137));
#217465=CARTESIAN_POINT('Ctrl Pts',(-63.7585739829325,75.5615242742643,
71.5020572684633));
#217466=CARTESIAN_POINT('Ctrl Pts',(-63.7332377069494,75.3560332950464,
72.2747690093564));
#217467=CARTESIAN_POINT('Ctrl Pts',(-63.7207474086351,75.2279788898429,
72.6537453669887));
#217468=CARTESIAN_POINT('Ctrl Pts',(-63.7081759237673,75.0753993185238,
73.0230612142441));
#217469=CARTESIAN_POINT('Ctrl Pts',(-63.7081759237673,75.0753993185238,
73.0230612142441));
#217470=CARTESIAN_POINT('Ctrl Pts',(-63.6875161657482,74.8246527237304,
73.6299884083759));
#217471=CARTESIAN_POINT('Ctrl Pts',(-63.6666330962714,74.5088568775848,
74.2079528890887));
#217472=CARTESIAN_POINT('Ctrl Pts',(-63.625033817803,73.7584474523042,75.285397747626));
#217473=CARTESIAN_POINT('Ctrl Pts',(-63.604712906491,73.3260967966463,75.7817602801978));
#217474=CARTESIAN_POINT('Ctrl Pts',(-63.5702347770151,72.5230362672801,
76.5238902708135));
#217475=CARTESIAN_POINT('Ctrl Pts',(-63.5563499250237,72.1810151983127,
76.7970165522756));
#217476=CARTESIAN_POINT('Ctrl Pts',(-63.5238782363532,71.3348165170477,
77.3781042268528));
#217477=CARTESIAN_POINT('Ctrl Pts',(-63.5056266428151,70.8176553251907,
77.6636872419475));
#217478=CARTESIAN_POINT('Ctrl Pts',(-63.4686546174704,69.7360997838413,
78.1303410844429));
#217479=CARTESIAN_POINT('Ctrl Pts',(-63.4499671432274,69.1743365019085,
78.3104533209256));
#217480=CARTESIAN_POINT('Ctrl Pts',(-63.412843637122,68.02296300716,78.5597118792829));
#217481=CARTESIAN_POINT('Ctrl Pts',(-63.3946215167477,67.4360343720838,
78.6280860916995));
#217482=CARTESIAN_POINT('Ctrl Pts',(-63.3575823140898,66.2577744649439,
78.6501758674783));
#217483=CARTESIAN_POINT('Ctrl Pts',(-63.3388446223193,65.6692399052088,
78.6039452830318));
#217484=CARTESIAN_POINT('Ctrl Pts',(-63.3018702281337,64.5101588768287,
78.3983799325527));
#217485=CARTESIAN_POINT('Ctrl Pts',(-63.283646501263,63.9423247648397,78.2396736254702));
#217486=CARTESIAN_POINT('Ctrl Pts',(-63.2465196644465,62.844006377131,77.814240414913));
#217487=CARTESIAN_POINT('Ctrl Pts',(-63.2277373367691,62.3162201136205,
77.5482653071633));
#217488=CARTESIAN_POINT('Ctrl Pts',(-63.1907483518579,61.3200174392572,
76.9180689523048));
#217489=CARTESIAN_POINT('Ctrl Pts',(-63.1724068011774,60.8539177174493,
76.5554173534265));
#217490=CARTESIAN_POINT('Ctrl Pts',(-63.1350988645248,59.9983322733126,
75.7448462794558));
#217491=CARTESIAN_POINT('Ctrl Pts',(-63.1163171878295,59.6109016499769,
75.2988106682674));
#217492=CARTESIAN_POINT('Ctrl Pts',(-63.0840698114675,59.0161042143516,
74.462098201395));
#217493=CARTESIAN_POINT('Ctrl Pts',(-63.070383528129,58.7888527537334,74.0879744284649));
#217494=CARTESIAN_POINT('Ctrl Pts',(-63.03575802426,58.2899042873179,73.1147421819726));
#217495=CARTESIAN_POINT('Ctrl Pts',(-63.0147220449659,58.0545822896112,
72.499792039988));
#217496=CARTESIAN_POINT('Ctrl Pts',(-62.9836482387311,57.8040493638457,
71.5473602390957));
#217497=CARTESIAN_POINT('Ctrl Pts',(-62.973330254332,57.7377964778962,71.2255528877246));
#217498=CARTESIAN_POINT('Ctrl Pts',(-62.9525789218377,57.640511421009,70.5768646016961));
#217499=CARTESIAN_POINT('Ctrl Pts',(-62.9421606938526,57.6094772131815,
70.2504729419999));
#217500=CARTESIAN_POINT('Ctrl Pts',(-62.931689741507,57.5961353792733,69.9231225687745));
#217501=CARTESIAN_POINT('',(-63.5151079737584,75.0753363416539,73.023213644598));
#217502=CARTESIAN_POINT('Ctrl Pts',(-63.5151079737584,75.0753363416539,
73.023213644598));
#217503=CARTESIAN_POINT('Ctrl Pts',(-63.4920115368903,74.8003777464773,
73.6887112847482));
#217504=CARTESIAN_POINT('Ctrl Pts',(-63.4695346041823,74.4472985330117,
74.3191708931087));
#217505=CARTESIAN_POINT('Ctrl Pts',(-63.423566941987,73.6004910487312,75.4824790007821));
#217506=CARTESIAN_POINT('Ctrl Pts',(-63.4000847322133,73.1099911278997,
76.0113920820928));
#217507=CARTESIAN_POINT('Ctrl Pts',(-63.361777030342,72.1979722538408,76.7866989681039));
#217508=CARTESIAN_POINT('Ctrl Pts',(-63.3466926852378,71.8097504735447,
77.0671855931678));
#217509=CARTESIAN_POINT('Ctrl Pts',(-63.2938297827708,70.3901047296146,
77.9312832124918));
#217510=CARTESIAN_POINT('Ctrl Pts',(-63.2553240369309,69.2683698962628,
78.3432902940439));
#217511=CARTESIAN_POINT('Ctrl Pts',(-63.1802061532443,66.9313631514609,
78.7137875751332));
#217512=CARTESIAN_POINT('Ctrl Pts',(-63.1416991694266,65.7385098139196,
78.669231390451));
#217513=CARTESIAN_POINT('Ctrl Pts',(-63.0854654839921,64.0155033228014,
78.2623486117566));
#217514=CARTESIAN_POINT('Ctrl Pts',(-63.0668904991214,63.4577723005613,
78.0720177871324));
#217515=CARTESIAN_POINT('Ctrl Pts',(-63.0288042469598,62.3857775646909,
77.5857743798567));
#217516=CARTESIAN_POINT('Ctrl Pts',(-63.0097643437471,61.8741393887536,
77.2907842916304));
#217517=CARTESIAN_POINT('Ctrl Pts',(-62.9722947176107,60.9161297538726,
76.6065876086381));
#217518=CARTESIAN_POINT('Ctrl Pts',(-62.9539264956367,60.4718989600415,
76.2191865236179));
#217519=CARTESIAN_POINT('Ctrl Pts',(-62.91777620211,59.6982676713801,75.3997319054868));
#217520=CARTESIAN_POINT('Ctrl Pts',(-62.9002893758449,59.3639057394616,
74.9757373538693));
#217521=CARTESIAN_POINT('Ctrl Pts',(-62.8569675334043,58.6228572569014,
73.8418303929263));
#217522=CARTESIAN_POINT('Ctrl Pts',(-62.8317663795232,58.2705836499956,
73.1020680896929));
#217523=CARTESIAN_POINT('Ctrl Pts',(-62.7795181749645,57.772579724387,71.5473692252264));
#217524=CARTESIAN_POINT('Ctrl Pts',(-62.7533222274278,57.629410894498,70.7393858054451));
#217525=CARTESIAN_POINT('Ctrl Pts',(-62.7276560748581,57.5961385652529,
69.9232007305414));
#217526=CARTESIAN_POINT('Ctrl Pts',(-64.4174334691588,58.2772202579663,
66.0829140514177));
#217527=CARTESIAN_POINT('Ctrl Pts',(-64.4028363489011,58.4518252279933,
65.6603017815621));
#217528=CARTESIAN_POINT('Ctrl Pts',(-64.388254068226,58.6580800871412,65.2514650584679));
#217529=CARTESIAN_POINT('Ctrl Pts',(-64.3594594276788,59.1299016586449,
64.4691031862401));
#217530=CARTESIAN_POINT('Ctrl Pts',(-64.3452859445577,59.3946760999142,
64.0966228430422));
#217531=CARTESIAN_POINT('Ctrl Pts',(-64.3026020263834,60.268874083405,63.0444148664755));
#217532=CARTESIAN_POINT('Ctrl Pts',(-64.2733419665553,60.9536431133377,
62.4348608785046));
#217533=CARTESIAN_POINT('Ctrl Pts',(-64.2264359972265,62.2072784339748,
61.6185901131439));
#217534=CARTESIAN_POINT('Ctrl Pts',(-64.2084843858883,62.72657227493,61.347720171344));
#217535=CARTESIAN_POINT('Ctrl Pts',(-64.1715858497388,63.8140295268703,
60.9078005015644));
#217536=CARTESIAN_POINT('Ctrl Pts',(-64.152733349663,64.3799657775133,60.7405714862318));
#217537=CARTESIAN_POINT('Ctrl Pts',(-64.1156388352873,65.5353959314313,
60.5181036515844));
#217538=CARTESIAN_POINT('Ctrl Pts',(-64.0974824103457,66.122123731388,60.4632319430865));
#217539=CARTESIAN_POINT('Ctrl Pts',(-64.060817865302,67.2978133386995,60.467597049163));
#217540=CARTESIAN_POINT('Ctrl Pts',(-64.0420536590333,67.8839943754661,
60.5268009521494));
#217541=CARTESIAN_POINT('Ctrl Pts',(-64.0046823532411,69.0393038763928,
60.7581054577239));
#217542=CARTESIAN_POINT('Ctrl Pts',(-63.9862706923076,69.605607286876,60.930174162333));
#217543=CARTESIAN_POINT('Ctrl Pts',(-63.9309385666082,71.2472767084625,
61.6095373623021));
#217544=CARTESIAN_POINT('Ctrl Pts',(-63.8929715723796,72.2440018990052,
62.2733606589597));
#217545=CARTESIAN_POINT('Ctrl Pts',(-63.8466555645126,73.2940183642383,
63.3177684313763));
#217546=CARTESIAN_POINT('Ctrl Pts',(-63.8374744635571,73.4927744769004,
63.5356918745553));
#217547=CARTESIAN_POINT('Ctrl Pts',(-63.8096802469964,74.0566727572609,
64.2178346791088));
#217548=CARTESIAN_POINT('Ctrl Pts',(-63.7906820867554,74.3875346091592,
64.7083363402621));
#217549=CARTESIAN_POINT('Ctrl Pts',(-63.7624534805635,74.8089437801989,
65.4869523152072));
#217550=CARTESIAN_POINT('Ctrl Pts',(-63.7531027711834,74.9366784331414,
65.7531568340785));
#217551=CARTESIAN_POINT('Ctrl Pts',(-63.7252693288848,75.2794825367097,
66.5669372241555));
#217552=CARTESIAN_POINT('Ctrl Pts',(-63.7070369345556,75.4546067534806,
67.1296363690236));
#217553=CARTESIAN_POINT('Ctrl Pts',(-63.6595558906483,75.7569768036545,
68.585706998936));
#217554=CARTESIAN_POINT('Ctrl Pts',(-63.6306895773755,75.8081294161607,
69.4884288883275));
#217555=CARTESIAN_POINT('Ctrl Pts',(-63.5879995871343,75.6843268963693,
70.8368980257031));
#217556=CARTESIAN_POINT('Ctrl Pts',(-63.5736937694455,75.6087802633196,
71.2861407676666));
#217557=CARTESIAN_POINT('Ctrl Pts',(-63.5444428965403,75.3910183266301,
72.1696495296368));
#217558=CARTESIAN_POINT('Ctrl Pts',(-63.5297035283193,75.2490935839844,
72.602659289293));
#217559=CARTESIAN_POINT('Ctrl Pts',(-63.5151079737584,75.0753363416539,
73.023213644598));
#217560=CARTESIAN_POINT('Origin',(-61.5936228798467,66.6770802411476,69.5524554490054));
#217561=CARTESIAN_POINT('',(-56.4535514884218,75.0783661981676,73.0234382919152));
#217562=CARTESIAN_POINT('Ctrl Pts',(-57.3654750286596,58.2758162995991,
66.081419319572));
#217563=CARTESIAN_POINT('Ctrl Pts',(-57.3600114213503,58.3418432452923,
65.9216083071428));
#217564=CARTESIAN_POINT('Ctrl Pts',(-57.354538030702,58.4124498587974,65.7636334960766));
#217565=CARTESIAN_POINT('Ctrl Pts',(-57.320335958553,58.8799319911198,64.7931181034278));
#217566=CARTESIAN_POINT('Ctrl Pts',(-57.2910632069123,59.3916444208721,
64.0416260517858));
#217567=CARTESIAN_POINT('Ctrl Pts',(-57.2531441869721,60.2044635996514,
63.163393185142));
#217568=CARTESIAN_POINT('Ctrl Pts',(-57.2438960971557,60.4133869689274,
62.9584408187008));
#217569=CARTESIAN_POINT('Ctrl Pts',(-57.2029172707919,61.3752732899755,
62.1018723117282));
#217570=CARTESIAN_POINT('Ctrl Pts',(-57.1706881268413,62.2224486874346,
61.5664300509027));
#217571=CARTESIAN_POINT('Ctrl Pts',(-57.1015161888563,64.2301218056132,
60.7182282354967));
#217572=CARTESIAN_POINT('Ctrl Pts',(-57.0632515782325,65.4003685532868,
60.4749454867403));
#217573=CARTESIAN_POINT('Ctrl Pts',(-57.0072783845977,67.1622342804553,
60.4569626146788));
#217574=CARTESIAN_POINT('Ctrl Pts',(-56.9889189922805,67.7394058978863,
60.5061953742382));
#217575=CARTESIAN_POINT('Ctrl Pts',(-56.9519861589916,68.8662837545505,
60.7117096933882));
#217576=CARTESIAN_POINT('Ctrl Pts',(-56.9336163160537,69.4138340516044,
60.8655922982073));
#217577=CARTESIAN_POINT('Ctrl Pts',(-56.8975593860576,70.4722303191574,
61.273130373858));
#217578=CARTESIAN_POINT('Ctrl Pts',(-56.8796493552864,70.9808100854609,
61.5257316508818));
#217579=CARTESIAN_POINT('Ctrl Pts',(-56.8444604524034,71.9121132112754,
62.1023983358425));
#217580=CARTESIAN_POINT('Ctrl Pts',(-56.8273003940205,72.3365280341286,
62.4194634437235));
#217581=CARTESIAN_POINT('Ctrl Pts',(-56.7937435649933,73.120819616518,63.1196740244442));
#217582=CARTESIAN_POINT('Ctrl Pts',(-56.7773285095329,73.4799297330221,
63.5007037465333));
#217583=CARTESIAN_POINT('Ctrl Pts',(-56.7445659828364,74.1180595577877,
64.3068205305523));
#217584=CARTESIAN_POINT('Ctrl Pts',(-56.7282914253951,74.3982024995525,
64.7286475597634));
#217585=CARTESIAN_POINT('Ctrl Pts',(-56.6928818440938,74.9290291194141,
65.693724022836));
#217586=CARTESIAN_POINT('Ctrl Pts',(-56.6741711027392,75.1641923499117,
66.2428631704159));
#217587=CARTESIAN_POINT('Ctrl Pts',(-56.6222397366015,75.6589306397739,
67.8069613270961));
#217588=CARTESIAN_POINT('Ctrl Pts',(-56.5886376242235,75.7999415281365,
68.8497498836176));
#217589=CARTESIAN_POINT('Ctrl Pts',(-56.5218871145513,75.720361681532,70.9690038904761));
#217590=CARTESIAN_POINT('Ctrl Pts',(-56.4874035662131,75.4893105070773,
72.028774587768));
#217591=CARTESIAN_POINT('Ctrl Pts',(-56.4535514884218,75.0783661981675,
73.0234382919155));
#217592=CARTESIAN_POINT('Ctrl Pts',(-56.4535514884218,75.0783661981676,
73.0234382919152));
#217593=CARTESIAN_POINT('Ctrl Pts',(-56.4350025485805,74.8531929810001,
73.5684552720914));
#217594=CARTESIAN_POINT('Ctrl Pts',(-56.4166167441613,74.5755185238252,
74.0902687254798));
#217595=CARTESIAN_POINT('Ctrl Pts',(-56.379165442425,73.9223966155769,75.0736683009857));
#217596=CARTESIAN_POINT('Ctrl Pts',(-56.3602283265256,73.5483169666455,
75.532799775141));
#217597=CARTESIAN_POINT('Ctrl Pts',(-56.329596782838,72.861721139502,76.2253320190393));
#217598=CARTESIAN_POINT('Ctrl Pts',(-56.317634398701,72.574065311345,76.4808487169403));
#217599=CARTESIAN_POINT('Ctrl Pts',(-56.2894402152713,71.8658413552301,
77.0337944793754));
#217600=CARTESIAN_POINT('Ctrl Pts',(-56.2731540034383,71.4344701947586,
77.3152453931667));
#217601=CARTESIAN_POINT('Ctrl Pts',(-56.219130437151,69.9379628269114,78.119840148702));
#217602=CARTESIAN_POINT('Ctrl Pts',(-56.1828647639803,68.794575824452,78.4715164095075));
#217603=CARTESIAN_POINT('Ctrl Pts',(-56.1075989870263,66.4376023995509,
78.7162692581898));
#217604=CARTESIAN_POINT('Ctrl Pts',(-56.0713507169347,65.2466035010035,
78.6070995097047));
#217605=CARTESIAN_POINT('Ctrl Pts',(-56.0244312016594,63.8295822101941,
78.1899669390205));
#217606=CARTESIAN_POINT('Ctrl Pts',(-56.0151271426989,63.5531910934736,
78.0938936901133));
#217607=CARTESIAN_POINT('Ctrl Pts',(-55.9899598033859,62.8127982775836,
77.79577991316));
#217608=CARTESIAN_POINT('Ctrl Pts',(-55.9743076255857,62.3602629387578,
77.5680756017296));
#217609=CARTESIAN_POINT('Ctrl Pts',(-55.9325391958517,61.2253033703755,
76.8728703666199));
#217610=CARTESIAN_POINT('Ctrl Pts',(-55.9060931859003,60.5835592141638,
76.3479941800254));
#217611=CARTESIAN_POINT('Ctrl Pts',(-55.8672462318577,59.7404020141169,
75.4416090443032));
#217612=CARTESIAN_POINT('Ctrl Pts',(-55.8543960477821,59.4802236078311,
75.1206589282082));
#217613=CARTESIAN_POINT('Ctrl Pts',(-55.8280947723416,58.9994034129875,
74.437273983811));
#217614=CARTESIAN_POINT('Ctrl Pts',(-55.8146661895923,58.7804893176157,
74.0748461126787));
#217615=CARTESIAN_POINT('Ctrl Pts',(-55.8011708396429,58.5876049474126,
73.6985038205814));
#217616=CARTESIAN_POINT('',(-56.2580209956237,75.0782830932473,73.0236394350927));
#217617=CARTESIAN_POINT('Ctrl Pts',(-56.2580209956237,75.0782830932473,
73.0236394350927));
#217618=CARTESIAN_POINT('Ctrl Pts',(-56.2443250754476,74.9153795836255,
73.4179099304444));
#217619=CARTESIAN_POINT('Ctrl Pts',(-56.2305642181659,74.7249216441682,
73.8002275282812));
#217620=CARTESIAN_POINT('Ctrl Pts',(-56.2033211069302,74.2926394472272,
74.5337242263198));
#217621=CARTESIAN_POINT('Ctrl Pts',(-56.1898709563397,74.0515679752653,
74.8841262966464));
#217622=CARTESIAN_POINT('Ctrl Pts',(-56.1512855608215,73.2926281453491,
75.8368058676945));
#217623=CARTESIAN_POINT('Ctrl Pts',(-56.1256639711522,72.7192902604295,
76.3898681292527));
#217624=CARTESIAN_POINT('Ctrl Pts',(-56.0833810803595,71.6592287485016,
77.1736969095174));
#217625=CARTESIAN_POINT('Ctrl Pts',(-56.0667865829977,71.2106984557556,
77.4487477683132));
#217626=CARTESIAN_POINT('Ctrl Pts',(-56.0320548232101,70.2335982860813,
77.9370958618639));
#217627=CARTESIAN_POINT('Ctrl Pts',(-56.0136903834561,69.7036449059816,
78.1426188139804));
#217628=CARTESIAN_POINT('Ctrl Pts',(-55.9724037787782,68.4715783064651,
78.4921548134416));
#217629=CARTESIAN_POINT('Ctrl Pts',(-55.949910350296,67.7645969923614,78.6053971315291));
#217630=CARTESIAN_POINT('Ctrl Pts',(-55.9038224877719,66.32063622386,78.6649527140372));
#217631=CARTESIAN_POINT('Ctrl Pts',(-55.8800043454388,65.5886261276757,
78.6067319429835));
#217632=CARTESIAN_POINT('Ctrl Pts',(-55.8418580524031,64.4193801977491,
78.369766115404));
#217633=CARTESIAN_POINT('Ctrl Pts',(-55.8272928052753,63.9748501154927,
78.2438378961159));
#217634=CARTESIAN_POINT('Ctrl Pts',(-55.7936110388137,62.9815107330797,
77.8788240150706));
#217635=CARTESIAN_POINT('Ctrl Pts',(-55.7742461928927,62.4428615051065,
77.618249109084));
#217636=CARTESIAN_POINT('Ctrl Pts',(-55.7285410136336,61.2288299480985,
76.8756090000899));
#217637=CARTESIAN_POINT('Ctrl Pts',(-55.702797084058,60.5860673776397,76.3503647630496));
#217638=CARTESIAN_POINT('Ctrl Pts',(-55.6629912962454,59.7417569897272,
75.4432276991319));
#217639=CARTESIAN_POINT('Ctrl Pts',(-55.6496589375082,59.4813000808383,
75.1220745554703));
#217640=CARTESIAN_POINT('Ctrl Pts',(-55.6228882380845,58.9999281637497,
74.4381366140573));
#217641=CARTESIAN_POINT('Ctrl Pts',(-55.6094895732801,58.7807521867564,
74.0753471720821));
#217642=CARTESIAN_POINT('Ctrl Pts',(-55.5961206596756,58.5876577945761,
73.6986069305967));
#217643=CARTESIAN_POINT('Ctrl Pts',(-56.2580209956237,75.0782830932472,
73.0236394350929));
#217644=CARTESIAN_POINT('Ctrl Pts',(-56.2925645228312,75.4891544873887,
72.0292196802937));
#217645=CARTESIAN_POINT('Ctrl Pts',(-56.3259262120769,75.720220574439,70.9697133303432));
#217646=CARTESIAN_POINT('Ctrl Pts',(-56.3939371624248,75.7999941374542,
68.8513038344539));
#217647=CARTESIAN_POINT('Ctrl Pts',(-56.4262220314782,75.6592736023998,
67.8090700677666));
#217648=CARTESIAN_POINT('Ctrl Pts',(-56.4785201578563,75.1651878195993,
66.2454276235155));
#217649=CARTESIAN_POINT('Ctrl Pts',(-56.4975993377663,74.9302102895212,
65.6962571767317));
#217650=CARTESIAN_POINT('Ctrl Pts',(-56.5321607618762,74.4002121154711,
64.7319763436369));
#217651=CARTESIAN_POINT('Ctrl Pts',(-56.5479173463761,74.1208645287935,
64.3109042611982));
#217652=CARTESIAN_POINT('Ctrl Pts',(-56.5798968217344,73.494700938003,63.5188286320515));
#217653=CARTESIAN_POINT('Ctrl Pts',(-56.5960655252397,73.1488683908934,
63.1492876181003));
#217654=CARTESIAN_POINT('Ctrl Pts',(-56.6291348647592,72.3745662518574,
62.4490620080192));
#217655=CARTESIAN_POINT('Ctrl Pts',(-56.6458198189785,71.9436713366265,
62.1239585426187));
#217656=CARTESIAN_POINT('Ctrl Pts',(-56.68057172786,71.0045022454338,61.5383786275759));
#217657=CARTESIAN_POINT('Ctrl Pts',(-56.698616759336,70.4953636692314,61.2836762939568));
#217658=CARTESIAN_POINT('Ctrl Pts',(-56.7346963800063,69.4361721782398,
60.8726227487683));
#217659=CARTESIAN_POINT('Ctrl Pts',(-56.7523394831835,68.8884388797823,
60.7171863104021));
#217660=CARTESIAN_POINT('Ctrl Pts',(-56.788210763293,67.7606126669312,60.5086553183781));
#217661=CARTESIAN_POINT('Ctrl Pts',(-56.8064949562029,67.1826894315703,
60.4580225336636));
#217662=CARTESIAN_POINT('Ctrl Pts',(-56.8624826951612,65.4198876776316,
60.4722152519561));
#217663=CARTESIAN_POINT('Ctrl Pts',(-56.8987059340921,64.2490704839672,
60.7129950715433));
#217664=CARTESIAN_POINT('Ctrl Pts',(-56.9683110302751,62.2292604910183,
61.5612370468008));
#217665=CARTESIAN_POINT('Ctrl Pts',(-56.9992267960155,61.372290861921,62.1024960302811));
#217666=CARTESIAN_POINT('Ctrl Pts',(-57.0403799912866,60.4035474054354,
62.967811165195));
#217667=CARTESIAN_POINT('Ctrl Pts',(-57.0496874866844,60.1950846130766,
63.172918921827));
#217668=CARTESIAN_POINT('Ctrl Pts',(-57.0874168908922,59.3907537315826,
64.0445044560468));
#217669=CARTESIAN_POINT('Ctrl Pts',(-57.1149213725863,58.8848057559073,
64.7871075949958));
#217670=CARTESIAN_POINT('Ctrl Pts',(-57.1489580148019,58.417345561021,65.7526958298713));
#217671=CARTESIAN_POINT('Ctrl Pts',(-57.1546554757547,58.34413324798,65.9160656035786));
#217672=CARTESIAN_POINT('Ctrl Pts',(-57.1603612091034,58.2758162839768,
66.0814193573839));
#217673=CARTESIAN_POINT('Origin',(-54.462516693425,66.6776194928561,69.5544896765311));
#217674=CARTESIAN_POINT('',(-49.1982221066882,75.0787836866508,73.0257672246888));
#217675=CARTESIAN_POINT('Ctrl Pts',(-50.1089321285242,58.276355535683,66.0834535849087));
#217676=CARTESIAN_POINT('Ctrl Pts',(-50.1001648443086,58.3817700064601,
65.8283093655669));
#217677=CARTESIAN_POINT('Ctrl Pts',(-50.091357844461,58.4988095027559,65.5779622274588));
#217678=CARTESIAN_POINT('Ctrl Pts',(-50.0673733290039,58.845963509162,64.9158995804182));
#217679=CARTESIAN_POINT('Ctrl Pts',(-50.0521062390893,59.0968945962679,
64.5162399824942));
#217680=CARTESIAN_POINT('Ctrl Pts',(-50.0169043107424,59.7502004724591,
63.6357882095687));
#217681=CARTESIAN_POINT('Ctrl Pts',(-49.9973020698474,60.1735288431777,
63.1735046916622));
#217682=CARTESIAN_POINT('Ctrl Pts',(-49.9487203819678,61.309018185135,62.1649067208048));
#217683=CARTESIAN_POINT('Ctrl Pts',(-49.9197679943601,62.0609702146647,
61.6732222160602));
#217684=CARTESIAN_POINT('Ctrl Pts',(-49.8537474866652,63.9486953595311,
60.8031147818176));
#217685=CARTESIAN_POINT('Ctrl Pts',(-49.8154492956854,65.1115774613567,
60.5222633777277));
#217686=CARTESIAN_POINT('Ctrl Pts',(-49.7594774935417,66.8729653580385,
60.4481640659964));
#217687=CARTESIAN_POINT('Ctrl Pts',(-49.7411381157849,67.4513788983311,
60.4789943263066));
#217688=CARTESIAN_POINT('Ctrl Pts',(-49.7042566752863,68.5840971818238,
60.6485014929856));
#217689=CARTESIAN_POINT('Ctrl Pts',(-49.6859159986314,69.1361734434929,
60.7848368355366));
#217690=CARTESIAN_POINT('Ctrl Pts',(-49.6499316417008,70.2067879832496,
61.1583482922952));
#217691=CARTESIAN_POINT('Ctrl Pts',(-49.6320659057619,70.7230320092189,
61.3945352583048));
#217692=CARTESIAN_POINT('Ctrl Pts',(-49.5967204675263,71.6787861381583,
61.9449286177151));
#217693=CARTESIAN_POINT('Ctrl Pts',(-49.5793543595703,72.1190398580046,
62.2532544285809));
#217694=CARTESIAN_POINT('Ctrl Pts',(-49.5453889300942,72.9359702314459,
62.9405283869928));
#217695=CARTESIAN_POINT('Ctrl Pts',(-49.5287567027039,73.3116600494043,
63.3174270927594));
#217696=CARTESIAN_POINT('Ctrl Pts',(-49.4957981899007,73.9766818142036,
64.1130850896679));
#217697=CARTESIAN_POINT('Ctrl Pts',(-49.4795549896811,74.268112948659,64.5276022967562));
#217698=CARTESIAN_POINT('Ctrl Pts',(-49.4441253151381,74.8267113564275,
65.4823825902168));
#217699=CARTESIAN_POINT('Ctrl Pts',(-49.425367023484,75.0777970242852,66.0293264987477));
#217700=CARTESIAN_POINT('Ctrl Pts',(-49.3977762232747,75.362219709797,66.8559648315499));
#217701=CARTESIAN_POINT('Ctrl Pts',(-49.3891007077892,75.4395676361253,
67.1188007279758));
#217702=CARTESIAN_POINT('Ctrl Pts',(-49.3654086650421,75.6171323513174,
67.8411921227889));
#217703=CARTESIAN_POINT('Ctrl Pts',(-49.3503126636981,75.6937569548679,
68.3056733009986));
#217704=CARTESIAN_POINT('Ctrl Pts',(-49.3198465655125,75.7762413958645,
69.262778266938));
#217705=CARTESIAN_POINT('Ctrl Pts',(-49.3045871399129,75.7787263345094,
69.7541768791264));
#217706=CARTESIAN_POINT('Ctrl Pts',(-49.2589558776886,75.6688407380179,
71.1999922741479));
#217707=CARTESIAN_POINT('Ctrl Pts',(-49.2282365965666,75.4451500591753,
72.1390896231537));
#217708=CARTESIAN_POINT('Ctrl Pts',(-49.1982221066882,75.0787836866507,
73.025767224689));
#217709=CARTESIAN_POINT('',(-48.6677134573784,61.073680689161,76.7064654074421));
#217710=CARTESIAN_POINT('Ctrl Pts',(-49.1982221066882,75.0787836866508,
73.0257672246888));
#217711=CARTESIAN_POINT('Ctrl Pts',(-49.1846980472593,74.913704732624,73.4252902759224));
#217712=CARTESIAN_POINT('Ctrl Pts',(-49.1712011184087,74.7203369872293,
73.8125282475041));
#217713=CARTESIAN_POINT('Ctrl Pts',(-49.1439889436598,74.2813616534623,
74.5541839958143));
#217714=CARTESIAN_POINT('Ctrl Pts',(-49.1303097641346,74.0366450956581,
74.9078602743798));
#217715=CARTESIAN_POINT('Ctrl Pts',(-49.0903095212971,73.2480510597892,
75.8907898671893));
#217716=CARTESIAN_POINT('Ctrl Pts',(-49.0648068913569,72.6419027431399,
76.4643810840044));
#217717=CARTESIAN_POINT('Ctrl Pts',(-49.0230777014757,71.5671431419043,
77.2332124069004));
#217718=CARTESIAN_POINT('Ctrl Pts',(-49.007421009719,71.1454839454682,77.4859717459455));
#217719=CARTESIAN_POINT('Ctrl Pts',(-48.9742148605163,70.2023028886257,
77.9521673598388));
#217720=CARTESIAN_POINT('Ctrl Pts',(-48.9568877851838,69.6771598053905,
78.1537422593015));
#217721=CARTESIAN_POINT('Ctrl Pts',(-48.9237288294822,68.659861073702,78.4396159088877));
#217722=CARTESIAN_POINT('Ctrl Pts',(-48.9080191469994,68.1727776032606,
78.5344253154042));
#217723=CARTESIAN_POINT('Ctrl Pts',(-48.873683136384,67.0983379452549,78.6536821387682));
#217724=CARTESIAN_POINT('Ctrl Pts',(-48.8554489933668,66.5113839390646,
78.6618866060698));
#217725=CARTESIAN_POINT('Ctrl Pts',(-48.8094548318523,65.0461525300166,
78.5405983068835));
#217726=CARTESIAN_POINT('Ctrl Pts',(-48.7811658054655,64.1799336903606,
78.3393276644481));
#217727=CARTESIAN_POINT('Ctrl Pts',(-48.7396885135181,62.9521885669229,
77.8574497716699));
#217728=CARTESIAN_POINT('Ctrl Pts',(-48.7261817253743,62.5597652232474,
77.6699847473452));
#217729=CARTESIAN_POINT('Ctrl Pts',(-48.6985186227286,61.7952368833308,
77.2349803636798));
#217730=CARTESIAN_POINT('Ctrl Pts',(-48.6843884535666,61.4249317932819,
76.9866399323976));
#217731=CARTESIAN_POINT('Ctrl Pts',(-48.6701794005809,61.0743248382493,
76.7121720277602));
#217732=CARTESIAN_POINT('',(-48.4675099033474,61.0743873391425,76.7079526484011));
#217733=CARTESIAN_POINT('Ctrl Pts',(-48.6675364832709,61.0743296293729,
76.7064311666085));
#217734=CARTESIAN_POINT('Ctrl Pts',(-48.6008609566297,61.0742541501395,
76.7121166899682));
#217735=CARTESIAN_POINT('Ctrl Pts',(-48.5341854299886,61.0742541501395,
76.7121166899682));
#217736=CARTESIAN_POINT('Ctrl Pts',(-48.4675099033474,61.0743873391425,
76.7079526484011));
#217737=CARTESIAN_POINT('',(-49.0012377727522,75.0788851372981,73.0255216843006));
#217738=CARTESIAN_POINT('Ctrl Pts',(-49.0012377727522,75.0788851372981,
73.0255216843007));
#217739=CARTESIAN_POINT('Ctrl Pts',(-48.9869942993643,74.9103006428599,
73.433562612226));
#217740=CARTESIAN_POINT('Ctrl Pts',(-48.9727665448605,74.712211176133,73.828783606424));
#217741=CARTESIAN_POINT('Ctrl Pts',(-48.9446794933677,74.262118103884,74.5840306233706));
#217742=CARTESIAN_POINT('Ctrl Pts',(-48.9308529409508,74.0111842107319,
74.9433420219173));
#217743=CARTESIAN_POINT('Ctrl Pts',(-48.8896864537942,73.1958164999378,
75.9478730054749));
#217744=CARTESIAN_POINT('Ctrl Pts',(-48.8618295254075,72.5650857674712,
76.5330266537419));
#217745=CARTESIAN_POINT('Ctrl Pts',(-48.8153368443041,71.3676828645975,
77.3643920920264));
#217746=CARTESIAN_POINT('Ctrl Pts',(-48.7964053555865,70.8406624110098,
77.6575966007387));
#217747=CARTESIAN_POINT('Ctrl Pts',(-48.7622406354934,69.8684013814934,
78.0784464648355));
#217748=CARTESIAN_POINT('Ctrl Pts',(-48.7474157728122,69.435108204469,78.2283117361156));
#217749=CARTESIAN_POINT('Ctrl Pts',(-48.7035598202974,68.1125708753328,
78.5765719982624));
#217750=CARTESIAN_POINT('Ctrl Pts',(-48.6750545183228,67.2029530271456,
78.6748551441207));
#217751=CARTESIAN_POINT('Ctrl Pts',(-48.6306159838825,65.8273428269903,
78.6167461339114));
#217752=CARTESIAN_POINT('Ctrl Pts',(-48.6156168883705,65.3629184399787,
78.5611000819068));
#217753=CARTESIAN_POINT('Ctrl Pts',(-48.5787691667423,64.2272104950673,
78.3352724470749));
#217754=CARTESIAN_POINT('Ctrl Pts',(-48.5570481635002,63.5671604509319,
78.1237188431728));
#217755=CARTESIAN_POINT('Ctrl Pts',(-48.5231754596626,62.6083701607617,
77.6908842886743));
#217756=CARTESIAN_POINT('Ctrl Pts',(-48.5115549194916,62.2884122013294,
77.5228376567529));
#217757=CARTESIAN_POINT('Ctrl Pts',(-48.4883063582053,61.6652772061066,
77.1466111270594));
#217758=CARTESIAN_POINT('Ctrl Pts',(-48.476702779211,61.3630201280924,76.9381823347568));
#217759=CARTESIAN_POINT('Ctrl Pts',(-48.4651187514169,61.0741848222002,
76.7120624158843));
#217760=CARTESIAN_POINT('Ctrl Pts',(-49.0012377727522,75.078885137298,73.0255216843008));
#217761=CARTESIAN_POINT('Ctrl Pts',(-49.0326707628863,75.450923235459,72.1250428395345));
#217762=CARTESIAN_POINT('Ctrl Pts',(-49.0629964763727,75.6757768809446,
71.1705888299228));
#217763=CARTESIAN_POINT('Ctrl Pts',(-49.1091535004338,75.7777234988366,
69.7357565069057));
#217764=CARTESIAN_POINT('Ctrl Pts',(-49.1241612222689,75.7751111726431,
69.2709474013524));
#217765=CARTESIAN_POINT('Ctrl Pts',(-49.1538032208726,75.6987817530598,
68.3441468554977));
#217766=CARTESIAN_POINT('Ctrl Pts',(-49.1684042707119,75.6249225116427,
67.8835400210816));
#217767=CARTESIAN_POINT('Ctrl Pts',(-49.1917625292445,75.4526744651001,
67.1667291178721));
#217768=CARTESIAN_POINT('Ctrl Pts',(-49.2003960293311,75.3774738893031,
66.9058065330857));
#217769=CARTESIAN_POINT('Ctrl Pts',(-49.2183905535684,75.1975516952871,
66.3725072663987));
#217770=CARTESIAN_POINT('Ctrl Pts',(-49.2277486140921,75.0911654414188,
66.1010130726577));
#217771=CARTESIAN_POINT('Ctrl Pts',(-49.255312390402,74.7393198726834,65.3163913233952));
#217772=CARTESIAN_POINT('Ctrl Pts',(-49.2731546401533,74.4585712256168,
64.8206448802581));
#217773=CARTESIAN_POINT('Ctrl Pts',(-49.3142586916319,73.7122552278678,
63.7506031450283));
#217774=CARTESIAN_POINT('Ctrl Pts',(-49.3377727083167,73.2193616288411,
63.2002168272672));
#217775=CARTESIAN_POINT('Ctrl Pts',(-49.3792277925132,72.2401419089374,
62.3428777396342));
#217776=CARTESIAN_POINT('Ctrl Pts',(-49.3968018831211,71.780930515834,62.0109347506041));
#217777=CARTESIAN_POINT('Ctrl Pts',(-49.4325669000478,70.8017678731028,
61.4337113078101));
#217778=CARTESIAN_POINT('Ctrl Pts',(-49.4507406214612,70.2834231666468,
61.1906502766293));
#217779=CARTESIAN_POINT('Ctrl Pts',(-49.4870584488999,69.2096738967599,
60.8056433766568));
#217780=CARTESIAN_POINT('Ctrl Pts',(-49.5048017336833,68.6567565845836,
60.6642347640358));
#217781=CARTESIAN_POINT('Ctrl Pts',(-49.5408220038162,67.5206384453855,
60.4849875690622));
#217782=CARTESIAN_POINT('Ctrl Pts',(-49.5591749832851,66.9396760153232,
60.4496632851458));
#217783=CARTESIAN_POINT('Ctrl Pts',(-49.6153043366467,65.1754023148062,
60.5114764952306));
#217784=CARTESIAN_POINT('Ctrl Pts',(-49.651559564527,64.0109182429452,60.7840022126295));
#217785=CARTESIAN_POINT('Ctrl Pts',(-49.7211504689484,62.0145825941254,
61.6869474545517));
#217786=CARTESIAN_POINT('Ctrl Pts',(-49.7520481397383,61.1728349495882,
62.2511002479665));
#217787=CARTESIAN_POINT('Ctrl Pts',(-49.7994150585316,60.0831561780242,
63.2788274913772));
#217788=CARTESIAN_POINT('Ctrl Pts',(-49.8151103594854,59.75354956367,63.6444866168048));
#217789=CARTESIAN_POINT('Ctrl Pts',(-49.8460313342345,59.1574259710313,
64.424539596982));
#217790=CARTESIAN_POINT('Ctrl Pts',(-49.8612146371712,58.8917316289723,
64.837535753946));
#217791=CARTESIAN_POINT('Ctrl Pts',(-49.8860248707078,58.5191076372099,
65.5347662480388));
#217792=CARTESIAN_POINT('Ctrl Pts',(-49.8954937757046,58.3908722997412,
65.8062782582976));
#217793=CARTESIAN_POINT('Ctrl Pts',(-49.9050113929448,58.276355535683,66.0834535849087));
#217794=CARTESIAN_POINT('Ctrl Pts',(-48.6992141518181,61.3765724540995,
76.9087096781305));
#217795=CARTESIAN_POINT('Ctrl Pts',(-48.6491771284881,60.0508982292929,
76.0595009463134));
#217796=CARTESIAN_POINT('Ctrl Pts',(-48.5491030818342,57.8143153964347,
73.6287810246093));
#217797=CARTESIAN_POINT('Ctrl Pts',(-48.3989920118381,56.6896833063533,
68.6586256876713));
#217798=CARTESIAN_POINT('Ctrl Pts',(-48.2488809418481,58.2322800110496,
63.6554187246849));
#217799=CARTESIAN_POINT('Ctrl Pts',(-48.1488068951881,60.8521889393111,
61.2125219408773));
#217800=CARTESIAN_POINT('Ctrl Pts',(-48.0987698718642,62.4030393117053,
60.392399558577));
#217801=CARTESIAN_POINT('Ctrl Pts',(-48.6180189895515,61.3765724540995,
76.9087096781305));
#217802=CARTESIAN_POINT('Ctrl Pts',(-48.5679819662217,60.0508982292929,
76.0595009463134));
#217803=CARTESIAN_POINT('Ctrl Pts',(-48.4679079195627,57.8143153964347,
73.6287810246093));
#217804=CARTESIAN_POINT('Ctrl Pts',(-48.3177968495717,56.6896833063533,
68.6586256876713));
#217805=CARTESIAN_POINT('Ctrl Pts',(-48.1676857795814,58.2322800110496,
63.6554187246849));
#217806=CARTESIAN_POINT('Ctrl Pts',(-48.0676117329217,60.8521889393111,
61.2125219408773));
#217807=CARTESIAN_POINT('Ctrl Pts',(-48.0175747095927,62.4030393117053,
60.392399558577));
#217808=CARTESIAN_POINT('Ctrl Pts',(-48.536823827284,61.3765724540995,76.9087096781305));
#217809=CARTESIAN_POINT('Ctrl Pts',(-48.4867868039552,60.0508982292929,
76.0595009463134));
#217810=CARTESIAN_POINT('Ctrl Pts',(-48.3867127572953,57.8143153964347,
73.6287810246093));
#217811=CARTESIAN_POINT('Ctrl Pts',(-48.2366016873052,56.6896833063533,
68.6586256876713));
#217812=CARTESIAN_POINT('Ctrl Pts',(-48.086490617314,58.2322800110496,63.6554187246849));
#217813=CARTESIAN_POINT('Ctrl Pts',(-47.9864165706552,60.8521889393111,
61.2125219408773));
#217814=CARTESIAN_POINT('Ctrl Pts',(-47.9363795473253,62.4030393117053,
60.392399558577));
#217815=CARTESIAN_POINT('Ctrl Pts',(-48.4556286650124,61.3765724540995,
76.9087096781305));
#217816=CARTESIAN_POINT('Ctrl Pts',(-48.4055916416887,60.0508982292929,
76.0595009463134));
#217817=CARTESIAN_POINT('Ctrl Pts',(-48.3055175950287,57.8143153964347,
73.6287810246093));
#217818=CARTESIAN_POINT('Ctrl Pts',(-48.1554065250387,56.6896833063533,
68.6586256876713));
#217819=CARTESIAN_POINT('Ctrl Pts',(-48.0052954550424,58.2322800110496,
63.6554187246849));
#217820=CARTESIAN_POINT('Ctrl Pts',(-47.9052214083887,60.8521889393111,
61.2125219408773));
#217821=CARTESIAN_POINT('Ctrl Pts',(-47.8551843850587,62.4030393117053,
60.392399558577));
#217822=CARTESIAN_POINT('',(-48.0901869004046,62.0494599115474,60.5887241650105));
#217823=CARTESIAN_POINT('Ctrl Pts',(-48.6675364832709,61.0744133081472,
76.7063115883213));
#217824=CARTESIAN_POINT('Ctrl Pts',(-48.6312818814118,60.1377246878961,
76.0508334285312));
#217825=CARTESIAN_POINT('Ctrl Pts',(-48.5950272795537,59.3165180062426,
75.2089926210815));
#217826=CARTESIAN_POINT('Ctrl Pts',(-48.558772677695,58.6733314433729,74.2361378419511));
#217827=CARTESIAN_POINT('Ctrl Pts',(-48.5488391350847,58.4971021979518,
73.9695814902986));
#217828=CARTESIAN_POINT('Ctrl Pts',(-48.5389055924745,58.3342372318397,
73.6931898163599));
#217829=CARTESIAN_POINT('Ctrl Pts',(-48.5289720498641,58.186022422969,73.4081017822123));
#217830=CARTESIAN_POINT('Ctrl Pts',(-48.4789350265345,57.4394380330742,
71.9720625789633));
#217831=CARTESIAN_POINT('Ctrl Pts',(-48.4288980032028,57.0645606697138,
70.3153441333173));
#217832=CARTESIAN_POINT('Ctrl Pts',(-48.378860979872,57.1342214388163,68.6531170833299));
#217833=CARTESIAN_POINT('Ctrl Pts',(-48.3288239565412,57.2038822079187,
66.9908900333425));
#217834=CARTESIAN_POINT('Ctrl Pts',(-48.2787869332112,57.7180811094842,
65.3231543790137));
#217835=CARTESIAN_POINT('Ctrl Pts',(-48.2287499098812,58.6301577923322,
63.8785623558974));
#217836=CARTESIAN_POINT('Ctrl Pts',(-48.1929768542908,59.2822303519465,
62.8457776834833));
#217837=CARTESIAN_POINT('Ctrl Pts',(-48.1572037987003,60.1376805095661,
61.9270378606398));
#217838=CARTESIAN_POINT('Ctrl Pts',(-48.1214304257129,61.1391178756878,
61.1874783353119));
#217839=CARTESIAN_POINT('Ctrl Pts',(-48.111015793019,61.430664393758,60.9721718051091));
#217840=CARTESIAN_POINT('Ctrl Pts',(-48.1006011334239,61.7345839021518,
60.7720515626229));
#217841=CARTESIAN_POINT('Ctrl Pts',(-48.090186439096,62.0494598503368,60.5887240860842));
#217842=CARTESIAN_POINT('',(-47.8901874902887,62.0494598737417,60.588724072085));
#217843=CARTESIAN_POINT('',(-48.0901862140809,62.0494598738326,60.5887240724044));
#217844=CARTESIAN_POINT('Ctrl Pts',(-48.4675451203219,61.0746269353901,
76.7064610762623));
#217845=CARTESIAN_POINT('Ctrl Pts',(-48.4374727537661,60.2976378300801,
76.1627715126034));
#217846=CARTESIAN_POINT('Ctrl Pts',(-48.4076478871442,59.6067484297961,
75.4956452737586));
#217847=CARTESIAN_POINT('Ctrl Pts',(-48.3478038746688,58.4441481286654,
73.9693330989566));
#217848=CARTESIAN_POINT('Ctrl Pts',(-48.3182577310618,57.9861362652872,
73.118218239834));
#217849=CARTESIAN_POINT('Ctrl Pts',(-48.2515859642631,57.2658215968254,
71.0669096930218));
#217850=CARTESIAN_POINT('Ctrl Pts',(-48.2150542464285,57.0838374275983,
69.855443032875));
#217851=CARTESIAN_POINT('Ctrl Pts',(-48.1419859937645,57.1855554964561,
67.4281199427107));
#217852=CARTESIAN_POINT('Ctrl Pts',(-48.1054696631336,57.4774766013662,
66.2128718196243));
#217853=CARTESIAN_POINT('Ctrl Pts',(-48.0390051710523,58.3991305558005,
64.1561131800471));
#217854=CARTESIAN_POINT('Ctrl Pts',(-48.0094233078613,58.959999203317,63.3004156653558));
#217855=CARTESIAN_POINT('Ctrl Pts',(-47.9496630882316,60.3396764638368,
61.7718652461384));
#217856=CARTESIAN_POINT('Ctrl Pts',(-47.9198152757014,61.1536715706108,
61.1102710786235));
#217857=CARTESIAN_POINT('Ctrl Pts',(-47.8901874908167,62.0494598739167,
60.5887240723555));
#217858=CARTESIAN_POINT('Ctrl Pts',(-63.7104920345709,57.8065696683908,
74.8099293892527));
#217859=CARTESIAN_POINT('Ctrl Pts',(-63.6718652093945,57.1031312732521,
73.6224666938169));
#217860=CARTESIAN_POINT('Ctrl Pts',(-63.5946115590417,56.1796658359588,
70.9619911069131));
#217861=CARTESIAN_POINT('Ctrl Pts',(-63.4787310835129,56.4635561166055,
66.7467220222677));
#217862=CARTESIAN_POINT('Ctrl Pts',(-63.3628506079829,58.3717651523206,
62.9775246456951));
#217863=CARTESIAN_POINT('Ctrl Pts',(-63.2469701324539,61.6008831507443,
60.2533615179501));
#217864=CARTESIAN_POINT('Ctrl Pts',(-63.1310896569249,65.6376592981465,
59.007288209015));
#217865=CARTESIAN_POINT('Ctrl Pts',(-63.0152091813959,69.8404311589655,
59.4373596262818));
#217866=CARTESIAN_POINT('Ctrl Pts',(-62.8993287058659,73.5411595353312,
61.4752179418165));
#217867=CARTESIAN_POINT('Ctrl Pts',(-62.7834482303369,76.1516039658375,
64.7969396843518));
#217868=CARTESIAN_POINT('Ctrl Pts',(-62.6675677548079,77.2568279536785,
68.8745291515198));
#217869=CARTESIAN_POINT('Ctrl Pts',(-62.5516872792779,76.6811533646194,
73.0598433065362));
#217870=CARTESIAN_POINT('Ctrl Pts',(-62.4358068037489,74.5160851144003,
76.6876160812524));
#217871=CARTESIAN_POINT('Ctrl Pts',(-62.3199263282199,71.1057661783553,
79.1812039750165));
#217872=CARTESIAN_POINT('Ctrl Pts',(-62.2040458526899,66.9922752255877,
80.1442449974989));
#217873=CARTESIAN_POINT('Ctrl Pts',(-62.0881653771609,62.8294618635471,
79.4236613850277));
#217874=CARTESIAN_POINT('Ctrl Pts',(-61.9722849016309,59.2790156194285,
77.1339916933007));
#217875=CARTESIAN_POINT('Ctrl Pts',(-61.8564044261019,56.9052887454224,
73.6391846088869));
#217876=CARTESIAN_POINT('Ctrl Pts',(-61.7405239505729,56.0855910260969,
69.4947484013197));
#217877=CARTESIAN_POINT('Ctrl Pts',(-61.6246434750429,56.9502154506322,
65.3594515033776));
#217878=CARTESIAN_POINT('Ctrl Pts',(-61.5087629995139,59.361727818425,61.8906096318565));
#217879=CARTESIAN_POINT('Ctrl Pts',(-61.3928825239839,62.9368122467912,
59.6396038211846));
#217880=CARTESIAN_POINT('Ctrl Pts',(-61.2770020484549,67.1072001829157,
58.9642370379884));
#217881=CARTESIAN_POINT('Ctrl Pts',(-61.1611215729249,71.209998102294,59.9718605105236));
#217882=CARTESIAN_POINT('Ctrl Pts',(-61.0452410973959,74.5930560815078,
62.5023099842148));
#217883=CARTESIAN_POINT('Ctrl Pts',(-60.9293606218659,76.7186286489653,
66.1533642278691));
#217884=CARTESIAN_POINT('Ctrl Pts',(-60.8134801463369,77.2488507637066,
70.3446790977719));
#217885=CARTESIAN_POINT('Ctrl Pts',(-60.6975996708069,76.0994423031657,
74.4100346812925));
#217886=CARTESIAN_POINT('Ctrl Pts',(-60.5817191952779,73.4531045980525,
77.7032326073399));
#217887=CARTESIAN_POINT('Ctrl Pts',(-60.4658387197479,69.7304796018871,
79.7008108830386));
#217888=CARTESIAN_POINT('Ctrl Pts',(-60.3499582442189,65.5232878073241,
80.0852494781353));
#217889=CARTESIAN_POINT('Ctrl Pts',(-60.2340777686899,61.5002728036194,
78.7954409227264));
#217890=CARTESIAN_POINT('Ctrl Pts',(-60.1181972931599,58.3009028215076,
76.0364034914597));
#217891=CARTESIAN_POINT('Ctrl Pts',(-60.0023168176309,56.433725669026,72.2466930393406));
#217892=CARTESIAN_POINT('Ctrl Pts',(-59.8864363421009,56.1955337939067,
68.0286934589439));
#217893=CARTESIAN_POINT('Ctrl Pts',(-59.7705558665719,57.624188386514,64.0528662639259));
#217894=CARTESIAN_POINT('Ctrl Pts',(-59.6546753910419,60.4926012496316,
60.9511790655875));
#217895=CARTESIAN_POINT('Ctrl Pts',(-59.5387949155129,64.3448310315735,
59.2166527507834));
#217896=CARTESIAN_POINT('Ctrl Pts',(-59.4229144399829,68.5685562369575,
59.1249945869912));
#217897=CARTESIAN_POINT('Ctrl Pts',(-59.3070339644539,72.4924052498076,
60.690773867081));
#217898=CARTESIAN_POINT('Ctrl Pts',(-59.1911534889249,75.4926725200354,
63.6651060840354));
#217899=CARTESIAN_POINT('Ctrl Pts',(-59.0752730133949,77.0924581103469,
67.575213741715));
#217900=CARTESIAN_POINT('Ctrl Pts',(-58.9593925378659,77.0374721262134,
71.7995755125809));
#217901=CARTESIAN_POINT('Ctrl Pts',(-58.8435120623359,75.3364547264357,
75.6667185969866));
#217902=CARTESIAN_POINT('Ctrl Pts',(-58.7276315868069,72.2597868531839,
78.5619509930676));
#217903=CARTESIAN_POINT('Ctrl Pts',(-58.6117511112779,68.2965125094352,
80.0250683177526));
#217904=CARTESIAN_POINT('Ctrl Pts',(-58.4958706357479,64.076603999578,79.8235044369148));
#217905=CARTESIAN_POINT('Ctrl Pts',(-58.3799901602189,60.2708262663669,
77.9892984302229));
#217906=CARTESIAN_POINT('Ctrl Pts',(-58.2641096846899,57.4841171366094,
74.8140018998644));
#217907=CARTESIAN_POINT('Ctrl Pts',(-58.1482292091609,56.1594309505501,
70.8023361189094));
#217908=CARTESIAN_POINT('Ctrl Pts',(-58.0323487336309,56.5073298688805,
66.5919653309315));
#217909=CARTESIAN_POINT('Ctrl Pts',(-57.9164682581019,58.4725144941193,
62.8521384340947));
#217910=CARTESIAN_POINT('Ctrl Pts',(-57.8005877825729,61.7426138472405,
60.1773102058845));
#217911=CARTESIAN_POINT('Ctrl Pts',(-57.6847073070439,65.7978375109195,
58.992651239347));
#217912=CARTESIAN_POINT('Ctrl Pts',(-57.5688268315149,69.9935976079059,
59.4864660203555));
#217913=CARTESIAN_POINT('Ctrl Pts',(-57.4529463559859,73.6629676456614,
61.5802614638165));
#217914=CARTESIAN_POINT('Ctrl Pts',(-57.3370658804569,76.2226921395821,
64.941223576645));
#217915=CARTESIAN_POINT('Ctrl Pts',(-57.2211854049279,77.2658965208973,
69.0351190986164));
#217916=CARTESIAN_POINT('Ctrl Pts',(-57.1053049293989,76.6267608625964,
73.2112130953809));
#217917=CARTESIAN_POINT('Ctrl Pts',(-56.9894244538699,74.4068773602934,
76.8057053079185));
#217918=CARTESIAN_POINT('Ctrl Pts',(-56.8735439783409,70.9591020322142,
79.2472413050085));
#217919=CARTESIAN_POINT('Ctrl Pts',(-56.7576635028119,66.8314672593026,
80.1477364670454));
#217920=CARTESIAN_POINT('Ctrl Pts',(-56.6417830272829,62.6800711209345,
79.3640414392399));
#217921=CARTESIAN_POINT('Ctrl Pts',(-56.5259025517539,59.1647873166941,
77.0207765453072));
#217922=CARTESIAN_POINT('Ctrl Pts',(-56.4100220762249,56.844382791141,73.4902227664913));
#217923=CARTESIAN_POINT('Ctrl Pts',(-56.3327684258729,56.3399124253312,
70.7195859421522));
#217924=CARTESIAN_POINT('Ctrl Pts',(-56.2941416006959,56.3683493792519,
69.3397002336784));
#217925=CARTESIAN_POINT('Ctrl Pts',(-63.4863639242949,58.1769980971959,
74.5904921130554));
#217926=CARTESIAN_POINT('Ctrl Pts',(-63.4477370991189,57.5029187523924,
73.4525899438659));
#217927=CARTESIAN_POINT('Ctrl Pts',(-63.3704834487659,56.6179955221206,
70.9031532726741));
#217928=CARTESIAN_POINT('Ctrl Pts',(-63.2546029732369,56.8900372185927,
66.863814728757));
#217929=CARTESIAN_POINT('Ctrl Pts',(-63.1387224977069,58.7186043048254,
63.2519304250262));
#217930=CARTESIAN_POINT('Ctrl Pts',(-63.0228420221779,61.8129502485881,
60.6414643074804));
#217931=CARTESIAN_POINT('Ctrl Pts',(-62.9069615466489,65.6812455241418,
59.4473977261369));
#217932=CARTESIAN_POINT('Ctrl Pts',(-62.7910810711199,69.7086084345096,
59.8595194715137));
#217933=CARTESIAN_POINT('Ctrl Pts',(-62.6752005955899,73.2548813938479,
61.8123247315615));
#217934=CARTESIAN_POINT('Ctrl Pts',(-62.5593201200609,75.7563750335582,
64.9954094640758));
#217935=CARTESIAN_POINT('Ctrl Pts',(-62.4434396445319,76.8154708502427,
68.9028146546496));
#217936=CARTESIAN_POINT('Ctrl Pts',(-62.3275591690019,76.2638228985589,
72.9134484825934));
#217937=CARTESIAN_POINT('Ctrl Pts',(-62.2116786934729,74.1891170001427,
76.3898107511058));
#217938=CARTESIAN_POINT('Ctrl Pts',(-62.0957982179439,70.9211328100948,
78.7793250358796));
#217939=CARTESIAN_POINT('Ctrl Pts',(-61.9799177424139,66.9793245359562,
79.7021721052773));
#217940=CARTESIAN_POINT('Ctrl Pts',(-61.8640372668849,62.9902523968414,
79.0116631243529));
#217941=CARTESIAN_POINT('Ctrl Pts',(-61.7481567913549,59.5879893208676,
76.8175562113823));
#217942=CARTESIAN_POINT('Ctrl Pts',(-61.6322763158259,57.3133334774654,
73.4686101118191));
#217943=CARTESIAN_POINT('Ctrl Pts',(-61.5163958402969,56.5278470647294,
69.4971481292357));
#217944=CARTESIAN_POINT('Ctrl Pts',(-61.4005153647669,57.3563850996458,
65.5344440135604));
#217945=CARTESIAN_POINT('Ctrl Pts',(-61.2846348892379,59.667249402905,62.210379430011));
#217946=CARTESIAN_POINT('Ctrl Pts',(-61.1687544137079,63.0931223517737,
60.0533227033746));
#217947=CARTESIAN_POINT('Ctrl Pts',(-61.0528739381789,67.0894529288327,
59.4061433599309));
#217948=CARTESIAN_POINT('Ctrl Pts',(-60.9369934626489,71.0210144592654,
60.3717121643543));
#217949=CARTESIAN_POINT('Ctrl Pts',(-60.8211129871199,74.2628754691667,
62.7965495560487));
#217950=CARTESIAN_POINT('Ctrl Pts',(-60.7052325115899,76.2997340960325,
66.2952216066778));
#217951=CARTESIAN_POINT('Ctrl Pts',(-60.5893520360609,76.8078266001889,
70.3116057007245));
#217952=CARTESIAN_POINT('Ctrl Pts',(-60.4734715605309,75.7063904156562,
74.2072876070264));
#217953=CARTESIAN_POINT('Ctrl Pts',(-60.3575910850019,73.1705015606764,
77.3630390070701));
#217954=CARTESIAN_POINT('Ctrl Pts',(-60.2417106094719,69.6032458696127,
79.277245374799));
#217955=CARTESIAN_POINT('Ctrl Pts',(-60.1258301339429,65.5716474980321,
79.6456388518812));
#217956=CARTESIAN_POINT('Ctrl Pts',(-60.0099496584129,61.7165390243107,
78.4096623797983));
#217957=CARTESIAN_POINT('Ctrl Pts',(-59.8940691828839,58.6506995190535,
75.765777489781));
#217958=CARTESIAN_POINT('Ctrl Pts',(-59.7781887073549,56.86145178922,72.1342362543012));
#217959=CARTESIAN_POINT('Ctrl Pts',(-59.6623082318249,56.6332012071813,
68.0922811759416));
#217960=CARTESIAN_POINT('Ctrl Pts',(-59.5464277562959,58.002228770078,64.2823910573551));
#217961=CARTESIAN_POINT('Ctrl Pts',(-59.4305472807659,60.7509241451938,
61.3101573992297));
#217962=CARTESIAN_POINT('Ctrl Pts',(-59.3146668052369,64.4423753730412,
59.6480241265653));
#217963=CARTESIAN_POINT('Ctrl Pts',(-59.1987863297069,68.4898171088944,
59.5601914529124));
#217964=CARTESIAN_POINT('Ctrl Pts',(-59.0829058541779,72.2498984322556,
61.0606205999848));
#217965=CARTESIAN_POINT('Ctrl Pts',(-58.9670253786489,75.1249450741959,
63.9108146267734));
#217966=CARTESIAN_POINT('Ctrl Pts',(-58.8511449031189,76.6579612274189,
67.6577281109137));
#217967=CARTESIAN_POINT('Ctrl Pts',(-58.7352644275899,76.6052701653223,
71.7057798442352));
#217968=CARTESIAN_POINT('Ctrl Pts',(-58.6193839520599,74.9752472631463,
75.4115219456312));
#217969=CARTESIAN_POINT('Ctrl Pts',(-58.5035034765309,72.0269887112709,
78.1859175005157));
#217970=CARTESIAN_POINT('Ctrl Pts',(-58.3876230010019,68.2291275319825,
79.5879694419675));
#217971=CARTESIAN_POINT('Ctrl Pts',(-58.2717425254719,64.1853431961836,
79.394818130247));
#217972=CARTESIAN_POINT('Ctrl Pts',(-58.1558620499429,60.5384052715379,
77.6371654462714));
#217973=CARTESIAN_POINT('Ctrl Pts',(-58.0399815744139,57.8680036026363,
74.5943946513582));
#217974=CARTESIAN_POINT('Ctrl Pts',(-57.9241010988849,56.5986051698264,
70.7501617236546));
#217975=CARTESIAN_POINT('Ctrl Pts',(-57.8082206233549,56.9319840080419,
66.7155170386891));
#217976=CARTESIAN_POINT('Ctrl Pts',(-57.6923401478259,58.8151487226244,
63.1317773939326));
#217977=CARTESIAN_POINT('Ctrl Pts',(-57.5764596722969,61.9487656031238,
60.5685871103211));
#217978=CARTESIAN_POINT('Ctrl Pts',(-57.4605791967679,65.8347384603639,
59.4333716522234));
#217979=CARTESIAN_POINT('Ctrl Pts',(-57.3446987212389,69.8553822533185,
59.906576337004));
#217980=CARTESIAN_POINT('Ctrl Pts',(-57.2288182457099,73.3716056610648,
61.9129841055396));
#217981=CARTESIAN_POINT('Ctrl Pts',(-57.1129377701809,75.8244962363713,
65.1336714529827));
#217982=CARTESIAN_POINT('Ctrl Pts',(-56.9970572946509,76.8241609272865,
69.0567021408465));
#217983=CARTESIAN_POINT('Ctrl Pts',(-56.8811768191219,76.2117005487124,
73.058500627591));
#217984=CARTESIAN_POINT('Ctrl Pts',(-56.7652963435929,74.0844671944947,
76.502971347812));
#217985=CARTESIAN_POINT('Ctrl Pts',(-56.6494158680649,70.7805899107851,
78.8426061994355));
#217986=CARTESIAN_POINT('Ctrl Pts',(-56.5335353925359,66.8252281299281,
79.705517853136));
#217987=CARTESIAN_POINT('Ctrl Pts',(-56.4176549170069,62.8470966996323,
78.9545315059017));
#217988=CARTESIAN_POINT('Ctrl Pts',(-56.3017744414779,59.4785285066753,
76.7090662664087));
#217989=CARTESIAN_POINT('Ctrl Pts',(-56.1858939659489,57.2549695240061,
73.3258654140387));
#217990=CARTESIAN_POINT('Ctrl Pts',(-56.1086403155959,56.7715539811408,
70.6708652489211));
#217991=CARTESIAN_POINT('Ctrl Pts',(-56.0700134904199,56.7988040763871,
69.3485711280681));
#217992=CARTESIAN_POINT('Ctrl Pts',(-63.2622358140189,58.547426526001,74.3710548368581));
#217993=CARTESIAN_POINT('Ctrl Pts',(-63.2236089888419,57.9027062315234,
73.282713193911));
#217994=CARTESIAN_POINT('Ctrl Pts',(-63.1463553384899,57.0563252082828,
70.8443154384342));
#217995=CARTESIAN_POINT('Ctrl Pts',(-63.0304748629609,57.3165183205799,
66.9809074352464));
#217996=CARTESIAN_POINT('Ctrl Pts',(-62.9145943874309,59.0654434573398,
63.5263362043602));
#217997=CARTESIAN_POINT('Ctrl Pts',(-62.7987139119019,62.0250173464219,
61.0295670970088));
#217998=CARTESIAN_POINT('Ctrl Pts',(-62.6828334363729,65.7248317501465,
59.8875072432628));
#217999=CARTESIAN_POINT('Ctrl Pts',(-62.5669529608439,69.5767857100507,
60.2816793167476));
#218000=CARTESIAN_POINT('Ctrl Pts',(-62.4510724853139,72.9686032523646,
62.1494315213011));
#218001=CARTESIAN_POINT('Ctrl Pts',(-62.3351920097849,75.3611461012774,
65.1938792437982));
#218002=CARTESIAN_POINT('Ctrl Pts',(-62.2193115342559,76.3741137468067,
68.9311001577751));
#218003=CARTESIAN_POINT('Ctrl Pts',(-62.1034310587259,75.8464924324996,
72.7670536586459));
#218004=CARTESIAN_POINT('Ctrl Pts',(-61.9875505831969,73.862148885889,76.0920054209542));
#218005=CARTESIAN_POINT('Ctrl Pts',(-61.8716701076679,70.73649944184,78.3774460967396));
#218006=CARTESIAN_POINT('Ctrl Pts',(-61.7557896321379,66.9663738463322,
79.2600992130555));
#218007=CARTESIAN_POINT('Ctrl Pts',(-61.6399091566089,63.1510429301467,
78.5996648636749));
#218008=CARTESIAN_POINT('Ctrl Pts',(-61.5240286810789,59.8969630223145,
76.5011207294713));
#218009=CARTESIAN_POINT('Ctrl Pts',(-61.4081482055499,57.7213782095142,
73.2980356147634));
#218010=CARTESIAN_POINT('Ctrl Pts',(-61.2922677300209,56.9701031033569,
69.4995478571637));
#218011=CARTESIAN_POINT('Ctrl Pts',(-61.1763872544909,57.7625547486447,
65.7094365237527));
#218012=CARTESIAN_POINT('Ctrl Pts',(-61.0605067789619,59.9727709873796,
62.5301492281785));
#218013=CARTESIAN_POINT('Ctrl Pts',(-60.9446263034319,63.2494324567334,
60.4670415855671));
#218014=CARTESIAN_POINT('Ctrl Pts',(-60.8287458279029,67.0717056747189,
59.8480496818693));
#218015=CARTESIAN_POINT('Ctrl Pts',(-60.7128653523729,70.8320308162221,
60.7715638181682));
#218016=CARTESIAN_POINT('Ctrl Pts',(-60.5969848768439,73.9326948568119,
63.090789127866));
#218017=CARTESIAN_POINT('Ctrl Pts',(-60.4811044013139,75.8808395430932,
66.4370789854654));
#218018=CARTESIAN_POINT('Ctrl Pts',(-60.3652239257849,76.3668024366729,
70.2785323036529));
#218019=CARTESIAN_POINT('Ctrl Pts',(-60.2493434502549,75.3133385281575,
74.004540532737));
#218020=CARTESIAN_POINT('Ctrl Pts',(-60.1334629747259,72.887898523321,77.0228454067829));
#218021=CARTESIAN_POINT('Ctrl Pts',(-60.0175824991959,69.4760121373647,
78.8536798665508));
#218022=CARTESIAN_POINT('Ctrl Pts',(-59.9017020236669,65.6200071887684,
79.2060282256323));
#218023=CARTESIAN_POINT('Ctrl Pts',(-59.7858215481369,61.9328052450312,
78.023883836878));
#218024=CARTESIAN_POINT('Ctrl Pts',(-59.6699410726079,59.0004962166207,
75.4951514881296));
#218025=CARTESIAN_POINT('Ctrl Pts',(-59.5540605970789,57.2891779094226,
72.0217794692935));
#218026=CARTESIAN_POINT('Ctrl Pts',(-59.4381801215489,57.0708686204521,
68.1558688929745));
#218027=CARTESIAN_POINT('Ctrl Pts',(-59.3222996460199,58.3802691536199,
64.5119158508119));
#218028=CARTESIAN_POINT('Ctrl Pts',(-59.2064191704899,61.0092470407258,
61.6691357328929));
#218029=CARTESIAN_POINT('Ctrl Pts',(-59.0905386949609,64.5399197144825,
60.0793955023591));
#218030=CARTESIAN_POINT('Ctrl Pts',(-58.9746582194309,68.4110779807901,
59.9953883188285));
#218031=CARTESIAN_POINT('Ctrl Pts',(-58.8587777439019,72.0073916146724,
61.4304673328671));
#218032=CARTESIAN_POINT('Ctrl Pts',(-58.7428972683729,74.7572176283345,
64.1565231694807));
#218033=CARTESIAN_POINT('Ctrl Pts',(-58.6270167928429,76.2234643444835,
67.7402424800746));
#218034=CARTESIAN_POINT('Ctrl Pts',(-58.5111363173139,76.1730682044392,
71.6119841758516));
#218035=CARTESIAN_POINT('Ctrl Pts',(-58.3952558417839,74.6140397998802,
75.1563252942433));
#218036=CARTESIAN_POINT('Ctrl Pts',(-58.2793753662549,71.7941905693904,
77.8098840079436));
#218037=CARTESIAN_POINT('Ctrl Pts',(-58.1634948907259,68.1617425545688,
79.1508705661768));
#218038=CARTESIAN_POINT('Ctrl Pts',(-58.0476144151959,64.2940823928253,
78.9661318235942));
#218039=CARTESIAN_POINT('Ctrl Pts',(-57.9317339396669,60.8059842767521,
77.2850324623464));
#218040=CARTESIAN_POINT('Ctrl Pts',(-57.8158534641379,58.2518900686915,
74.3747874028885));
#218041=CARTESIAN_POINT('Ctrl Pts',(-57.6999729886089,57.0377793891086,
70.6979873284379));
#218042=CARTESIAN_POINT('Ctrl Pts',(-57.5840925130789,57.3566381471987,
66.8390687464839));
#218043=CARTESIAN_POINT('Ctrl Pts',(-57.4682120375499,59.157782951098,63.4114163537943));
#218044=CARTESIAN_POINT('Ctrl Pts',(-57.3523315620209,62.1549173589786,
60.9598640147741));
#218045=CARTESIAN_POINT('Ctrl Pts',(-57.2364510864919,65.8716394097845,
59.8740920651051));
#218046=CARTESIAN_POINT('Ctrl Pts',(-57.1205706109629,69.7171668986981,
60.326686653654));
#218047=CARTESIAN_POINT('Ctrl Pts',(-57.0046901354339,73.0802436764493,
62.2457067472407));
#218048=CARTESIAN_POINT('Ctrl Pts',(-56.8888096599039,75.4263003331489,
65.3261193292961));
#218049=CARTESIAN_POINT('Ctrl Pts',(-56.7729291843749,76.3824253336746,
69.0782851830545));
#218050=CARTESIAN_POINT('Ctrl Pts',(-56.6570487088459,75.7966402348365,
72.9057881597825));
#218051=CARTESIAN_POINT('Ctrl Pts',(-56.5411682333169,73.7620570287082,
76.2002373876932));
#218052=CARTESIAN_POINT('Ctrl Pts',(-56.4252877577879,70.6020777893704,
78.4379710938565));
#218053=CARTESIAN_POINT('Ctrl Pts',(-56.3094072822599,66.8189890005654,
79.2632992392271));
#218054=CARTESIAN_POINT('Ctrl Pts',(-56.1935268067309,63.0141222783363,
78.5450215725671));
#218055=CARTESIAN_POINT('Ctrl Pts',(-56.0776463312019,59.7922696966654,
76.3973559875148));
#218056=CARTESIAN_POINT('Ctrl Pts',(-55.9617658556729,57.6655562568715,
73.1615080615852));
#218057=CARTESIAN_POINT('Ctrl Pts',(-55.8845122053199,57.2031955369423,
70.6221445556835));
#218058=CARTESIAN_POINT('Ctrl Pts',(-55.8458853801439,57.2292587735241,
69.3574420224531));
#218059=CARTESIAN_POINT('Ctrl Pts',(-63.0381077037429,58.9178549548062,
74.1516175606608));
#218060=CARTESIAN_POINT('Ctrl Pts',(-62.9994808785659,58.3024937106637,
73.11283644396));
#218061=CARTESIAN_POINT('Ctrl Pts',(-62.9222272282139,57.4946548944447,
70.7854776041952));
#218062=CARTESIAN_POINT('Ctrl Pts',(-62.8063467526839,57.7429994225583,
67.098000141731));
#218063=CARTESIAN_POINT('Ctrl Pts',(-62.6904662771549,59.4122826098446,
63.8007419836913));
#218064=CARTESIAN_POINT('Ctrl Pts',(-62.5745858016259,62.2370844442565,
61.4176698865354));
#218065=CARTESIAN_POINT('Ctrl Pts',(-62.4587053260969,65.7684179761418,
60.3276167603848));
#218066=CARTESIAN_POINT('Ctrl Pts',(-62.3428248505679,69.4449629855937,
60.7038391619823));
#218067=CARTESIAN_POINT('Ctrl Pts',(-62.2269443750379,72.6823251108832,
62.4865383110415));
#218068=CARTESIAN_POINT('Ctrl Pts',(-62.1110638995089,74.9659171689976,
65.3923490235231));
#218069=CARTESIAN_POINT('Ctrl Pts',(-61.9951834239799,75.9327566433709,
68.959385660905));
#218070=CARTESIAN_POINT('Ctrl Pts',(-61.8793029484499,75.429161966439,72.6206588347031));
#218071=CARTESIAN_POINT('Ctrl Pts',(-61.7634224729209,73.5351807716313,
75.7942000908075));
#218072=CARTESIAN_POINT('Ctrl Pts',(-61.6475419973919,70.5518660735791,
77.9755671576036));
#218073=CARTESIAN_POINT('Ctrl Pts',(-61.5316615218619,66.9534231567007,
78.8180263208339));
#218074=CARTESIAN_POINT('Ctrl Pts',(-61.4157810463329,63.3118334634422,
78.1876666029973));
#218075=CARTESIAN_POINT('Ctrl Pts',(-61.2999005708029,60.2059367237536,
76.1846852475529));
#218076=CARTESIAN_POINT('Ctrl Pts',(-61.1840200952739,58.1294229415569,
73.1274611176965));
#218077=CARTESIAN_POINT('Ctrl Pts',(-61.0681396197439,57.4123591419893,
69.5019475850797));
#218078=CARTESIAN_POINT('Ctrl Pts',(-60.9522591442149,58.1687243976584,
65.8844290339353));
#218079=CARTESIAN_POINT('Ctrl Pts',(-60.8363786686859,60.2782925718688,
62.8499190263368));
#218080=CARTESIAN_POINT('Ctrl Pts',(-60.7204981931559,63.4057425617159,
60.8807604677571));
#218081=CARTESIAN_POINT('Ctrl Pts',(-60.6046177176269,67.0539584206267,
60.2899560038079));
#218082=CARTESIAN_POINT('Ctrl Pts',(-60.4887372420969,70.6430471731958,
61.1714154719933));
#218083=CARTESIAN_POINT('Ctrl Pts',(-60.3728567665679,73.6025142444707,
63.3850286996998));
#218084=CARTESIAN_POINT('Ctrl Pts',(-60.2569762910379,75.4619449901604,
66.5789363642741));
#218085=CARTESIAN_POINT('Ctrl Pts',(-60.1410958155089,75.9257782731553,
70.2454589066056));
#218086=CARTESIAN_POINT('Ctrl Pts',(-60.0252153399789,74.9202866406472,
73.8017934584711));
#218087=CARTESIAN_POINT('Ctrl Pts',(-59.9093348644499,72.6052954859446,
76.6826518065131));
#218088=CARTESIAN_POINT('Ctrl Pts',(-59.7934543889199,69.34877840509,78.4301143583121));
#218089=CARTESIAN_POINT('Ctrl Pts',(-59.6775739133909,65.6683668794744,
78.7664175993805));
#218090=CARTESIAN_POINT('Ctrl Pts',(-59.5616934378609,62.149071465724,77.6381052939462));
#218091=CARTESIAN_POINT('Ctrl Pts',(-59.4458129623319,59.3502929141666,
75.224525486451));
#218092=CARTESIAN_POINT('Ctrl Pts',(-59.3299324868019,57.7169040296169,
71.9093226842531));
#218093=CARTESIAN_POINT('Ctrl Pts',(-59.2140520112729,57.5085360337358,
68.219456609976));
#218094=CARTESIAN_POINT('Ctrl Pts',(-59.0981715357439,58.7583095371751,
64.7414406442363));
#218095=CARTESIAN_POINT('Ctrl Pts',(-58.9822910602139,61.2675699362972,
62.0281140665389));
#218096=CARTESIAN_POINT('Ctrl Pts',(-58.8664105846849,64.6374640559506,
60.5107668781401));
#218097=CARTESIAN_POINT('Ctrl Pts',(-58.7505301091549,68.3323388527351,
60.4305851847563));
#218098=CARTESIAN_POINT('Ctrl Pts',(-58.6346496336259,71.7648847971204,
61.800314065771));
#218099=CARTESIAN_POINT('Ctrl Pts',(-58.5187691580959,74.3894901824946,
64.4022317122195));
#218100=CARTESIAN_POINT('Ctrl Pts',(-58.4028886825669,75.7889674615547,
67.8227568492751));
#218101=CARTESIAN_POINT('Ctrl Pts',(-58.2870082070379,75.740866243548,71.5181885075058));
#218102=CARTESIAN_POINT('Ctrl Pts',(-58.1711277315079,74.2528323365911,
74.9011286428881));
#218103=CARTESIAN_POINT('Ctrl Pts',(-58.0552472559789,71.5613924274766,
77.4338505153925));
#218104=CARTESIAN_POINT('Ctrl Pts',(-57.9393667804499,68.0943575771148,
78.7137716903922));
#218105=CARTESIAN_POINT('Ctrl Pts',(-57.8234863049199,64.4028215894282,
78.5374455169307));
#218106=CARTESIAN_POINT('Ctrl Pts',(-57.7076058293909,61.0735632819335,
76.9328994783959));
#218107=CARTESIAN_POINT('Ctrl Pts',(-57.5917253538619,58.6357765347184,
74.1551801543823));
#218108=CARTESIAN_POINT('Ctrl Pts',(-57.4758448783329,57.4769536083849,
70.6458129331832));
#218109=CARTESIAN_POINT('Ctrl Pts',(-57.3599644028029,57.7812922863604,
66.9626204542406));
#218110=CARTESIAN_POINT('Ctrl Pts',(-57.2440839272739,59.5004171796032,
63.6910553136322));
#218111=CARTESIAN_POINT('Ctrl Pts',(-57.1282034517449,62.3610691148619,
61.3511409192107));
#218112=CARTESIAN_POINT('Ctrl Pts',(-57.0123229762159,65.908540359229,60.3148124779815));
#218113=CARTESIAN_POINT('Ctrl Pts',(-56.8964425006869,69.5789515441067,
60.7467969703095));
#218114=CARTESIAN_POINT('Ctrl Pts',(-56.7805620251579,72.7888816918543,
62.5784293889601));
#218115=CARTESIAN_POINT('Ctrl Pts',(-56.6646815496279,75.0281044299382,
65.5185672056338));
#218116=CARTESIAN_POINT('Ctrl Pts',(-56.5488010740989,75.9406897400636,
69.0998682252856));
#218117=CARTESIAN_POINT('Ctrl Pts',(-56.4329205985699,75.3815799209528,
72.7530756919932));
#218118=CARTESIAN_POINT('Ctrl Pts',(-56.3170401230409,73.439646862909,75.8975034275876));
#218119=CARTESIAN_POINT('Ctrl Pts',(-56.2011596475119,70.4235656679413,
78.0333359882836));
#218120=CARTESIAN_POINT('Ctrl Pts',(-56.0852791719829,66.81274987119,78.8210806253173));
#218121=CARTESIAN_POINT('Ctrl Pts',(-55.9693986964549,63.1811478570336,
78.1355116392275));
#218122=CARTESIAN_POINT('Ctrl Pts',(-55.8535182209259,60.1060108866471,
76.0856457086154));
#218123=CARTESIAN_POINT('Ctrl Pts',(-55.7376377453969,58.0761429897366,
72.9971507091326));
#218124=CARTESIAN_POINT('Ctrl Pts',(-55.6603840950439,57.6348370927523,
70.5734238624516));
#218125=CARTESIAN_POINT('Ctrl Pts',(-55.6217572698679,57.6597134706593,
69.3663129168428));
#218126=CARTESIAN_POINT('',(-63.5337774910882,56.4405479536543,69.9703292528641));
#218127=CARTESIAN_POINT('',(-63.5337571161032,56.4405871136771,69.9703282277341));
#218128=CARTESIAN_POINT('Ctrl Pts',(-63.5337978660731,56.4405087936315,
69.970330277994));
#218129=CARTESIAN_POINT('Ctrl Pts',(-63.5202231218634,56.4206513278838,
69.4838986812489));
#218130=CARTESIAN_POINT('Ctrl Pts',(-63.5066190833876,56.4354746233135,
68.9966731918193));
#218131=CARTESIAN_POINT('Ctrl Pts',(-63.4794168880834,56.5330349183312,
68.0400039530818));
#218132=CARTESIAN_POINT('Ctrl Pts',(-63.465861497201,56.6139662085722,67.5715749189794));
#218133=CARTESIAN_POINT('Ctrl Pts',(-63.425565687372,56.9527669983538,66.1903259139352));
#218134=CARTESIAN_POINT('Ctrl Pts',(-63.3996267041034,57.3049409708213,
65.3059259002616));
#218135=CARTESIAN_POINT('Ctrl Pts',(-63.3570313944311,58.048595780408,63.9991853257494));
#218136=CARTESIAN_POINT('Ctrl Pts',(-63.3411184424965,58.3625411606416,
63.539031567641));
#218137=CARTESIAN_POINT('Ctrl Pts',(-63.3110423001554,59.0356488652194,
62.7067648440937));
#218138=CARTESIAN_POINT('Ctrl Pts',(-63.2968122207668,59.3886727116809,
62.3318121573921));
#218139=CARTESIAN_POINT('Ctrl Pts',(-63.2645159255659,60.2394786389348,
61.5544994963403));
#218140=CARTESIAN_POINT('Ctrl Pts',(-63.2463846911154,60.7497831421837,
61.1690009106554));
#218141=CARTESIAN_POINT('Ctrl Pts',(-63.2103027884577,61.8298654770057,
60.5013647330321));
#218142=CARTESIAN_POINT('Ctrl Pts',(-63.1927714244286,62.3966764148673,
60.2196342170887));
#218143=CARTESIAN_POINT('Ctrl Pts',(-63.1567815091212,63.5980703290134,
59.7551586861337));
#218144=CARTESIAN_POINT('Ctrl Pts',(-63.1382325648421,64.2316566098064,
59.577812813029));
#218145=CARTESIAN_POINT('Ctrl Pts',(-63.0876061050843,65.9835571276424,
59.2645618345226));
#218146=CARTESIAN_POINT('Ctrl Pts',(-63.0568645631276,67.1143060400938,
59.2499479601664));
#218147=CARTESIAN_POINT('Ctrl Pts',(-63.005891965054,68.8928844070064,59.5207399612207));
#218148=CARTESIAN_POINT('Ctrl Pts',(-62.9865902405449,69.5492990432607,
59.6882858783912));
#218149=CARTESIAN_POINT('Ctrl Pts',(-62.9488489080176,70.8186997677901,
60.1498250157125));
#218150=CARTESIAN_POINT('Ctrl Pts',(-62.9301167844335,71.4286371594735,
60.4425142523593));
#218151=CARTESIAN_POINT('Ctrl Pts',(-62.8963763793845,72.4470147332593,
61.0614295219787));
#218152=CARTESIAN_POINT('Ctrl Pts',(-62.8816004439642,72.8677289241764,
61.3628567478541));
#218153=CARTESIAN_POINT('Ctrl Pts',(-62.8576637723445,73.5180351319628,
61.9075921696466));
#218154=CARTESIAN_POINT('Ctrl Pts',(-62.8484332830644,73.7616829155249,
62.132664553432));
#218155=CARTESIAN_POINT('Ctrl Pts',(-62.8014970604723,74.9411857777908,
63.3333367980829));
#218156=CARTESIAN_POINT('Ctrl Pts',(-62.7630176062056,75.6883752126844,
64.4754208690331));
#218157=CARTESIAN_POINT('Ctrl Pts',(-62.6903484747373,76.6602419101073,
66.8932985386122));
#218158=CARTESIAN_POINT('Ctrl Pts',(-62.6545794831604,76.9104611156789,
68.1331288680544));
#218159=CARTESIAN_POINT('Ctrl Pts',(-62.6006820311669,76.9415153841524,
70.0621434233975));
#218160=CARTESIAN_POINT('Ctrl Pts',(-62.5819408139266,76.8856908376953,
70.7364519076855));
#218161=CARTESIAN_POINT('Ctrl Pts',(-62.5436946277216,76.642179247713,72.0648786987987));
#218162=CARTESIAN_POINT('Ctrl Pts',(-62.5243815110003,76.4549659444319,
72.7157337662098));
#218163=CARTESIAN_POINT('Ctrl Pts',(-62.5042594192214,76.1887426466089,
73.3844628512366));
#218164=CARTESIAN_POINT('Ctrl Pts',(-62.5030257008656,76.1721423876946,
73.4253892597614));
#218165=CARTESIAN_POINT('Ctrl Pts',(-62.5017927901887,76.1552807340937,
73.4662010514616));
#218166=CARTESIAN_POINT('',(-56.402655786563,57.5592983598715,74.2253115652726));
#218167=CARTESIAN_POINT('Ctrl Pts',(-56.5793858481529,60.8283504752015,
78.0464295027996));
#218168=CARTESIAN_POINT('Ctrl Pts',(-56.5407590229759,59.6918928073868,
77.2632582583922));
#218169=CARTESIAN_POINT('Ctrl Pts',(-56.4635053726229,57.7381457991904,
75.2350099031933));
#218170=CARTESIAN_POINT('Ctrl Pts',(-56.3476248970939,56.2287169260511,
71.289035799845));
#218171=CARTESIAN_POINT('Ctrl Pts',(-56.2317444215639,56.3809813114179,
67.0670781799153));
#218172=CARTESIAN_POINT('Ctrl Pts',(-56.1158639460339,58.1705823100065,
63.2401216789652));
#218173=CARTESIAN_POINT('Ctrl Pts',(-55.9999834705049,61.313099618598,60.4164989490926));
#218174=CARTESIAN_POINT('Ctrl Pts',(-55.8841029949749,65.30901125743,59.0450242272283));
#218175=CARTESIAN_POINT('Ctrl Pts',(-55.7682225194459,69.5231601025766,
59.3436988676508));
#218176=CARTESIAN_POINT('Ctrl Pts',(-55.6523420439159,73.2856959312731,
61.2650472476525));
#218177=CARTESIAN_POINT('Ctrl Pts',(-55.5364615683869,75.9985545373602,
64.5036664147486));
#218178=CARTESIAN_POINT('Ctrl Pts',(-55.4205810928579,77.2305202478881,
68.5447697661598));
#218179=CARTESIAN_POINT('Ctrl Pts',(-55.3047006173279,76.7857690673864,
72.746013893864));
#218180=CARTESIAN_POINT('Ctrl Pts',(-55.1888201417989,74.7349952969698,
76.4396006022122));
#218181=CARTESIAN_POINT('Ctrl Pts',(-55.0729396662689,71.4041745240506,
79.0384251072975));
#218182=CARTESIAN_POINT('Ctrl Pts',(-54.9570591907399,67.3227489862028,
80.1293977965976));
#218183=CARTESIAN_POINT('Ctrl Pts',(-54.8411787152099,63.1394714137716,
79.5391058504835));
#218184=CARTESIAN_POINT('Ctrl Pts',(-54.7252982396809,59.5192841709575,
77.3613776404707));
#218185=CARTESIAN_POINT('Ctrl Pts',(-54.6094177641509,57.0376250150175,
73.9423684764854));
#218186=CARTESIAN_POINT('Ctrl Pts',(-54.4935372886209,56.0889598348911,
69.8255383602719));
#218187=CARTESIAN_POINT('Ctrl Pts',(-54.3776568130909,56.8240813181107,
65.6652676678047));
#218188=CARTESIAN_POINT('Ctrl Pts',(-54.2617763375609,59.1261400783554,
62.1228417625685));
#218189=CARTESIAN_POINT('Ctrl Pts',(-54.1458958620309,62.6292181558182,
59.7613380439862));
#218190=CARTESIAN_POINT('Ctrl Pts',(-54.0300153865009,66.776492586088,58.9561233957071));
#218191=CARTESIAN_POINT('Ctrl Pts',(-53.9141349109709,70.9087437938121,
59.8351886867614));
#218192=CARTESIAN_POINT('Ctrl Pts',(-53.7982544354409,74.3691401822294,
62.258804304951));
#218193=CARTESIAN_POINT('Ctrl Pts',(-53.6823739599209,76.6076431474328,
65.8417305258611));
#218194=CARTESIAN_POINT('Ctrl Pts',(-53.5664934843909,77.2684370811464,
70.014452324264));
#218195=CARTESIAN_POINT('Ctrl Pts',(-53.4506130088609,76.2464871457476,
74.1137052024411));
#218196=CARTESIAN_POINT('Ctrl Pts',(-53.3347325333309,73.7042348226836,
77.487902730087));
#218197=CARTESIAN_POINT('Ctrl Pts',(-53.2188520578009,70.0457774353802,
79.6007078263948));
#218198=CARTESIAN_POINT('Ctrl Pts',(-53.1029715822709,65.8526358756345,
80.1162848716646));
#218199=CARTESIAN_POINT('Ctrl Pts',(-52.9870911067409,61.7913204129621,
78.9526816135228));
#218200=CARTESIAN_POINT('Ctrl Pts',(-52.8712106312109,58.5073872312147,
76.2948556810079));
#218201=CARTESIAN_POINT('Ctrl Pts',(-52.7553301556809,56.522825669145,72.5652751099482));
#218202=CARTESIAN_POINT('Ctrl Pts',(-52.6394496801509,56.15308671803,68.356765998908));
#218203=CARTESIAN_POINT('Ctrl Pts',(-52.5235692046209,57.4569413028341,
64.3382813278711));
#218204=CARTESIAN_POINT('Ctrl Pts',(-52.4076887290909,60.2271384976534,
61.1485692199367));
#218205=CARTESIAN_POINT('Ctrl Pts',(-52.2918082535609,64.0233485753049,
59.2946423400516));
#218206=CARTESIAN_POINT('Ctrl Pts',(-52.1759277780309,68.2421545116176,
59.0711869721972));
#218207=CARTESIAN_POINT('Ctrl Pts',(-52.0600473025109,72.2129666206316,
60.5137219022862));
#218208=CARTESIAN_POINT('Ctrl Pts',(-51.9441668269809,75.3046144514435,
63.3929526189662));
#218209=CARTESIAN_POINT('Ctrl Pts',(-51.8282863514509,77.0256728996043,
67.2512182458574));
#218210=CARTESIAN_POINT('Ctrl Pts',(-51.7124058759209,77.1025754485052,
71.4752378750256));
#218211=CARTESIAN_POINT('Ctrl Pts',(-51.5965254003909,75.5230982469212,
75.3935930910952));
#218212=CARTESIAN_POINT('Ctrl Pts',(-51.4806449248609,72.5383031205348,
78.3834515966281));
#218213=CARTESIAN_POINT('Ctrl Pts',(-51.3647644493309,68.6226306709332,
79.9695679533436));
#218214=CARTESIAN_POINT('Ctrl Pts',(-51.2488839738009,64.3984867631581,
79.8998250253566));
#218215=CARTESIAN_POINT('Ctrl Pts',(-51.1330034982709,60.537309566982,78.1853086243629));
#218216=CARTESIAN_POINT('Ctrl Pts',(-51.0171230227409,57.6528427914971,
75.0985453923105));
#218217=CARTESIAN_POINT('Ctrl Pts',(-50.9012425472109,56.2035795976409,
71.1301840145486));
#218218=CARTESIAN_POINT('Ctrl Pts',(-50.7853620716809,56.4198839710304,
66.9110053921681));
#218219=CARTESIAN_POINT('Ctrl Pts',(-50.6694815961509,58.2673737940418,
63.111658450455));
#218220=CARTESIAN_POINT('Ctrl Pts',(-50.5536011206309,61.4523859689387,
60.336058826028));
#218221=CARTESIAN_POINT('Ctrl Pts',(-50.4377206451009,65.4686548966643,
59.0253949753286));
#218222=CARTESIAN_POINT('Ctrl Pts',(-50.3218401695709,69.6777846525631,
59.3880001752186));
#218223=CARTESIAN_POINT('Ctrl Pts',(-50.2059596940409,73.4107236016189,
61.366237423659));
#218224=CARTESIAN_POINT('Ctrl Pts',(-50.0900792185109,76.0741118301684,
64.6456610117157));
#218225=CARTESIAN_POINT('Ctrl Pts',(-49.9741987429809,77.2445971339387,
68.7049983484055));
#218226=CARTESIAN_POINT('Ctrl Pts',(-49.8583182674509,76.7361280689603,
72.8990079143938));
#218227=CARTESIAN_POINT('Ctrl Pts',(-49.7424377919209,74.6295266708348,
76.5610405859094));
#218228=CARTESIAN_POINT('Ctrl Pts',(-49.6265573163909,71.2596439053081,
79.1090104644245));
#218229=CARTESIAN_POINT('Ctrl Pts',(-49.5106768408609,67.1621256395096,
80.1378991151167));
#218230=CARTESIAN_POINT('Ctrl Pts',(-49.3947963653309,62.9883026295467,
79.4842080039734));
#218231=CARTESIAN_POINT('Ctrl Pts',(-49.2789158898109,59.4015395979127,
77.2516717552151));
#218232=CARTESIAN_POINT('Ctrl Pts',(-49.2016622394509,57.7820069698283,
74.9477549101844));
#218233=CARTESIAN_POINT('Ctrl Pts',(-49.1630354142809,57.2293348468531,
73.6830625549967));
#218234=CARTESIAN_POINT('Ctrl Pts',(-56.3552577378769,61.0726603761865,
77.6919120683442));
#218235=CARTESIAN_POINT('Ctrl Pts',(-56.3166309126999,59.9836344637329,
76.9414276436267));
#218236=CARTESIAN_POINT('Ctrl Pts',(-56.2393772623469,58.1114300002093,
74.9978312579017));
#218237=CARTESIAN_POINT('Ctrl Pts',(-56.1234967868169,56.6649993918269,
71.2165482676822));
#218238=CARTESIAN_POINT('Ctrl Pts',(-56.0076163112879,56.8109087960282,
67.1708003444752));
#218239=CARTESIAN_POINT('Ctrl Pts',(-55.8917358357579,58.5258181284236,
63.5035675795475));
#218240=CARTESIAN_POINT('Ctrl Pts',(-55.7758553602289,61.5371777912702,
60.7977929546753));
#218241=CARTESIAN_POINT('Ctrl Pts',(-55.6599748846989,65.3663140994574,
59.4835587753602));
#218242=CARTESIAN_POINT('Ctrl Pts',(-55.5440944091699,69.4045791587436,
59.7697677843113));
#218243=CARTESIAN_POINT('Ctrl Pts',(-55.4282139336399,73.0100799442327,
61.6109258247082));
#218244=CARTESIAN_POINT('Ctrl Pts',(-55.3123334581109,75.6097133511933,
64.7143763916865));
#218245=CARTESIAN_POINT('Ctrl Pts',(-55.1964529825809,76.7902611357812,
68.58681826895));
#218246=CARTESIAN_POINT('Ctrl Pts',(-55.0805725070519,76.3640723089752,
72.612717208417));
#218247=CARTESIAN_POINT('Ctrl Pts',(-54.9646920315229,74.3988906398205,
76.152146567904));
#218248=CARTESIAN_POINT('Ctrl Pts',(-54.8488115559929,71.2070866385185,
78.6425052571067));
#218249=CARTESIAN_POINT('Ctrl Pts',(-54.7329310804639,67.2960054813953,
79.6879445744451));
#218250=CARTESIAN_POINT('Ctrl Pts',(-54.6170506049339,63.2873232362219,
79.1222893429069));
#218251=CARTESIAN_POINT('Ctrl Pts',(-54.5011701294009,59.8182299061273,
77.035451866986));
#218252=CARTESIAN_POINT('Ctrl Pts',(-54.3852896538709,57.4401464955149,
73.7591401486176));
#218253=CARTESIAN_POINT('Ctrl Pts',(-54.2694091783509,56.5310752712668,
69.8141320760029));
#218254=CARTESIAN_POINT('Ctrl Pts',(-54.1535287028209,57.235515363221,65.8274964843525));
#218255=CARTESIAN_POINT('Ctrl Pts',(-54.0376482272909,59.4414942684621,
62.4329190064619));
#218256=CARTESIAN_POINT('Ctrl Pts',(-53.9217677517609,62.7983661588541,
60.1699761668686));
#218257=CARTESIAN_POINT('Ctrl Pts',(-53.8058872762309,66.7725479066749,
59.398368352605));
#218258=CARTESIAN_POINT('Ctrl Pts',(-53.6900068007009,70.7323334485579,
60.2407445429475));
#218259=CARTESIAN_POINT('Ctrl Pts',(-53.5741263251709,74.0483050338323,
62.5632069494067));
#218260=CARTESIAN_POINT('Ctrl Pts',(-53.4582458496409,76.1933807399002,
65.9965944019083));
#218261=CARTESIAN_POINT('Ctrl Pts',(-53.3423653741109,76.8265954534646,
69.9951614340195));
#218262=CARTESIAN_POINT('Ctrl Pts',(-53.2264848985809,75.84729812247,73.9233258808397));
#218263=CARTESIAN_POINT('Ctrl Pts',(-53.1106044230509,73.4111504909153,
77.1566962433291));
#218264=CARTESIAN_POINT('Ctrl Pts',(-52.9947239475209,69.9053842778755,
79.1813202684909));
#218265=CARTESIAN_POINT('Ctrl Pts',(-52.8788434719909,65.8872497336091,
79.6753789369893));
#218266=CARTESIAN_POINT('Ctrl Pts',(-52.7629629964609,61.9954393276913,
78.5603403958908));
#218267=CARTESIAN_POINT('Ctrl Pts',(-52.6470825209309,58.8485659940342,
76.0134427918172));
#218268=CARTESIAN_POINT('Ctrl Pts',(-52.5312020454009,56.946833067975,72.4395218271453));
#218269=CARTESIAN_POINT('Ctrl Pts',(-52.4153215698809,56.5925257233132,
68.4066611192533));
#218270=CARTESIAN_POINT('Ctrl Pts',(-52.2994410943509,57.8419619928253,
64.5558938980169));
#218271=CARTESIAN_POINT('Ctrl Pts',(-52.1835606188209,60.4965408770102,
61.4993091811534));
#218272=CARTESIAN_POINT('Ctrl Pts',(-52.0676801432909,64.1343104664627,
59.7227587040345));
#218273=CARTESIAN_POINT('Ctrl Pts',(-51.9517996677609,68.1770382462698,
59.5086295791555));
#218274=CARTESIAN_POINT('Ctrl Pts',(-51.8359191922309,71.9821225909486,
60.8909581629449));
#218275=CARTESIAN_POINT('Ctrl Pts',(-51.7200387167009,74.9447358895156,
63.6500198923846));
#218276=CARTESIAN_POINT('Ctrl Pts',(-51.6041582411709,76.5939633970318,
67.3472550501956));
#218277=CARTESIAN_POINT('Ctrl Pts',(-51.4882777656409,76.6676563033805,
71.3949789216125));
#218278=CARTESIAN_POINT('Ctrl Pts',(-51.3723972901109,75.1541009379953,
75.1497957399931));
#218279=CARTESIAN_POINT('Ctrl Pts',(-51.2565168145809,72.2938806868999,
78.0148680425532));
#218280=CARTESIAN_POINT('Ctrl Pts',(-51.1406363390509,68.5416346657267,
79.534785468025));
#218281=CARTESIAN_POINT('Ctrl Pts',(-51.0247558635209,64.4937917026564,
79.4679533651302));
#218282=CARTESIAN_POINT('Ctrl Pts',(-50.9088753880009,60.7937664942429,
77.8249948626797));
#218283=CARTESIAN_POINT('Ctrl Pts',(-50.7929949124709,58.0296872407287,
74.8670622968579));
#218284=CARTESIAN_POINT('Ctrl Pts',(-50.6771144369409,56.6409112073073,
71.0643263985101));
#218285=CARTESIAN_POINT('Ctrl Pts',(-50.5612339614109,56.8481877951267,
67.0212414872383));
#218286=CARTESIAN_POINT('Ctrl Pts',(-50.4453534858809,58.6185698755448,
63.3804659554293));
#218287=CARTESIAN_POINT('Ctrl Pts',(-50.3294730103509,61.6706508180947,
60.7207101200916));
#218288=CARTESIAN_POINT('Ctrl Pts',(-50.2135925348209,65.5192947733674,
59.4647487795595));
#218289=CARTESIAN_POINT('Ctrl Pts',(-50.0977120592909,69.552750222577,59.8122201107395));
#218290=CARTESIAN_POINT('Ctrl Pts',(-49.9818315837609,73.1298893983293,
61.7078926778295));
#218291=CARTESIAN_POINT('Ctrl Pts',(-49.8659511082309,75.6821171477224,
64.8504446324208));
#218292=CARTESIAN_POINT('Ctrl Pts',(-49.7500706327009,76.8037505020027,
68.7403594723971));
#218293=CARTESIAN_POINT('Ctrl Pts',(-49.6341901571709,76.3165031516394,
72.7593257953695));
#218294=CARTESIAN_POINT('Ctrl Pts',(-49.5183096816509,74.2978239040633,
76.2685180728018));
#218295=CARTESIAN_POINT('Ctrl Pts',(-49.4024292061209,71.0685882206619,
78.7101446291031));
#218296=CARTESIAN_POINT('Ctrl Pts',(-49.2865487305909,67.1420859895845,
79.6960910777589));
#218297=CARTESIAN_POINT('Ctrl Pts',(-49.1706682550609,63.1424637066209,
79.0696827398739));
#218298=CARTESIAN_POINT('Ctrl Pts',(-49.0547877795309,59.7053995784171,
76.9303247204408));
#218299=CARTESIAN_POINT('Ctrl Pts',(-48.9775341291809,58.1534605594795,
74.7225652803545));
#218300=CARTESIAN_POINT('Ctrl Pts',(-48.9389073040009,57.6238550316623,
73.5106567464228));
#218301=CARTESIAN_POINT('Ctrl Pts',(-56.1311296275999,61.3169702771804,
77.3373946338935));
#218302=CARTESIAN_POINT('Ctrl Pts',(-56.0925028024239,60.2753761200882,
76.619597028865));
#218303=CARTESIAN_POINT('Ctrl Pts',(-56.0152491520709,58.4847142012186,
74.7606526126071));
#218304=CARTESIAN_POINT('Ctrl Pts',(-55.8993686765409,57.1012818576024,
71.1440607355204));
#218305=CARTESIAN_POINT('Ctrl Pts',(-55.7834882010119,57.2408362806385,
67.2745225090351));
#218306=CARTESIAN_POINT('Ctrl Pts',(-55.6676077254819,58.8810539468492,
63.7670134801353));
#218307=CARTESIAN_POINT('Ctrl Pts',(-55.5517272499529,61.7612559639331,
61.1790869602541));
#218308=CARTESIAN_POINT('Ctrl Pts',(-55.4358467744229,65.4236169414932,
59.9220933234976));
#218309=CARTESIAN_POINT('Ctrl Pts',(-55.3199662988939,69.2859982149144,
60.1958367009625));
#218310=CARTESIAN_POINT('Ctrl Pts',(-55.2040858233639,72.7344639571905,
61.9568044017577));
#218311=CARTESIAN_POINT('Ctrl Pts',(-55.0882053478349,75.2208721650242,
64.9250863686192));
#218312=CARTESIAN_POINT('Ctrl Pts',(-54.9723248723049,76.3500020236737,
68.6288667717324));
#218313=CARTESIAN_POINT('Ctrl Pts',(-54.8564443967759,75.9423755505674,
72.4794205229619));
#218314=CARTESIAN_POINT('Ctrl Pts',(-54.7405639212469,74.0627859826778,
75.8646925335889));
#218315=CARTESIAN_POINT('Ctrl Pts',(-54.6246834457169,71.0099987529967,
78.2465854069094));
#218316=CARTESIAN_POINT('Ctrl Pts',(-54.5088029701909,67.2692619766016,
79.2464913522907));
#218317=CARTESIAN_POINT('Ctrl Pts',(-54.3929224946609,63.4351750586927,
78.7054728353225));
#218318=CARTESIAN_POINT('Ctrl Pts',(-54.2770420191309,60.1171756413221,
76.7095260935192));
#218319=CARTESIAN_POINT('Ctrl Pts',(-54.1611615436009,57.8426679760259,
73.5759118207695));
#218320=CARTESIAN_POINT('Ctrl Pts',(-54.0452810680709,56.973190707635,69.8027257917525));
#218321=CARTESIAN_POINT('Ctrl Pts',(-53.9294005925409,57.6469494083309,
65.9897253009273));
#218322=CARTESIAN_POINT('Ctrl Pts',(-53.8135201170109,59.7568484585497,
62.7429962503755));
#218323=CARTESIAN_POINT('Ctrl Pts',(-53.6976396414809,62.9675141618542,
60.5786142897589));
#218324=CARTESIAN_POINT('Ctrl Pts',(-53.5817591659509,66.7686032272295,
59.8406133095026));
#218325=CARTESIAN_POINT('Ctrl Pts',(-53.4658786904209,70.5559231032727,
60.6463003991197));
#218326=CARTESIAN_POINT('Ctrl Pts',(-53.3499982148909,73.7274698854091,
62.8676095938364));
#218327=CARTESIAN_POINT('Ctrl Pts',(-53.2341177393609,75.7791183323543,
66.1514582779196));
#218328=CARTESIAN_POINT('Ctrl Pts',(-53.1182372638309,76.3847538257845,
69.9758705437336));
#218329=CARTESIAN_POINT('Ctrl Pts',(-53.0023567883009,75.4481090992107,
73.7329465591993));
#218330=CARTESIAN_POINT('Ctrl Pts',(-52.8864763127809,73.1180661591807,
76.8254897565408));
#218331=CARTESIAN_POINT('Ctrl Pts',(-52.7705958372509,69.7649911204159,
78.7619327105721));
#218332=CARTESIAN_POINT('Ctrl Pts',(-52.6547153617209,65.9218635916335,
79.2344730023141));
#218333=CARTESIAN_POINT('Ctrl Pts',(-52.5388348861909,62.1995582424626,
78.1679991782881));
#218334=CARTESIAN_POINT('Ctrl Pts',(-52.4229544106609,59.1897447568815,
75.7320299026639));
#218335=CARTESIAN_POINT('Ctrl Pts',(-52.3070739351309,57.3708404668259,
72.3137685443966));
#218336=CARTESIAN_POINT('Ctrl Pts',(-52.1911934596009,57.0319647285943,
68.4565562396562));
#218337=CARTESIAN_POINT('Ctrl Pts',(-52.0753129840709,58.2269826827762,
64.7735064682079));
#218338=CARTESIAN_POINT('Ctrl Pts',(-51.9594325085409,60.7659432563194,
61.8500491424068));
#218339=CARTESIAN_POINT('Ctrl Pts',(-51.8435520330109,64.2452723575601,
60.1508750680324));
#218340=CARTESIAN_POINT('Ctrl Pts',(-51.7276715574809,68.1119219808598,
59.9460721861075));
#218341=CARTESIAN_POINT('Ctrl Pts',(-51.6117910819509,71.7512785612103,
61.2681944235776));
#218342=CARTESIAN_POINT('Ctrl Pts',(-51.4959106064209,74.5848573275517,
63.9070871657535));
#218343=CARTESIAN_POINT('Ctrl Pts',(-51.3800301308909,76.162253894446,67.4432918544721));
#218344=CARTESIAN_POINT('Ctrl Pts',(-51.2641496553709,76.2327371582677,
71.3147199681373));
#218345=CARTESIAN_POINT('Ctrl Pts',(-51.1482691798409,74.7851036291041,
74.9059983888393));
#218346=CARTESIAN_POINT('Ctrl Pts',(-51.0323887043109,72.0494582533171,
77.6462844884435));
#218347=CARTESIAN_POINT('Ctrl Pts',(-50.9165082287809,68.4606386605805,
79.1000029826967));
#218348=CARTESIAN_POINT('Ctrl Pts',(-50.8006277532509,64.5890966422126,
79.0360817049179));
#218349=CARTESIAN_POINT('Ctrl Pts',(-50.6847472777209,61.0502234215632,
77.4646811010362));
#218350=CARTESIAN_POINT('Ctrl Pts',(-50.5688668021909,58.4065316900025,
74.6355792014605));
#218351=CARTESIAN_POINT('Ctrl Pts',(-50.4529863266609,57.0782428169735,
70.9984687825245));
#218352=CARTESIAN_POINT('Ctrl Pts',(-50.3371058511309,57.2764916192201,
67.1314775823678));
#218353=CARTESIAN_POINT('Ctrl Pts',(-50.2212253756009,58.9697659570288,
63.6492734604498));
#218354=CARTESIAN_POINT('Ctrl Pts',(-50.1053449000709,61.8889156671989,
61.105361414176));
#218355=CARTESIAN_POINT('Ctrl Pts',(-49.9894644245409,65.5699346500343,
59.9041025837992));
#218356=CARTESIAN_POINT('Ctrl Pts',(-49.8735839490209,69.4277157925497,
60.2364400462553));
#218357=CARTESIAN_POINT('Ctrl Pts',(-49.7577034734909,72.8490551950089,
62.0495479319754));
#218358=CARTESIAN_POINT('Ctrl Pts',(-49.6418229979609,75.2901224652598,
65.055228253093));
#218359=CARTESIAN_POINT('Ctrl Pts',(-49.5259425224309,76.3629038700644,
68.7757205963566));
#218360=CARTESIAN_POINT('Ctrl Pts',(-49.4100620469009,75.8968782343272,
72.6196436763185));
#218361=CARTESIAN_POINT('Ctrl Pts',(-49.2941815713709,73.9661211373074,
75.9759955596767));
#218362=CARTESIAN_POINT('Ctrl Pts',(-49.1783010958409,70.8775325360307,
78.3112787937738));
#218363=CARTESIAN_POINT('Ctrl Pts',(-49.0624206203109,67.1220463396723,
79.254283040401));
#218364=CARTESIAN_POINT('Ctrl Pts',(-48.9465401447809,63.2966247837026,
78.6551574757722));
#218365=CARTESIAN_POINT('Ctrl Pts',(-48.8306596692509,60.0092595589126,
76.6089776856617));
#218366=CARTESIAN_POINT('Ctrl Pts',(-48.7534060189009,58.5249141491315,
74.4973756505227));
#218367=CARTESIAN_POINT('Ctrl Pts',(-48.7147791937209,58.0183752164734,
73.3382509378444));
#218368=CARTESIAN_POINT('Ctrl Pts',(-55.9070015173239,61.5612801781646,
76.9828771994399));
#218369=CARTESIAN_POINT('Ctrl Pts',(-55.8683746921479,60.5671177764436,
76.2977664141033));
#218370=CARTESIAN_POINT('Ctrl Pts',(-55.7911210417949,58.8579984022376,
74.5234739673154));
#218371=CARTESIAN_POINT('Ctrl Pts',(-55.6752405662649,57.5375643233782,
71.0715732033576));
#218372=CARTESIAN_POINT('Ctrl Pts',(-55.5593600907359,57.67076376524,67.3782446735902));
#218373=CARTESIAN_POINT('Ctrl Pts',(-55.4434796152059,59.2362897652659,
64.0304593807185));
#218374=CARTESIAN_POINT('Ctrl Pts',(-55.3275991396769,61.9853341366056,
61.5603809658357));
#218375=CARTESIAN_POINT('Ctrl Pts',(-55.2117186641469,65.4809197835205,
60.3606278716295));
#218376=CARTESIAN_POINT('Ctrl Pts',(-55.0958381886179,69.1674172710837,
60.6219056176175));
#218377=CARTESIAN_POINT('Ctrl Pts',(-54.9799577130879,72.4588479701517,
62.3026829788097));
#218378=CARTESIAN_POINT('Ctrl Pts',(-54.8640772375589,74.8320309788573,
65.135796345557));
#218379=CARTESIAN_POINT('Ctrl Pts',(-54.7481967620289,75.9097429115672,
68.6709152745216));
#218380=CARTESIAN_POINT('Ctrl Pts',(-54.6323162864999,75.5206787921568,
72.3461238375152));
#218381=CARTESIAN_POINT('Ctrl Pts',(-54.5164358109709,73.7266813255289,
75.5772384992809));
#218382=CARTESIAN_POINT('Ctrl Pts',(-54.4005553354409,70.8129108674647,
77.8506655567186));
#218383=CARTESIAN_POINT('Ctrl Pts',(-54.2846748599109,67.2425184717931,
78.8050381301378));
#218384=CARTESIAN_POINT('Ctrl Pts',(-54.1687943843809,63.5830268811459,
78.2886563277363));
#218385=CARTESIAN_POINT('Ctrl Pts',(-54.0529139088509,60.4161213764918,
76.3836003200345));
#218386=CARTESIAN_POINT('Ctrl Pts',(-53.9370334333209,58.2451894565326,
73.3926834929056));
#218387=CARTESIAN_POINT('Ctrl Pts',(-53.8211529577909,57.4153061440108,
69.7913195074836));
#218388=CARTESIAN_POINT('Ctrl Pts',(-53.7052724822609,58.0583834534414,
66.1519541174747));
#218389=CARTESIAN_POINT('Ctrl Pts',(-53.5893920067309,60.0722026486568,
63.0530734942681));
#218390=CARTESIAN_POINT('Ctrl Pts',(-53.4735115312009,63.1366621648809,
60.9872524126374));
#218391=CARTESIAN_POINT('Ctrl Pts',(-53.3576310556809,66.7646585478257,
60.2828582664043));
#218392=CARTESIAN_POINT('Ctrl Pts',(-53.2417505801509,70.3795127580189,
61.0518562553049));
#218393=CARTESIAN_POINT('Ctrl Pts',(-53.1258701046209,73.4066347370121,
63.172012238292));
#218394=CARTESIAN_POINT('Ctrl Pts',(-53.0099896290909,75.3648559248227,
66.3063221539671));
#218395=CARTESIAN_POINT('Ctrl Pts',(-52.8941091535609,75.9429121981029,
69.9565796534893));
#218396=CARTESIAN_POINT('Ctrl Pts',(-52.7782286780309,75.0489200759327,
73.5425672375986));
#218397=CARTESIAN_POINT('Ctrl Pts',(-52.6623482025009,72.8249818274116,
76.4942832697837));
#218398=CARTESIAN_POINT('Ctrl Pts',(-52.5464677269709,69.6245979629103,
78.3425451526678));
#218399=CARTESIAN_POINT('Ctrl Pts',(-52.4305872514409,65.9564774496083,
78.7935670676356));
#218400=CARTESIAN_POINT('Ctrl Pts',(-52.3147067759109,62.4036771571881,
77.77565796066));
#218401=CARTESIAN_POINT('Ctrl Pts',(-52.1988263003809,59.5309235196917,
75.4506170134694));
#218402=CARTESIAN_POINT('Ctrl Pts',(-52.0829458248509,57.7948478656563,
72.1880152615929));
#218403=CARTESIAN_POINT('Ctrl Pts',(-51.9670653493209,57.4714037338775,
68.5064513600016));
#218404=CARTESIAN_POINT('Ctrl Pts',(-51.8511848737909,58.6120033727586,
64.991119038349));
#218405=CARTESIAN_POINT('Ctrl Pts',(-51.7353043982609,61.0353456356765,
62.2007891036227));
#218406=CARTESIAN_POINT('Ctrl Pts',(-51.6194239227409,64.356234248718,60.5789914320152));
#218407=CARTESIAN_POINT('Ctrl Pts',(-51.5035434472109,68.0468057155105,
60.3835147930695));
#218408=CARTESIAN_POINT('Ctrl Pts',(-51.3876629716809,71.520434531528,61.6454306842399));
#218409=CARTESIAN_POINT('Ctrl Pts',(-51.2717824961509,74.2249787656239,
64.164154439174));
#218410=CARTESIAN_POINT('Ctrl Pts',(-51.1559020206209,75.7305443918741,
67.5393286588116));
#218411=CARTESIAN_POINT('Ctrl Pts',(-51.0400215450909,75.7978180131431,
71.2344610147253));
#218412=CARTESIAN_POINT('Ctrl Pts',(-50.9241410695609,74.4161063201778,
74.6622010377381));
#218413=CARTESIAN_POINT('Ctrl Pts',(-50.8082605940309,71.8050358196814,
77.2777009343682));
#218414=CARTESIAN_POINT('Ctrl Pts',(-50.6923801185009,68.3796426553727,
78.6652204973787));
#218415=CARTESIAN_POINT('Ctrl Pts',(-50.5764996429709,64.6844015817095,
78.604210044692));
#218416=CARTESIAN_POINT('Ctrl Pts',(-50.4606191674409,61.3066803488238,
77.1043673393539));
#218417=CARTESIAN_POINT('Ctrl Pts',(-50.3447386919109,58.7833761392345,
74.4040961060069));
#218418=CARTESIAN_POINT('Ctrl Pts',(-50.2288582163809,57.515574426631,70.9326111664812));
#218419=CARTESIAN_POINT('Ctrl Pts',(-50.1129777408609,57.7047954433261,
67.2417136774408));
#218420=CARTESIAN_POINT('Ctrl Pts',(-49.9970972653309,59.3209620385326,
63.9180809654223));
#218421=CARTESIAN_POINT('Ctrl Pts',(-49.8812167898009,62.107180516346,61.4900127082349));
#218422=CARTESIAN_POINT('Ctrl Pts',(-49.7653363142709,65.6205745267381,
60.3434563880283));
#218423=CARTESIAN_POINT('Ctrl Pts',(-49.6494558387409,69.3026813625722,
60.6606599817841));
#218424=CARTESIAN_POINT('Ctrl Pts',(-49.5335753632109,72.5682209917208,
62.3912031861476));
#218425=CARTESIAN_POINT('Ctrl Pts',(-49.4176948876809,74.8981277828147,
65.2600118737985));
#218426=CARTESIAN_POINT('Ctrl Pts',(-49.3018144121509,75.9220572381282,
68.8110817203493));
#218427=CARTESIAN_POINT('Ctrl Pts',(-49.1859339366209,75.4772533170059,
72.4799615572945));
#218428=CARTESIAN_POINT('Ctrl Pts',(-49.0700534610909,73.634418370535,75.6834730465697));
#218429=CARTESIAN_POINT('Ctrl Pts',(-48.9541729855609,70.6864768513839,
77.9124129584511));
#218430=CARTESIAN_POINT('Ctrl Pts',(-48.8382925100409,67.1020066897472,
78.8124750030432));
#218431=CARTESIAN_POINT('Ctrl Pts',(-48.7224120345109,63.4507858607777,
78.2406322116709));
#218432=CARTESIAN_POINT('Ctrl Pts',(-48.6065315589809,60.313119539417,76.2876306508875));
#218433=CARTESIAN_POINT('Ctrl Pts',(-48.5292779086209,58.896367738792,74.2721860206966));
#218434=CARTESIAN_POINT('Ctrl Pts',(-48.4906510834509,58.4128954012822,
73.1658451292715));
#218435=CARTESIAN_POINT('Ctrl Pts',(-49.2716875596105,60.362314694705,77.6221314644388));
#218436=CARTESIAN_POINT('Ctrl Pts',(-49.1710276021328,60.4814587922915,
77.4698472472393));
#218437=CARTESIAN_POINT('Ctrl Pts',(-49.0703675292835,60.6006070147117,
77.3175659697655));
#218438=CARTESIAN_POINT('Ctrl Pts',(-48.8698648784283,60.8379437239874,
77.01424632034));
#218439=CARTESIAN_POINT('Ctrl Pts',(-48.7700220760568,60.9561324122244,
76.8632075588121));
#218440=CARTESIAN_POINT('Ctrl Pts',(-48.6701794005812,61.0743248382571,
76.7121720277662));
#218441=CARTESIAN_POINT('Ctrl Pts',(-49.3172045433909,60.6595417501922,
77.9029428178256));
#218442=CARTESIAN_POINT('Ctrl Pts',(-49.2671675200609,59.1615528419803,
76.9294625104546));
#218443=CARTESIAN_POINT('Ctrl Pts',(-49.1670934734009,56.6466762806369,
74.1587488145408));
#218444=CARTESIAN_POINT('Ctrl Pts',(-49.0169824034109,55.4130069209437,
68.5383989146951));
#218445=CARTESIAN_POINT('Ctrl Pts',(-48.8668713334209,57.1841073201011,
62.9167841918779));
#218446=CARTESIAN_POINT('Ctrl Pts',(-48.7667972867609,60.1408900588271,
60.1918250007294));
#218447=CARTESIAN_POINT('Ctrl Pts',(-48.7167602634309,61.8842256853186,
59.2817848695541));
#218448=CARTESIAN_POINT('Ctrl Pts',(-49.0930764331109,60.9113854019325,
77.5537369843529));
#218449=CARTESIAN_POINT('Ctrl Pts',(-49.0430394097809,59.4739188100978,
76.6239047484312));
#218450=CARTESIAN_POINT('Ctrl Pts',(-48.9429653631309,57.0567877266815,
73.9726075199027));
#218451=CARTESIAN_POINT('Ctrl Pts',(-48.7928542931309,55.8614156728147,
68.5806263247324));
#218452=CARTESIAN_POINT('Ctrl Pts',(-48.6427432231409,57.5522584141988,
63.176215785295));
#218453=CARTESIAN_POINT('Ctrl Pts',(-48.5426691764809,60.390720514573,60.5503257501769));
#218454=CARTESIAN_POINT('Ctrl Pts',(-48.4926321531609,62.0664492882006,
59.6718675500255));
#218455=CARTESIAN_POINT('Ctrl Pts',(-48.8689483228409,61.1632290536717,
77.204531150883));
#218456=CARTESIAN_POINT('Ctrl Pts',(-48.8189112995109,59.7862847782248,
76.3183469864108));
#218457=CARTESIAN_POINT('Ctrl Pts',(-48.7188372528509,57.4668991727264,
73.7864662252636));
#218458=CARTESIAN_POINT('Ctrl Pts',(-48.5687261828609,56.3098244246853,
68.6228537347707));
#218459=CARTESIAN_POINT('Ctrl Pts',(-48.4186151128609,57.9204095082861,
63.4356473787112));
#218460=CARTESIAN_POINT('Ctrl Pts',(-48.3185410662109,60.6405509703189,
60.9088264996243));
#218461=CARTESIAN_POINT('Ctrl Pts',(-48.2685040428809,62.2486728910826,
60.0619502304968));
#218462=CARTESIAN_POINT('Ctrl Pts',(-48.6448202125609,61.4150727054204,
76.8553253174161));
#218463=CARTESIAN_POINT('Ctrl Pts',(-48.5947831892309,60.0986507463515,
76.0127892243912));
#218464=CARTESIAN_POINT('Ctrl Pts',(-48.4947091425709,57.8770106187709,
73.6003249306255));
#218465=CARTESIAN_POINT('Ctrl Pts',(-48.3445980725809,56.7582331765563,
68.665081144808));
#218466=CARTESIAN_POINT('Ctrl Pts',(-48.1944870025909,58.2885606023838,
63.6950789721284));
#218467=CARTESIAN_POINT('Ctrl Pts',(-48.0944129559309,60.8903814260647,
61.2673272490718));
#218468=CARTESIAN_POINT('Ctrl Pts',(-48.0443759326009,62.4308964939646,
60.4520329109682));
#218469=CARTESIAN_POINT('Ctrl Pts',(-48.173560826516,61.9759278335774,60.4464459620599));
#218470=CARTESIAN_POINT('Ctrl Pts',(-48.1596729098122,61.9881764360414,
60.4701459438214));
#218471=CARTESIAN_POINT('Ctrl Pts',(-48.1457849931352,62.0004250385118,
60.4938459255953));
#218472=CARTESIAN_POINT('Ctrl Pts',(-48.1179938256783,62.0249357675969,
60.5412720571877));
#218473=CARTESIAN_POINT('Ctrl Pts',(-48.1040905748985,62.0371978942117,
60.5649982070061));
#218474=CARTESIAN_POINT('Ctrl Pts',(-48.0901873241468,62.0494600208332,
60.5887243568377));
#218475=CARTESIAN_POINT('Origin',(-47.9901862140809,61.5168009229541,59.5580752732411));
#218476=CARTESIAN_POINT('Ctrl Pts',(-47.890187490573,62.0494598736152,60.5887240719837));
#218477=CARTESIAN_POINT('Ctrl Pts',(-47.8762912240803,62.0372039110344,
60.5650098490355));
#218478=CARTESIAN_POINT('Ctrl Pts',(-47.8623949575891,62.0249479484533,
60.5412956260867));
#218479=CARTESIAN_POINT('Ctrl Pts',(-47.8346038364013,62.0004372684354,
60.4938695894352));
#218480=CARTESIAN_POINT('Ctrl Pts',(-47.8207089817047,61.9881825509987,
60.4701577757327));
#218481=CARTESIAN_POINT('Ctrl Pts',(-47.8068141270095,61.9759278335617,
60.4464459620295));
#218482=CARTESIAN_POINT('Ctrl Pts',(-48.5133467647509,61.4150727054112,
76.8553253174122));
#218483=CARTESIAN_POINT('Ctrl Pts',(-48.4633097414209,60.0986507463519,
76.0127892243903));
#218484=CARTESIAN_POINT('Ctrl Pts',(-48.3632356947609,57.8770106187713,
73.6003249306246));
#218485=CARTESIAN_POINT('Ctrl Pts',(-48.2131246247709,56.7582331765567,
68.6650811448071));
#218486=CARTESIAN_POINT('Ctrl Pts',(-48.0630135547809,58.2885606023838,
63.6950789721284));
#218487=CARTESIAN_POINT('Ctrl Pts',(-47.9629395081209,60.8903814260647,
61.2673272490718));
#218488=CARTESIAN_POINT('Ctrl Pts',(-47.9129024847909,62.4308964939646,
60.4520329109682));
#218489=CARTESIAN_POINT('Ctrl Pts',(-48.2892186544709,61.163229053672,77.2045311508821));
#218490=CARTESIAN_POINT('Ctrl Pts',(-48.2391816311409,59.7862847782252,
76.3183469864098));
#218491=CARTESIAN_POINT('Ctrl Pts',(-48.1391075844909,57.4668991727267,
73.7864662252627));
#218492=CARTESIAN_POINT('Ctrl Pts',(-47.9889965144909,56.3098244246853,
68.6228537347707));
#218493=CARTESIAN_POINT('Ctrl Pts',(-47.8388854445009,57.9204095082865,
63.4356473787103));
#218494=CARTESIAN_POINT('Ctrl Pts',(-47.7388113978409,60.6405509703189,
60.9088264996243));
#218495=CARTESIAN_POINT('Ctrl Pts',(-47.6887743745209,62.2486728910826,
60.0619502304968));
#218496=CARTESIAN_POINT('Ctrl Pts',(-48.0650905442009,60.9113854019325,
77.5537369843529));
#218497=CARTESIAN_POINT('Ctrl Pts',(-48.0150535208709,59.4739188100982,
76.6239047484303));
#218498=CARTESIAN_POINT('Ctrl Pts',(-47.9149794742109,57.0567877266818,
73.9726075199017));
#218499=CARTESIAN_POINT('Ctrl Pts',(-47.7648684042209,55.8614156728147,
68.5806263247324));
#218500=CARTESIAN_POINT('Ctrl Pts',(-47.6147573342209,57.5522584141988,
63.176215785295));
#218501=CARTESIAN_POINT('Ctrl Pts',(-47.5146832875709,60.390720514573,60.5503257501769));
#218502=CARTESIAN_POINT('Ctrl Pts',(-47.4646462642409,62.0664492882006,
59.6718675500255));
#218503=CARTESIAN_POINT('Ctrl Pts',(-47.8409624339209,60.6595417501829,
77.9029428178218));
#218504=CARTESIAN_POINT('Ctrl Pts',(-47.7909254105909,59.1615528419807,
76.9294625104537));
#218505=CARTESIAN_POINT('Ctrl Pts',(-47.6908513639309,56.6466762806373,
74.1587488145399));
#218506=CARTESIAN_POINT('Ctrl Pts',(-47.5407402939409,55.4130069209437,
68.5383989146951));
#218507=CARTESIAN_POINT('Ctrl Pts',(-47.3906292239509,57.1841073201011,
62.9167841918779));
#218508=CARTESIAN_POINT('Ctrl Pts',(-47.2905551772909,60.1408900588271,
60.1918250007294));
#218509=CARTESIAN_POINT('Ctrl Pts',(-47.2405181539609,61.8842256853186,
59.2817848695541));
#218510=CARTESIAN_POINT('Ctrl Pts',(-48.4651187514177,61.0741848222236,
76.7120624159032));
#218511=CARTESIAN_POINT('Ctrl Pts',(-48.3651833447158,60.9558726340169,
76.8632423199665));
#218512=CARTESIAN_POINT('Ctrl Pts',(-48.2652478157504,60.837564185308,77.0144254557038));
#218513=CARTESIAN_POINT('Ctrl Pts',(-48.0647417952908,60.6002034168244,
77.3177584421339));
#218514=CARTESIAN_POINT('Ctrl Pts',(-47.9641710718521,60.4811508722256,
77.4699086827435));
#218515=CARTESIAN_POINT('Ctrl Pts',(-47.8636004674102,60.3621024374858,
77.6220618559046));
#218516=CARTESIAN_POINT('Ctrl Pts',(-55.7755280695129,61.5612801781646,
76.9828771994399));
#218517=CARTESIAN_POINT('Ctrl Pts',(-55.7369012443359,60.5671177764436,
76.2977664141033));
#218518=CARTESIAN_POINT('Ctrl Pts',(-55.6596475939829,58.8579984022376,
74.5234739673154));
#218519=CARTESIAN_POINT('Ctrl Pts',(-55.5437671184529,57.5375643233782,
71.0715732033576));
#218520=CARTESIAN_POINT('Ctrl Pts',(-55.4278866429239,57.67076376524,67.3782446735902));
#218521=CARTESIAN_POINT('Ctrl Pts',(-55.3120061673939,59.2362897652659,
64.0304593807185));
#218522=CARTESIAN_POINT('Ctrl Pts',(-55.1961256918649,61.9853341366056,
61.5603809658357));
#218523=CARTESIAN_POINT('Ctrl Pts',(-55.0802452163349,65.4809197835205,
60.3606278716295));
#218524=CARTESIAN_POINT('Ctrl Pts',(-54.9643647408059,69.1674172710837,
60.6219056176175));
#218525=CARTESIAN_POINT('Ctrl Pts',(-54.8484842652759,72.4588479701517,
62.3026829788097));
#218526=CARTESIAN_POINT('Ctrl Pts',(-54.7326037897459,74.8320309788573,
65.135796345557));
#218527=CARTESIAN_POINT('Ctrl Pts',(-54.6167233142169,75.9097429115672,
68.6709152745216));
#218528=CARTESIAN_POINT('Ctrl Pts',(-54.5008428386909,75.5206787921569,
72.3461238375153));
#218529=CARTESIAN_POINT('Ctrl Pts',(-54.3849623631609,73.7266813255289,
75.5772384992809));
#218530=CARTESIAN_POINT('Ctrl Pts',(-54.2690818876309,70.8129108674647,
77.8506655567186));
#218531=CARTESIAN_POINT('Ctrl Pts',(-54.1532014121009,67.2425184717931,
78.8050381301378));
#218532=CARTESIAN_POINT('Ctrl Pts',(-54.0373209365709,63.5830268811459,
78.2886563277363));
#218533=CARTESIAN_POINT('Ctrl Pts',(-53.9214404610409,60.4161213764918,
76.3836003200345));
#218534=CARTESIAN_POINT('Ctrl Pts',(-53.8055599855109,58.2451894565326,
73.3926834929056));
#218535=CARTESIAN_POINT('Ctrl Pts',(-53.6896795099809,57.4153061440108,
69.7913195074836));
#218536=CARTESIAN_POINT('Ctrl Pts',(-53.5737990344509,58.0583834534414,
66.1519541174747));
#218537=CARTESIAN_POINT('Ctrl Pts',(-53.4579185589209,60.0722026486568,
63.0530734942681));
#218538=CARTESIAN_POINT('Ctrl Pts',(-53.3420380833909,63.1366621648809,
60.9872524126374));
#218539=CARTESIAN_POINT('Ctrl Pts',(-53.2261576078609,66.7646585478257,
60.2828582664043));
#218540=CARTESIAN_POINT('Ctrl Pts',(-53.1102771323309,70.3795127580189,
61.0518562553049));
#218541=CARTESIAN_POINT('Ctrl Pts',(-52.9943966568009,73.4066347370121,
63.172012238292));
#218542=CARTESIAN_POINT('Ctrl Pts',(-52.8785161812709,75.3648559248227,
66.3063221539671));
#218543=CARTESIAN_POINT('Ctrl Pts',(-52.7626357057409,75.9429121981029,
69.9565796534893));
#218544=CARTESIAN_POINT('Ctrl Pts',(-52.6467552302109,75.0489200759327,
73.5425672375986));
#218545=CARTESIAN_POINT('Ctrl Pts',(-52.5308747546809,72.8249818274117,
76.4942832697837));
#218546=CARTESIAN_POINT('Ctrl Pts',(-52.4149942791509,69.6245979629103,
78.3425451526678));
#218547=CARTESIAN_POINT('Ctrl Pts',(-52.2991138036209,65.9564774496083,
78.7935670676356));
#218548=CARTESIAN_POINT('Ctrl Pts',(-52.1832333281009,62.4036771571881,
77.77565796066));
#218549=CARTESIAN_POINT('Ctrl Pts',(-52.0673528525709,59.5309235196917,
75.4506170134694));
#218550=CARTESIAN_POINT('Ctrl Pts',(-51.9514723770409,57.7948478656563,
72.1880152615929));
#218551=CARTESIAN_POINT('Ctrl Pts',(-51.8355919015109,57.4714037338775,
68.5064513600016));
#218552=CARTESIAN_POINT('Ctrl Pts',(-51.7197114259809,58.6120033727586,
64.991119038349));
#218553=CARTESIAN_POINT('Ctrl Pts',(-51.6038309504509,61.0353456356765,
62.2007891036227));
#218554=CARTESIAN_POINT('Ctrl Pts',(-51.4879504749209,64.356234248718,60.5789914320152));
#218555=CARTESIAN_POINT('Ctrl Pts',(-51.3720699993909,68.0468057155105,
60.3835147930695));
#218556=CARTESIAN_POINT('Ctrl Pts',(-51.2561895238609,71.520434531528,61.6454306842399));
#218557=CARTESIAN_POINT('Ctrl Pts',(-51.1403090483309,74.2249787656239,
64.164154439174));
#218558=CARTESIAN_POINT('Ctrl Pts',(-51.0244285728009,75.7305443918741,
67.5393286588116));
#218559=CARTESIAN_POINT('Ctrl Pts',(-50.9085480972709,75.7978180131431,
71.2344610147254));
#218560=CARTESIAN_POINT('Ctrl Pts',(-50.7926676217409,74.4161063201778,
74.6622010377381));
#218561=CARTESIAN_POINT('Ctrl Pts',(-50.6767871462109,71.8050358196814,
77.2777009343682));
#218562=CARTESIAN_POINT('Ctrl Pts',(-50.5609066706809,68.3796426553727,
78.6652204973787));
#218563=CARTESIAN_POINT('Ctrl Pts',(-50.4450261951609,64.6844015817095,
78.604210044692));
#218564=CARTESIAN_POINT('Ctrl Pts',(-50.3291457196309,61.3066803488238,
77.1043673393539));
#218565=CARTESIAN_POINT('Ctrl Pts',(-50.2132652441009,58.7833761392345,
74.4040961060069));
#218566=CARTESIAN_POINT('Ctrl Pts',(-50.0973847685709,57.515574426631,70.9326111664812));
#218567=CARTESIAN_POINT('Ctrl Pts',(-49.9815042930409,57.7047954433261,
67.2417136774408));
#218568=CARTESIAN_POINT('Ctrl Pts',(-49.8656238175109,59.3209620385326,
63.9180809654223));
#218569=CARTESIAN_POINT('Ctrl Pts',(-49.7497433419809,62.107180516346,61.4900127082349));
#218570=CARTESIAN_POINT('Ctrl Pts',(-49.6338628664509,65.6205745267381,
60.3434563880283));
#218571=CARTESIAN_POINT('Ctrl Pts',(-49.5179823909209,69.3026813625722,
60.6606599817841));
#218572=CARTESIAN_POINT('Ctrl Pts',(-49.4021019153909,72.5682209917208,
62.3912031861476));
#218573=CARTESIAN_POINT('Ctrl Pts',(-49.2862214398709,74.8981277828147,
65.2600118737985));
#218574=CARTESIAN_POINT('Ctrl Pts',(-49.1703409643409,75.9220572381282,
68.8110817203493));
#218575=CARTESIAN_POINT('Ctrl Pts',(-49.0544604888109,75.4772533170059,
72.4799615572945));
#218576=CARTESIAN_POINT('Ctrl Pts',(-48.9385800132809,73.634418370535,75.6834730465697));
#218577=CARTESIAN_POINT('Ctrl Pts',(-48.8226995377509,70.6864768513839,
77.9124129584511));
#218578=CARTESIAN_POINT('Ctrl Pts',(-48.7068190622209,67.1020066897472,
78.8124750030432));
#218579=CARTESIAN_POINT('Ctrl Pts',(-48.5909385866909,63.4507858607777,
78.2406322116709));
#218580=CARTESIAN_POINT('Ctrl Pts',(-48.4750581111709,60.313119539417,76.2876306508875));
#218581=CARTESIAN_POINT('Ctrl Pts',(-48.3978044608109,58.896367738792,74.2721860206966));
#218582=CARTESIAN_POINT('Ctrl Pts',(-48.3591776356409,58.4128954012822,
73.1658451292715));
#218583=CARTESIAN_POINT('Ctrl Pts',(-55.5513999592359,61.3169702771804,
77.3373946338935));
#218584=CARTESIAN_POINT('Ctrl Pts',(-55.5127731340599,60.2753761200882,
76.619597028865));
#218585=CARTESIAN_POINT('Ctrl Pts',(-55.4355194837069,58.4847142012186,
74.7606526126071));
#218586=CARTESIAN_POINT('Ctrl Pts',(-55.3196390081769,57.1012818576024,
71.1440607355204));
#218587=CARTESIAN_POINT('Ctrl Pts',(-55.2037585326479,57.2408362806385,
67.2745225090351));
#218588=CARTESIAN_POINT('Ctrl Pts',(-55.0878780571179,58.8810539468492,
63.7670134801353));
#218589=CARTESIAN_POINT('Ctrl Pts',(-54.9719975815889,61.7612559639331,
61.1790869602541));
#218590=CARTESIAN_POINT('Ctrl Pts',(-54.8561171060589,65.4236169414932,
59.9220933234976));
#218591=CARTESIAN_POINT('Ctrl Pts',(-54.7402366305299,69.2859982149144,
60.1958367009625));
#218592=CARTESIAN_POINT('Ctrl Pts',(-54.6243561549999,72.7344639571905,
61.9568044017577));
#218593=CARTESIAN_POINT('Ctrl Pts',(-54.5084756794709,75.2208721650242,
64.9250863686192));
#218594=CARTESIAN_POINT('Ctrl Pts',(-54.3925952039409,76.3500020236737,
68.6288667717324));
#218595=CARTESIAN_POINT('Ctrl Pts',(-54.2767147284109,75.9423755505674,
72.4794205229619));
#218596=CARTESIAN_POINT('Ctrl Pts',(-54.1608342528809,74.0627859826778,
75.8646925335889));
#218597=CARTESIAN_POINT('Ctrl Pts',(-54.0449537773509,71.0099987529967,
78.2465854069094));
#218598=CARTESIAN_POINT('Ctrl Pts',(-53.9290733018209,67.2692619766016,
79.2464913522907));
#218599=CARTESIAN_POINT('Ctrl Pts',(-53.8131928262909,63.4351750586927,
78.7054728353225));
#218600=CARTESIAN_POINT('Ctrl Pts',(-53.6973123507609,60.1171756413221,
76.7095260935192));
#218601=CARTESIAN_POINT('Ctrl Pts',(-53.5814318752309,57.8426679760259,
73.5759118207695));
#218602=CARTESIAN_POINT('Ctrl Pts',(-53.4655513997009,56.973190707635,69.8027257917525));
#218603=CARTESIAN_POINT('Ctrl Pts',(-53.3496709241709,57.6469494083309,
65.9897253009273));
#218604=CARTESIAN_POINT('Ctrl Pts',(-53.2337904486409,59.7568484585497,
62.7429962503755));
#218605=CARTESIAN_POINT('Ctrl Pts',(-53.1179099731109,62.9675141618542,
60.5786142897589));
#218606=CARTESIAN_POINT('Ctrl Pts',(-53.0020294975809,66.7686032272295,
59.8406133095026));
#218607=CARTESIAN_POINT('Ctrl Pts',(-52.8861490220609,70.5559231032727,
60.6463003991197));
#218608=CARTESIAN_POINT('Ctrl Pts',(-52.7702685465309,73.7274698854095,
62.8676095938355));
#218609=CARTESIAN_POINT('Ctrl Pts',(-52.6543880710009,75.7791183323543,
66.1514582779196));
#218610=CARTESIAN_POINT('Ctrl Pts',(-52.5385075954709,76.3847538257845,
69.9758705437336));
#218611=CARTESIAN_POINT('Ctrl Pts',(-52.4226271199409,75.4481090992107,
73.7329465591993));
#218612=CARTESIAN_POINT('Ctrl Pts',(-52.3067466444109,73.1180661591808,
76.8254897565408));
#218613=CARTESIAN_POINT('Ctrl Pts',(-52.1908661688809,69.7649911204159,
78.7619327105721));
#218614=CARTESIAN_POINT('Ctrl Pts',(-52.0749856933509,65.9218635916335,
79.2344730023141));
#218615=CARTESIAN_POINT('Ctrl Pts',(-51.9591052178209,62.1995582424626,
78.1679991782881));
#218616=CARTESIAN_POINT('Ctrl Pts',(-51.8432247422909,59.1897447568815,
75.7320299026639));
#218617=CARTESIAN_POINT('Ctrl Pts',(-51.7273442667609,57.3708404668259,
72.3137685443966));
#218618=CARTESIAN_POINT('Ctrl Pts',(-51.6114637912309,57.0319647285943,
68.4565562396562));
#218619=CARTESIAN_POINT('Ctrl Pts',(-51.4955833157009,58.2269826827762,
64.7735064682079));
#218620=CARTESIAN_POINT('Ctrl Pts',(-51.3797028401709,60.7659432563194,
61.8500491424068));
#218621=CARTESIAN_POINT('Ctrl Pts',(-51.2638223646409,64.2452723575601,
60.1508750680324));
#218622=CARTESIAN_POINT('Ctrl Pts',(-51.1479418891109,68.1119219808598,
59.9460721861075));
#218623=CARTESIAN_POINT('Ctrl Pts',(-51.0320614135809,71.7512785612103,
61.2681944235776));
#218624=CARTESIAN_POINT('Ctrl Pts',(-50.9161809380509,74.5848573275517,
63.9070871657535));
#218625=CARTESIAN_POINT('Ctrl Pts',(-50.8003004625309,76.162253894446,67.4432918544721));
#218626=CARTESIAN_POINT('Ctrl Pts',(-50.6844199870009,76.2327371582677,
71.3147199681373));
#218627=CARTESIAN_POINT('Ctrl Pts',(-50.5685395114709,74.7851036291041,
74.9059983888393));
#218628=CARTESIAN_POINT('Ctrl Pts',(-50.4526590359409,72.0494582533172,
77.6462844884435));
#218629=CARTESIAN_POINT('Ctrl Pts',(-50.3367785604109,68.4606386605805,
79.1000029826967));
#218630=CARTESIAN_POINT('Ctrl Pts',(-50.2208980848809,64.5890966422126,
79.0360817049179));
#218631=CARTESIAN_POINT('Ctrl Pts',(-50.1050176093509,61.0502234215632,
77.4646811010362));
#218632=CARTESIAN_POINT('Ctrl Pts',(-49.9891371338209,58.4065316900025,
74.6355792014605));
#218633=CARTESIAN_POINT('Ctrl Pts',(-49.8732566582909,57.0782428169735,
70.9984687825245));
#218634=CARTESIAN_POINT('Ctrl Pts',(-49.7573761827609,57.2764916192201,
67.1314775823678));
#218635=CARTESIAN_POINT('Ctrl Pts',(-49.6414957072309,58.9697659570288,
63.6492734604498));
#218636=CARTESIAN_POINT('Ctrl Pts',(-49.5256152317109,61.8889156671989,
61.105361414176));
#218637=CARTESIAN_POINT('Ctrl Pts',(-49.4097347561809,65.5699346500343,
59.9041025837992));
#218638=CARTESIAN_POINT('Ctrl Pts',(-49.2938542806509,69.4277157925497,
60.2364400462553));
#218639=CARTESIAN_POINT('Ctrl Pts',(-49.1779738051209,72.8490551950089,
62.0495479319754));
#218640=CARTESIAN_POINT('Ctrl Pts',(-49.0620933295909,75.2901224652598,
65.055228253093));
#218641=CARTESIAN_POINT('Ctrl Pts',(-48.9462128540609,76.3629038700644,
68.7757205963566));
#218642=CARTESIAN_POINT('Ctrl Pts',(-48.8303323785309,75.8968782343273,
72.6196436763184));
#218643=CARTESIAN_POINT('Ctrl Pts',(-48.7144519030009,73.966121137307,75.9759955596776));
#218644=CARTESIAN_POINT('Ctrl Pts',(-48.5985714274709,70.8775325360307,
78.3112787937738));
#218645=CARTESIAN_POINT('Ctrl Pts',(-48.4826909519509,67.1220463396723,
79.254283040401));
#218646=CARTESIAN_POINT('Ctrl Pts',(-48.3668104764209,63.2966247837026,
78.6551574757722));
#218647=CARTESIAN_POINT('Ctrl Pts',(-48.2509300008909,60.0092595589126,
76.6089776856617));
#218648=CARTESIAN_POINT('Ctrl Pts',(-48.1736763505409,58.5249141491315,
74.4973756505227));
#218649=CARTESIAN_POINT('Ctrl Pts',(-48.1350495253609,58.0183752164734,
73.3382509378444));
#218650=CARTESIAN_POINT('Ctrl Pts',(-55.3272718489599,61.0726603761865,
77.6919120683442));
#218651=CARTESIAN_POINT('Ctrl Pts',(-55.2886450237839,59.9836344637329,
76.9414276436267));
#218652=CARTESIAN_POINT('Ctrl Pts',(-55.2113913734309,58.1114300002093,
74.9978312579017));
#218653=CARTESIAN_POINT('Ctrl Pts',(-55.0955108979009,56.6649993918269,
71.2165482676822));
#218654=CARTESIAN_POINT('Ctrl Pts',(-54.9796304223719,56.8109087960282,
67.1708003444752));
#218655=CARTESIAN_POINT('Ctrl Pts',(-54.8637499468419,58.5258181284236,
63.5035675795475));
#218656=CARTESIAN_POINT('Ctrl Pts',(-54.7478694713129,61.5371777912702,
60.7977929546753));
#218657=CARTESIAN_POINT('Ctrl Pts',(-54.6319889957829,65.3663140994574,
59.4835587753602));
#218658=CARTESIAN_POINT('Ctrl Pts',(-54.5161085202509,69.4045791587436,
59.7697677843113));
#218659=CARTESIAN_POINT('Ctrl Pts',(-54.4002280447209,73.0100799442327,
61.6109258247082));
#218660=CARTESIAN_POINT('Ctrl Pts',(-54.2843475691909,75.6097133511933,
64.7143763916865));
#218661=CARTESIAN_POINT('Ctrl Pts',(-54.1684670936609,76.7902611357812,
68.58681826895));
#218662=CARTESIAN_POINT('Ctrl Pts',(-54.0525866181309,76.3640723089752,
72.612717208417));
#218663=CARTESIAN_POINT('Ctrl Pts',(-53.9367061426009,74.3988906398205,
76.152146567904));
#218664=CARTESIAN_POINT('Ctrl Pts',(-53.8208256670709,71.2070866385185,
78.6425052571067));
#218665=CARTESIAN_POINT('Ctrl Pts',(-53.7049451915509,67.2960054813953,
79.6879445744451));
#218666=CARTESIAN_POINT('Ctrl Pts',(-53.5890647160209,63.2873232362219,
79.1222893429069));
#218667=CARTESIAN_POINT('Ctrl Pts',(-53.4731842404909,59.8182299061273,
77.035451866986));
#218668=CARTESIAN_POINT('Ctrl Pts',(-53.3573037649609,57.4401464955149,
73.7591401486176));
#218669=CARTESIAN_POINT('Ctrl Pts',(-53.2414232894309,56.5310752712668,
69.8141320760029));
#218670=CARTESIAN_POINT('Ctrl Pts',(-53.1255428139009,57.235515363221,65.8274964843525));
#218671=CARTESIAN_POINT('Ctrl Pts',(-53.0096623383709,59.4414942684621,
62.4329190064619));
#218672=CARTESIAN_POINT('Ctrl Pts',(-52.8937818628409,62.7983661588541,
60.1699761668686));
#218673=CARTESIAN_POINT('Ctrl Pts',(-52.7779013873109,66.7725479066749,
59.398368352605));
#218674=CARTESIAN_POINT('Ctrl Pts',(-52.6620209117809,70.7323334485579,
60.2407445429475));
#218675=CARTESIAN_POINT('Ctrl Pts',(-52.5461404362509,74.0483050338323,
62.5632069494067));
#218676=CARTESIAN_POINT('Ctrl Pts',(-52.4302599607209,76.1933807399002,
65.9965944019083));
#218677=CARTESIAN_POINT('Ctrl Pts',(-52.3143794851909,76.8265954534646,
69.9951614340195));
#218678=CARTESIAN_POINT('Ctrl Pts',(-52.1984990096609,75.84729812247,73.9233258808397));
#218679=CARTESIAN_POINT('Ctrl Pts',(-52.0826185341309,73.4111504909153,
77.1566962433291));
#218680=CARTESIAN_POINT('Ctrl Pts',(-51.9667380586009,69.9053842778755,
79.1813202684909));
#218681=CARTESIAN_POINT('Ctrl Pts',(-51.8508575830709,65.8872497336091,
79.6753789369893));
#218682=CARTESIAN_POINT('Ctrl Pts',(-51.7349771075409,61.9954393276913,
78.5603403958908));
#218683=CARTESIAN_POINT('Ctrl Pts',(-51.6190966320109,58.8485659940342,
76.0134427918172));
#218684=CARTESIAN_POINT('Ctrl Pts',(-51.5032161564809,56.946833067975,72.4395218271453));
#218685=CARTESIAN_POINT('Ctrl Pts',(-51.3873356809509,56.5925257233132,
68.4066611192533));
#218686=CARTESIAN_POINT('Ctrl Pts',(-51.2714552054309,57.8419619928253,
64.5558938980169));
#218687=CARTESIAN_POINT('Ctrl Pts',(-51.1555747299009,60.4965408770102,
61.4993091811534));
#218688=CARTESIAN_POINT('Ctrl Pts',(-51.0396942543709,64.1343104664627,
59.7227587040345));
#218689=CARTESIAN_POINT('Ctrl Pts',(-50.9238137788409,68.1770382462698,
59.5086295791555));
#218690=CARTESIAN_POINT('Ctrl Pts',(-50.8079333033109,71.9821225909486,
60.8909581629449));
#218691=CARTESIAN_POINT('Ctrl Pts',(-50.6920528277809,74.9447358895156,
63.6500198923846));
#218692=CARTESIAN_POINT('Ctrl Pts',(-50.5761723522509,76.5939633970318,
67.3472550501956));
#218693=CARTESIAN_POINT('Ctrl Pts',(-50.4602918767209,76.6676563033805,
71.3949789216125));
#218694=CARTESIAN_POINT('Ctrl Pts',(-50.3444114011909,75.1541009379953,
75.1497957399931));
#218695=CARTESIAN_POINT('Ctrl Pts',(-50.2285309256609,72.2938806868999,
78.0148680425532));
#218696=CARTESIAN_POINT('Ctrl Pts',(-50.1126504501309,68.5416346657267,
79.534785468025));
#218697=CARTESIAN_POINT('Ctrl Pts',(-49.9967699746009,64.4937917026564,
79.4679533651302));
#218698=CARTESIAN_POINT('Ctrl Pts',(-49.8808894990709,60.7937664942429,
77.8249948626797));
#218699=CARTESIAN_POINT('Ctrl Pts',(-49.7650090235509,58.0296872407287,
74.8670622968579));
#218700=CARTESIAN_POINT('Ctrl Pts',(-49.6491285480209,56.6409112073073,
71.0643263985101));
#218701=CARTESIAN_POINT('Ctrl Pts',(-49.5332480724909,56.8481877951267,
67.0212414872383));
#218702=CARTESIAN_POINT('Ctrl Pts',(-49.4173675969609,58.6185698755448,
63.3804659554293));
#218703=CARTESIAN_POINT('Ctrl Pts',(-49.3014871214309,61.6706508180947,
60.7207101200916));
#218704=CARTESIAN_POINT('Ctrl Pts',(-49.1856066459009,65.5192947733674,
59.4647487795595));
#218705=CARTESIAN_POINT('Ctrl Pts',(-49.0697261703709,69.552750222577,59.8122201107395));
#218706=CARTESIAN_POINT('Ctrl Pts',(-48.9538456948409,73.1298893983293,
61.7078926778295));
#218707=CARTESIAN_POINT('Ctrl Pts',(-48.8379652193109,75.6821171477224,
64.8504446324208));
#218708=CARTESIAN_POINT('Ctrl Pts',(-48.7220847437809,76.8037505020027,
68.7403594723971));
#218709=CARTESIAN_POINT('Ctrl Pts',(-48.6062042682609,76.3165031516395,
72.7593257953694));
#218710=CARTESIAN_POINT('Ctrl Pts',(-48.4903237927309,74.2978239040633,
76.2685180728018));
#218711=CARTESIAN_POINT('Ctrl Pts',(-48.3744433172009,71.0685882206619,
78.7101446291031));
#218712=CARTESIAN_POINT('Ctrl Pts',(-48.2585628416709,67.1420859895845,
79.6960910777589));
#218713=CARTESIAN_POINT('Ctrl Pts',(-48.1426823661409,63.1424637066209,
79.0696827398739));
#218714=CARTESIAN_POINT('Ctrl Pts',(-48.0268018906109,59.7053995784171,
76.9303247204408));
#218715=CARTESIAN_POINT('Ctrl Pts',(-47.9495482402609,58.1534605594795,
74.7225652803545));
#218716=CARTESIAN_POINT('Ctrl Pts',(-47.9109214150809,57.6238550316623,
73.5106567464228));
#218717=CARTESIAN_POINT('Ctrl Pts',(-55.1031437386839,60.8283504752015,
78.0464295027996));
#218718=CARTESIAN_POINT('Ctrl Pts',(-55.0645169135079,59.6918928073868,
77.2632582583922));
#218719=CARTESIAN_POINT('Ctrl Pts',(-54.9872632631549,57.7381457991904,
75.2350099031933));
#218720=CARTESIAN_POINT('Ctrl Pts',(-54.8713827876249,56.2287169260511,
71.289035799845));
#218721=CARTESIAN_POINT('Ctrl Pts',(-54.7555023120959,56.3809813114179,
67.0670781799153));
#218722=CARTESIAN_POINT('Ctrl Pts',(-54.6396218365659,58.1705823100065,
63.2401216789652));
#218723=CARTESIAN_POINT('Ctrl Pts',(-54.5237413610409,61.313099618598,60.4164989490926));
#218724=CARTESIAN_POINT('Ctrl Pts',(-54.4078608855109,65.30901125743,59.0450242272283));
#218725=CARTESIAN_POINT('Ctrl Pts',(-54.2919804099809,69.5231601025766,
59.3436988676508));
#218726=CARTESIAN_POINT('Ctrl Pts',(-54.1760999344509,73.2856959312731,
61.2650472476525));
#218727=CARTESIAN_POINT('Ctrl Pts',(-54.0602194589209,75.9985545373602,
64.5036664147486));
#218728=CARTESIAN_POINT('Ctrl Pts',(-53.9443389833909,77.2305202478881,
68.5447697661598));
#218729=CARTESIAN_POINT('Ctrl Pts',(-53.8284585078609,76.7857690673864,
72.746013893864));
#218730=CARTESIAN_POINT('Ctrl Pts',(-53.7125780323309,74.7349952969698,
76.4396006022122));
#218731=CARTESIAN_POINT('Ctrl Pts',(-53.5966975568009,71.4041745240506,
79.0384251072975));
#218732=CARTESIAN_POINT('Ctrl Pts',(-53.4808170812709,67.3227489862028,
80.1293977965976));
#218733=CARTESIAN_POINT('Ctrl Pts',(-53.3649366057409,63.1394714137716,
79.5391058504835));
#218734=CARTESIAN_POINT('Ctrl Pts',(-53.2490561302109,59.5192841709575,
77.3613776404707));
#218735=CARTESIAN_POINT('Ctrl Pts',(-53.1331756546809,57.0376250150175,
73.9423684764854));
#218736=CARTESIAN_POINT('Ctrl Pts',(-53.0172951791509,56.0889598348911,
69.8255383602719));
#218737=CARTESIAN_POINT('Ctrl Pts',(-52.9014147036209,56.8240813181107,
65.6652676678047));
#218738=CARTESIAN_POINT('Ctrl Pts',(-52.7855342280909,59.1261400783554,
62.1228417625685));
#218739=CARTESIAN_POINT('Ctrl Pts',(-52.6696537525609,62.6292181558182,
59.7613380439862));
#218740=CARTESIAN_POINT('Ctrl Pts',(-52.5537732770309,66.776492586088,58.9561233957071));
#218741=CARTESIAN_POINT('Ctrl Pts',(-52.4378928015009,70.9087437938121,
59.8351886867614));
#218742=CARTESIAN_POINT('Ctrl Pts',(-52.3220123259709,74.3691401822294,
62.258804304951));
#218743=CARTESIAN_POINT('Ctrl Pts',(-52.2061318504409,76.6076431474328,
65.8417305258611));
#218744=CARTESIAN_POINT('Ctrl Pts',(-52.0902513749109,77.2684370811464,
70.014452324264));
#218745=CARTESIAN_POINT('Ctrl Pts',(-51.9743708993809,76.2464871457476,
74.1137052024411));
#218746=CARTESIAN_POINT('Ctrl Pts',(-51.8584904238609,73.7042348226836,
77.487902730087));
#218747=CARTESIAN_POINT('Ctrl Pts',(-51.7426099483309,70.0457774353802,
79.6007078263948));
#218748=CARTESIAN_POINT('Ctrl Pts',(-51.6267294728009,65.8526358756345,
80.1162848716646));
#218749=CARTESIAN_POINT('Ctrl Pts',(-51.5108489972709,61.7913204129621,
78.9526816135228));
#218750=CARTESIAN_POINT('Ctrl Pts',(-51.3949685217409,58.5073872312147,
76.2948556810079));
#218751=CARTESIAN_POINT('Ctrl Pts',(-51.2790880462109,56.522825669145,72.5652751099482));
#218752=CARTESIAN_POINT('Ctrl Pts',(-51.1632075706809,56.15308671803,68.356765998908));
#218753=CARTESIAN_POINT('Ctrl Pts',(-51.0473270951509,57.4569413028341,
64.3382813278711));
#218754=CARTESIAN_POINT('Ctrl Pts',(-50.9314466196209,60.2271384976534,
61.1485692199367));
#218755=CARTESIAN_POINT('Ctrl Pts',(-50.8155661440909,64.0233485753049,
59.2946423400516));
#218756=CARTESIAN_POINT('Ctrl Pts',(-50.6996856685609,68.2421545116176,
59.0711869721972));
#218757=CARTESIAN_POINT('Ctrl Pts',(-50.5838051930309,72.2129666206316,
60.5137219022862));
#218758=CARTESIAN_POINT('Ctrl Pts',(-50.4679247175009,75.3046144514435,
63.3929526189662));
#218759=CARTESIAN_POINT('Ctrl Pts',(-50.3520442419709,77.0256728996043,
67.2512182458574));
#218760=CARTESIAN_POINT('Ctrl Pts',(-50.2361637664409,77.1025754485052,
71.4752378750256));
#218761=CARTESIAN_POINT('Ctrl Pts',(-50.1202832909109,75.5230982469212,
75.3935930910952));
#218762=CARTESIAN_POINT('Ctrl Pts',(-50.0044028153909,72.5383031205348,
78.3834515966281));
#218763=CARTESIAN_POINT('Ctrl Pts',(-49.8885223398609,68.6226306709332,
79.9695679533436));
#218764=CARTESIAN_POINT('Ctrl Pts',(-49.7726418643309,64.3984867631581,
79.8998250253566));
#218765=CARTESIAN_POINT('Ctrl Pts',(-49.6567613888009,60.537309566982,78.1853086243629));
#218766=CARTESIAN_POINT('Ctrl Pts',(-49.5408809132709,57.6528427914971,
75.0985453923105));
#218767=CARTESIAN_POINT('Ctrl Pts',(-49.4250004377409,56.2035795976409,
71.1301840145486));
#218768=CARTESIAN_POINT('Ctrl Pts',(-49.3091199622109,56.4198839710304,
66.9110053921681));
#218769=CARTESIAN_POINT('Ctrl Pts',(-49.1932394866809,58.2673737940418,
63.111658450455));
#218770=CARTESIAN_POINT('Ctrl Pts',(-49.0773590111509,61.4523859689387,
60.336058826028));
#218771=CARTESIAN_POINT('Ctrl Pts',(-48.9614785356209,65.4686548966643,
59.0253949753286));
#218772=CARTESIAN_POINT('Ctrl Pts',(-48.8455980601009,69.6777846525631,
59.3880001752186));
#218773=CARTESIAN_POINT('Ctrl Pts',(-48.7297175845709,73.4107236016189,
61.366237423659));
#218774=CARTESIAN_POINT('Ctrl Pts',(-48.6138371090409,76.0741118301684,
64.6456610117157));
#218775=CARTESIAN_POINT('Ctrl Pts',(-48.4979566335109,77.2445971339387,
68.7049983484055));
#218776=CARTESIAN_POINT('Ctrl Pts',(-48.3820761579809,76.7361280689603,
72.8990079143937));
#218777=CARTESIAN_POINT('Ctrl Pts',(-48.2661956824509,74.6295266708348,
76.5610405859094));
#218778=CARTESIAN_POINT('Ctrl Pts',(-48.1503152069209,71.2596439053081,
79.1090104644245));
#218779=CARTESIAN_POINT('Ctrl Pts',(-48.0344347313909,67.1621256395096,
80.1378991151167));
#218780=CARTESIAN_POINT('Ctrl Pts',(-47.9185542558709,62.9883026295467,
79.4842080039734));
#218781=CARTESIAN_POINT('Ctrl Pts',(-47.8026737803409,59.4015395979127,
77.2516717552151));
#218782=CARTESIAN_POINT('Ctrl Pts',(-47.7254201299809,57.7820069698283,
74.9477549101844));
#218783=CARTESIAN_POINT('Ctrl Pts',(-47.6867933048109,57.2293348468531,
73.6830625549967));
#218784=CARTESIAN_POINT('',(-55.5975553638665,58.5901119100723,73.6973239050991));
#218785=CARTESIAN_POINT('Ctrl Pts',(-62.9066342559309,58.9178549548062,
74.1516175606608));
#218786=CARTESIAN_POINT('Ctrl Pts',(-62.8680074307549,58.3024937106637,
73.11283644396));
#218787=CARTESIAN_POINT('Ctrl Pts',(-62.7907537804019,57.4946548944447,
70.7854776041952));
#218788=CARTESIAN_POINT('Ctrl Pts',(-62.6748733048729,57.7429994225583,
67.098000141731));
#218789=CARTESIAN_POINT('Ctrl Pts',(-62.5589928293429,59.4122826098446,
63.8007419836913));
#218790=CARTESIAN_POINT('Ctrl Pts',(-62.4431123538139,62.2370844442565,
61.4176698865354));
#218791=CARTESIAN_POINT('Ctrl Pts',(-62.3272318782849,65.7684179761418,
60.3276167603848));
#218792=CARTESIAN_POINT('Ctrl Pts',(-62.2113514027559,69.4449629855937,
60.7038391619823));
#218793=CARTESIAN_POINT('Ctrl Pts',(-62.0954709272259,72.6823251108832,
62.4865383110415));
#218794=CARTESIAN_POINT('Ctrl Pts',(-61.9795904516969,74.9659171689976,
65.3923490235231));
#218795=CARTESIAN_POINT('Ctrl Pts',(-61.8637099761679,75.9327566433709,
68.959385660905));
#218796=CARTESIAN_POINT('Ctrl Pts',(-61.7478295006379,75.429161966439,72.6206588347031));
#218797=CARTESIAN_POINT('Ctrl Pts',(-61.6319490251089,73.5351807716313,
75.7942000908075));
#218798=CARTESIAN_POINT('Ctrl Pts',(-61.5160685495799,70.5518660735791,
77.9755671576036));
#218799=CARTESIAN_POINT('Ctrl Pts',(-61.4001880740499,66.9534231567007,
78.8180263208339));
#218800=CARTESIAN_POINT('Ctrl Pts',(-61.2843075985209,63.3118334634422,
78.1876666029973));
#218801=CARTESIAN_POINT('Ctrl Pts',(-61.1684271229909,60.2059367237536,
76.1846852475529));
#218802=CARTESIAN_POINT('Ctrl Pts',(-61.0525466474619,58.1294229415569,
73.1274611176965));
#218803=CARTESIAN_POINT('Ctrl Pts',(-60.9366661719329,57.4123591419893,
69.5019475850797));
#218804=CARTESIAN_POINT('Ctrl Pts',(-60.8207856964029,58.1687243976584,
65.8844290339352));
#218805=CARTESIAN_POINT('Ctrl Pts',(-60.7049052208739,60.2782925718688,
62.8499190263368));
#218806=CARTESIAN_POINT('Ctrl Pts',(-60.5890247453439,63.4057425617159,
60.8807604677571));
#218807=CARTESIAN_POINT('Ctrl Pts',(-60.4731442698149,67.0539584206267,
60.2899560038079));
#218808=CARTESIAN_POINT('Ctrl Pts',(-60.3572637942849,70.6430471731958,
61.1714154719933));
#218809=CARTESIAN_POINT('Ctrl Pts',(-60.2413833187559,73.6025142444707,
63.3850286996998));
#218810=CARTESIAN_POINT('Ctrl Pts',(-60.1255028432259,75.4619449901604,
66.5789363642741));
#218811=CARTESIAN_POINT('Ctrl Pts',(-60.0096223676969,75.9257782731553,
70.2454589066056));
#218812=CARTESIAN_POINT('Ctrl Pts',(-59.8937418921669,74.9202866406472,
73.8017934584711));
#218813=CARTESIAN_POINT('Ctrl Pts',(-59.7778614166379,72.6052954859447,
76.6826518065131));
#218814=CARTESIAN_POINT('Ctrl Pts',(-59.6619809411079,69.34877840509,78.4301143583121));
#218815=CARTESIAN_POINT('Ctrl Pts',(-59.5461004655789,65.6683668794744,
78.7664175993805));
#218816=CARTESIAN_POINT('Ctrl Pts',(-59.4302199900499,62.149071465724,77.6381052939462));
#218817=CARTESIAN_POINT('Ctrl Pts',(-59.3143395145199,59.3502929141666,
75.224525486451));
#218818=CARTESIAN_POINT('Ctrl Pts',(-59.1984590389909,57.7169040296169,
71.9093226842531));
#218819=CARTESIAN_POINT('Ctrl Pts',(-59.0825785634609,57.5085360337358,
68.219456609976));
#218820=CARTESIAN_POINT('Ctrl Pts',(-58.9666980879319,58.7583095371751,
64.7414406442363));
#218821=CARTESIAN_POINT('Ctrl Pts',(-58.8508176124019,61.2675699362972,
62.0281140665389));
#218822=CARTESIAN_POINT('Ctrl Pts',(-58.7349371368729,64.6374640559506,
60.5107668781401));
#218823=CARTESIAN_POINT('Ctrl Pts',(-58.6190566613429,68.3323388527351,
60.4305851847563));
#218824=CARTESIAN_POINT('Ctrl Pts',(-58.5031761858139,71.7648847971213,
61.8003140657714));
#218825=CARTESIAN_POINT('Ctrl Pts',(-58.3872957102849,74.3894901824946,
64.4022317122195));
#218826=CARTESIAN_POINT('Ctrl Pts',(-58.2714152347549,75.7889674615547,
67.8227568492751));
#218827=CARTESIAN_POINT('Ctrl Pts',(-58.1555347592259,75.740866243548,71.5181885075058));
#218828=CARTESIAN_POINT('Ctrl Pts',(-58.0396542836959,74.2528323365911,
74.9011286428881));
#218829=CARTESIAN_POINT('Ctrl Pts',(-57.9237738081669,71.5613924274766,
77.4338505153925));
#218830=CARTESIAN_POINT('Ctrl Pts',(-57.8078933326379,68.0943575771148,
78.7137716903922));
#218831=CARTESIAN_POINT('Ctrl Pts',(-57.6920128571079,64.4028215894282,
78.5374455169307));
#218832=CARTESIAN_POINT('Ctrl Pts',(-57.5761323815789,61.0735632819335,
76.9328994783959));
#218833=CARTESIAN_POINT('Ctrl Pts',(-57.4602519060499,58.6357765347184,
74.1551801543823));
#218834=CARTESIAN_POINT('Ctrl Pts',(-57.3443714305209,57.4769536083849,
70.6458129331832));
#218835=CARTESIAN_POINT('Ctrl Pts',(-57.2284909549909,57.7812922863604,
66.9626204542406));
#218836=CARTESIAN_POINT('Ctrl Pts',(-57.1126104794619,59.5004171796032,
63.6910553136322));
#218837=CARTESIAN_POINT('Ctrl Pts',(-56.9967300039329,62.3610691148619,
61.3511409192107));
#218838=CARTESIAN_POINT('Ctrl Pts',(-56.8808495284039,65.908540359229,60.3148124779815));
#218839=CARTESIAN_POINT('Ctrl Pts',(-56.7649690528749,69.5789515441067,
60.7467969703095));
#218840=CARTESIAN_POINT('Ctrl Pts',(-56.6490885773459,72.7888816918543,
62.5784293889601));
#218841=CARTESIAN_POINT('Ctrl Pts',(-56.5332081018169,75.0281044299382,
65.5185672056338));
#218842=CARTESIAN_POINT('Ctrl Pts',(-56.4173276262869,75.9406897400636,
69.0998682252856));
#218843=CARTESIAN_POINT('Ctrl Pts',(-56.3014471507579,75.3815799209528,
72.7530756919933));
#218844=CARTESIAN_POINT('Ctrl Pts',(-56.1855666752289,73.439646862909,75.8975034275876));
#218845=CARTESIAN_POINT('Ctrl Pts',(-56.0696861997009,70.4235656679413,
78.0333359882836));
#218846=CARTESIAN_POINT('Ctrl Pts',(-55.9538057241719,66.81274987119,78.8210806253173));
#218847=CARTESIAN_POINT('Ctrl Pts',(-55.8379252486429,63.1811478570346,
78.1355116392279));
#218848=CARTESIAN_POINT('Ctrl Pts',(-55.7220447731139,60.1060108866471,
76.0856457086154));
#218849=CARTESIAN_POINT('Ctrl Pts',(-55.6061642975849,58.0761429897366,
72.9971507091326));
#218850=CARTESIAN_POINT('Ctrl Pts',(-55.5289106472319,57.6348370927523,
70.5734238624516));
#218851=CARTESIAN_POINT('Ctrl Pts',(-55.4902838220559,57.6597134706593,
69.3663129168428));
#218852=CARTESIAN_POINT('Ctrl Pts',(-62.6825061456549,58.547426526001,74.3710548368581));
#218853=CARTESIAN_POINT('Ctrl Pts',(-62.6438793204789,57.9027062315234,
73.282713193911));
#218854=CARTESIAN_POINT('Ctrl Pts',(-62.5666256701259,57.0563252082828,
70.8443154384342));
#218855=CARTESIAN_POINT('Ctrl Pts',(-62.4507451945969,57.3165183205799,
66.9809074352464));
#218856=CARTESIAN_POINT('Ctrl Pts',(-62.3348647190669,59.0654434573398,
63.5263362043602));
#218857=CARTESIAN_POINT('Ctrl Pts',(-62.2189842435379,62.0250173464219,
61.0295670970088));
#218858=CARTESIAN_POINT('Ctrl Pts',(-62.1031037680089,65.7248317501465,
59.8875072432628));
#218859=CARTESIAN_POINT('Ctrl Pts',(-61.9872232924799,69.5767857100507,
60.2816793167476));
#218860=CARTESIAN_POINT('Ctrl Pts',(-61.8713428169499,72.9686032523646,
62.1494315213011));
#218861=CARTESIAN_POINT('Ctrl Pts',(-61.7554623414209,75.3611461012774,
65.1938792437982));
#218862=CARTESIAN_POINT('Ctrl Pts',(-61.6395818658919,76.3741137468067,
68.9311001577751));
#218863=CARTESIAN_POINT('Ctrl Pts',(-61.5237013903619,75.8464924324996,
72.7670536586459));
#218864=CARTESIAN_POINT('Ctrl Pts',(-61.4078209148329,73.862148885889,76.0920054209542));
#218865=CARTESIAN_POINT('Ctrl Pts',(-61.2919404393039,70.73649944184,78.3774460967396));
#218866=CARTESIAN_POINT('Ctrl Pts',(-61.1760599637739,66.9663738463322,
79.2600992130555));
#218867=CARTESIAN_POINT('Ctrl Pts',(-61.0601794882449,63.1510429301467,
78.5996648636749));
#218868=CARTESIAN_POINT('Ctrl Pts',(-60.9442990127149,59.8969630223145,
76.5011207294713));
#218869=CARTESIAN_POINT('Ctrl Pts',(-60.8284185371859,57.7213782095142,
73.2980356147634));
#218870=CARTESIAN_POINT('Ctrl Pts',(-60.7125380616569,56.9701031033569,
69.4995478571637));
#218871=CARTESIAN_POINT('Ctrl Pts',(-60.5966575861269,57.7625547486447,
65.7094365237527));
#218872=CARTESIAN_POINT('Ctrl Pts',(-60.4807771105979,59.9727709873792,
62.5301492281794));
#218873=CARTESIAN_POINT('Ctrl Pts',(-60.3648966350679,63.2494324567334,
60.4670415855671));
#218874=CARTESIAN_POINT('Ctrl Pts',(-60.2490161595389,67.0717056747189,
59.8480496818693));
#218875=CARTESIAN_POINT('Ctrl Pts',(-60.1331356840089,70.8320308162221,
60.7715638181682));
#218876=CARTESIAN_POINT('Ctrl Pts',(-60.0172552084799,73.9326948568119,
63.090789127866));
#218877=CARTESIAN_POINT('Ctrl Pts',(-59.9013747329499,75.8808395430932,
66.4370789854654));
#218878=CARTESIAN_POINT('Ctrl Pts',(-59.7854942574209,76.3668024366729,
70.2785323036529));
#218879=CARTESIAN_POINT('Ctrl Pts',(-59.6696137818909,75.3133385281575,
74.004540532737));
#218880=CARTESIAN_POINT('Ctrl Pts',(-59.5537333063619,72.887898523321,77.0228454067829));
#218881=CARTESIAN_POINT('Ctrl Pts',(-59.4378528308319,69.4760121373647,
78.8536798665508));
#218882=CARTESIAN_POINT('Ctrl Pts',(-59.3219723553029,65.6200071887684,
79.2060282256323));
#218883=CARTESIAN_POINT('Ctrl Pts',(-59.2060918797729,61.9328052450312,
78.023883836878));
#218884=CARTESIAN_POINT('Ctrl Pts',(-59.0902114042439,59.0004962166207,
75.4951514881296));
#218885=CARTESIAN_POINT('Ctrl Pts',(-58.9743309287149,57.2891779094226,
72.0217794692935));
#218886=CARTESIAN_POINT('Ctrl Pts',(-58.8584504531849,57.0708686204521,
68.1558688929745));
#218887=CARTESIAN_POINT('Ctrl Pts',(-58.7425699776559,58.3802691536199,
64.5119158508119));
#218888=CARTESIAN_POINT('Ctrl Pts',(-58.6266895021259,61.0092470407258,
61.6691357328929));
#218889=CARTESIAN_POINT('Ctrl Pts',(-58.5108090265969,64.5399197144825,
60.0793955023591));
#218890=CARTESIAN_POINT('Ctrl Pts',(-58.3949285510669,68.4110779807901,
59.9953883188285));
#218891=CARTESIAN_POINT('Ctrl Pts',(-58.2790480755379,72.0073916146724,
61.4304673328671));
#218892=CARTESIAN_POINT('Ctrl Pts',(-58.1631676000089,74.7572176283345,
64.1565231694807));
#218893=CARTESIAN_POINT('Ctrl Pts',(-58.0472871244789,76.2234643444835,
67.7402424800746));
#218894=CARTESIAN_POINT('Ctrl Pts',(-57.9314066489499,76.1730682044392,
71.6119841758516));
#218895=CARTESIAN_POINT('Ctrl Pts',(-57.8155261734199,74.6140397998802,
75.1563252942433));
#218896=CARTESIAN_POINT('Ctrl Pts',(-57.6996456978909,71.7941905693904,
77.8098840079436));
#218897=CARTESIAN_POINT('Ctrl Pts',(-57.5837652223619,68.1617425545688,
79.1508705661768));
#218898=CARTESIAN_POINT('Ctrl Pts',(-57.4678847468319,64.2940823928253,
78.9661318235942));
#218899=CARTESIAN_POINT('Ctrl Pts',(-57.3520042713029,60.8059842767521,
77.2850324623464));
#218900=CARTESIAN_POINT('Ctrl Pts',(-57.2361237957739,58.2518900686915,
74.3747874028885));
#218901=CARTESIAN_POINT('Ctrl Pts',(-57.1202433202449,57.0377793891086,
70.6979873284379));
#218902=CARTESIAN_POINT('Ctrl Pts',(-57.0043628447149,57.3566381471987,
66.8390687464839));
#218903=CARTESIAN_POINT('Ctrl Pts',(-56.8884823691859,59.157782951098,63.4114163537943));
#218904=CARTESIAN_POINT('Ctrl Pts',(-56.7726018936569,62.1549173589786,
60.9598640147741));
#218905=CARTESIAN_POINT('Ctrl Pts',(-56.6567214181279,65.8716394097845,
59.8740920651051));
#218906=CARTESIAN_POINT('Ctrl Pts',(-56.5408409425989,69.7171668986981,
60.326686653654));
#218907=CARTESIAN_POINT('Ctrl Pts',(-56.4249604670699,73.0802436764493,
62.2457067472407));
#218908=CARTESIAN_POINT('Ctrl Pts',(-56.3090799915409,75.4263003331489,
65.3261193292961));
#218909=CARTESIAN_POINT('Ctrl Pts',(-56.1931995160109,76.3824253336746,
69.0782851830545));
#218910=CARTESIAN_POINT('Ctrl Pts',(-56.0773190404819,75.7966402348364,
72.9057881597826));
#218911=CARTESIAN_POINT('Ctrl Pts',(-55.9614385649529,73.7620570287082,
76.2002373876932));
#218912=CARTESIAN_POINT('Ctrl Pts',(-55.8455580894239,70.6020777893704,
78.4379710938565));
#218913=CARTESIAN_POINT('Ctrl Pts',(-55.7296776138959,66.8189890005644,
79.2632992392267));
#218914=CARTESIAN_POINT('Ctrl Pts',(-55.6137971383669,63.0141222783363,
78.5450215725671));
#218915=CARTESIAN_POINT('Ctrl Pts',(-55.4979166628379,59.7922696966654,
76.3973559875148));
#218916=CARTESIAN_POINT('Ctrl Pts',(-55.3820361873089,57.6655562568715,
73.1615080615852));
#218917=CARTESIAN_POINT('Ctrl Pts',(-55.3047825369559,57.2031955369423,
70.6221445556835));
#218918=CARTESIAN_POINT('Ctrl Pts',(-55.2661557117799,57.2292587735241,
69.3574420224531));
#218919=CARTESIAN_POINT('Ctrl Pts',(-62.4583780353789,58.1769980971959,
74.5904921130554));
#218920=CARTESIAN_POINT('Ctrl Pts',(-62.4197512102019,57.5029187523924,
73.4525899438659));
#218921=CARTESIAN_POINT('Ctrl Pts',(-62.3424975598499,56.6179955221206,
70.9031532726741));
#218922=CARTESIAN_POINT('Ctrl Pts',(-62.2266170843209,56.8900372185927,
66.863814728757));
#218923=CARTESIAN_POINT('Ctrl Pts',(-62.1107366087909,58.7186043048254,
63.2519304250262));
#218924=CARTESIAN_POINT('Ctrl Pts',(-61.9948561332619,61.8129502485881,
60.6414643074804));
#218925=CARTESIAN_POINT('Ctrl Pts',(-61.8789756577329,65.6812455241418,
59.4473977261369));
#218926=CARTESIAN_POINT('Ctrl Pts',(-61.7630951822039,69.7086084345096,
59.8595194715137));
#218927=CARTESIAN_POINT('Ctrl Pts',(-61.6472147066739,73.2548813938479,
61.8123247315615));
#218928=CARTESIAN_POINT('Ctrl Pts',(-61.5313342311449,75.7563750335582,
64.9954094640758));
#218929=CARTESIAN_POINT('Ctrl Pts',(-61.4154537556159,76.8154708502427,
68.9028146546496));
#218930=CARTESIAN_POINT('Ctrl Pts',(-61.2995732800859,76.2638228985589,
72.9134484825934));
#218931=CARTESIAN_POINT('Ctrl Pts',(-61.1836928045569,74.1891170001427,
76.3898107511058));
#218932=CARTESIAN_POINT('Ctrl Pts',(-61.0678123290279,70.9211328100948,
78.7793250358796));
#218933=CARTESIAN_POINT('Ctrl Pts',(-60.9519318534979,66.9793245359562,
79.7021721052773));
#218934=CARTESIAN_POINT('Ctrl Pts',(-60.8360513779689,62.9902523968414,
79.0116631243529));
#218935=CARTESIAN_POINT('Ctrl Pts',(-60.7201709024389,59.5879893208676,
76.8175562113823));
#218936=CARTESIAN_POINT('Ctrl Pts',(-60.6042904269099,57.3133334774654,
73.4686101118191));
#218937=CARTESIAN_POINT('Ctrl Pts',(-60.4884099513809,56.5278470647294,
69.4971481292357));
#218938=CARTESIAN_POINT('Ctrl Pts',(-60.3725294758509,57.3563850996458,
65.5344440135604));
#218939=CARTESIAN_POINT('Ctrl Pts',(-60.2566490003219,59.667249402905,62.210379430011));
#218940=CARTESIAN_POINT('Ctrl Pts',(-60.1407685247919,63.0931223517737,
60.0533227033746));
#218941=CARTESIAN_POINT('Ctrl Pts',(-60.0248880492629,67.0894529288327,
59.4061433599309));
#218942=CARTESIAN_POINT('Ctrl Pts',(-59.9090075737329,71.0210144592654,
60.3717121643543));
#218943=CARTESIAN_POINT('Ctrl Pts',(-59.7931270982039,74.2628754691676,
62.796549556049));
#218944=CARTESIAN_POINT('Ctrl Pts',(-59.6772466226739,76.2997340960325,
66.2952216066778));
#218945=CARTESIAN_POINT('Ctrl Pts',(-59.5613661471449,76.8078266001889,
70.3116057007245));
#218946=CARTESIAN_POINT('Ctrl Pts',(-59.4454856716149,75.7063904156562,
74.2072876070264));
#218947=CARTESIAN_POINT('Ctrl Pts',(-59.3296051960859,73.1705015606764,
77.3630390070701));
#218948=CARTESIAN_POINT('Ctrl Pts',(-59.2137247205559,69.6032458696127,
79.277245374799));
#218949=CARTESIAN_POINT('Ctrl Pts',(-59.0978442450269,65.5716474980321,
79.6456388518812));
#218950=CARTESIAN_POINT('Ctrl Pts',(-58.9819637694969,61.7165390243107,
78.4096623797983));
#218951=CARTESIAN_POINT('Ctrl Pts',(-58.8660832939679,58.6506995190535,
75.765777489781));
#218952=CARTESIAN_POINT('Ctrl Pts',(-58.7502028184379,56.86145178922,72.1342362543012));
#218953=CARTESIAN_POINT('Ctrl Pts',(-58.6343223429089,56.6332012071813,
68.0922811759416));
#218954=CARTESIAN_POINT('Ctrl Pts',(-58.5184418673799,58.002228770078,64.2823910573551));
#218955=CARTESIAN_POINT('Ctrl Pts',(-58.4025613918499,60.7509241451938,
61.3101573992297));
#218956=CARTESIAN_POINT('Ctrl Pts',(-58.2866809163209,64.4423753730412,
59.6480241265653));
#218957=CARTESIAN_POINT('Ctrl Pts',(-58.1708004407909,68.4898171088944,
59.5601914529124));
#218958=CARTESIAN_POINT('Ctrl Pts',(-58.0549199652619,72.2498984322556,
61.0606205999848));
#218959=CARTESIAN_POINT('Ctrl Pts',(-57.9390394897319,75.1249450741959,
63.9108146267734));
#218960=CARTESIAN_POINT('Ctrl Pts',(-57.8231590142029,76.6579612274189,
67.6577281109137));
#218961=CARTESIAN_POINT('Ctrl Pts',(-57.7072785386739,76.6052701653223,
71.7057798442352));
#218962=CARTESIAN_POINT('Ctrl Pts',(-57.5913980631439,74.9752472631463,
75.4115219456312));
#218963=CARTESIAN_POINT('Ctrl Pts',(-57.4755175876149,72.0269887112709,
78.1859175005157));
#218964=CARTESIAN_POINT('Ctrl Pts',(-57.3596371120859,68.2291275319825,
79.5879694419675));
#218965=CARTESIAN_POINT('Ctrl Pts',(-57.2437566365559,64.1853431961846,
79.3948181302474));
#218966=CARTESIAN_POINT('Ctrl Pts',(-57.1278761610269,60.5384052715379,
77.6371654462714));
#218967=CARTESIAN_POINT('Ctrl Pts',(-57.0119956854979,57.8680036026363,
74.5943946513582));
#218968=CARTESIAN_POINT('Ctrl Pts',(-56.8961152099689,56.5986051698264,
70.7501617236546));
#218969=CARTESIAN_POINT('Ctrl Pts',(-56.7802347344389,56.9319840080419,
66.7155170386891));
#218970=CARTESIAN_POINT('Ctrl Pts',(-56.6643542589099,58.8151487226244,
63.1317773939326));
#218971=CARTESIAN_POINT('Ctrl Pts',(-56.5484737833809,61.9487656031238,
60.5685871103211));
#218972=CARTESIAN_POINT('Ctrl Pts',(-56.4325933078519,65.8347384603639,
59.4333716522234));
#218973=CARTESIAN_POINT('Ctrl Pts',(-56.3167128323229,69.8553822533185,
59.906576337004));
#218974=CARTESIAN_POINT('Ctrl Pts',(-56.2008323567939,73.3716056610648,
61.9129841055396));
#218975=CARTESIAN_POINT('Ctrl Pts',(-56.0849518812639,75.8244962363713,
65.1336714529827));
#218976=CARTESIAN_POINT('Ctrl Pts',(-55.9690714057349,76.8241609272865,
69.0567021408465));
#218977=CARTESIAN_POINT('Ctrl Pts',(-55.8531909302059,76.2117005487124,
73.058500627591));
#218978=CARTESIAN_POINT('Ctrl Pts',(-55.7373104546769,74.0844671944947,
76.502971347812));
#218979=CARTESIAN_POINT('Ctrl Pts',(-55.6214299791479,70.7805899107851,
78.8426061994355));
#218980=CARTESIAN_POINT('Ctrl Pts',(-55.5055495036199,66.8252281299281,
79.705517853136));
#218981=CARTESIAN_POINT('Ctrl Pts',(-55.3896690280909,62.8470966996323,
78.9545315059017));
#218982=CARTESIAN_POINT('Ctrl Pts',(-55.2737885525619,59.4785285066753,
76.7090662664087));
#218983=CARTESIAN_POINT('Ctrl Pts',(-55.1579080770329,57.2549695240061,
73.3258654140387));
#218984=CARTESIAN_POINT('Ctrl Pts',(-55.0806544266799,56.7715539811408,
70.6708652489211));
#218985=CARTESIAN_POINT('Ctrl Pts',(-55.0420276015039,56.7988040763871,
69.3485711280681));
#218986=CARTESIAN_POINT('Ctrl Pts',(-62.2342499251029,57.8065696683908,
74.8099293892527));
#218987=CARTESIAN_POINT('Ctrl Pts',(-62.1956230999259,57.1031312732521,
73.6224666938169));
#218988=CARTESIAN_POINT('Ctrl Pts',(-62.1183694495739,56.1796658359588,
70.9619911069131));
#218989=CARTESIAN_POINT('Ctrl Pts',(-62.0024889740439,56.4635561166055,
66.7467220222677));
#218990=CARTESIAN_POINT('Ctrl Pts',(-61.8866084985149,58.3717651523206,
62.9775246456951));
#218991=CARTESIAN_POINT('Ctrl Pts',(-61.7707280229859,61.6008831507443,
60.2533615179501));
#218992=CARTESIAN_POINT('Ctrl Pts',(-61.6548475474569,65.6376592981465,
59.007288209015));
#218993=CARTESIAN_POINT('Ctrl Pts',(-61.5389670719279,69.8404311589655,
59.4373596262818));
#218994=CARTESIAN_POINT('Ctrl Pts',(-61.4230865963979,73.5411595353312,
61.4752179418165));
#218995=CARTESIAN_POINT('Ctrl Pts',(-61.3072061208689,76.1516039658375,
64.7969396843518));
#218996=CARTESIAN_POINT('Ctrl Pts',(-61.1913256453399,77.2568279536785,
68.8745291515198));
#218997=CARTESIAN_POINT('Ctrl Pts',(-61.0754451698099,76.6811533646194,
73.0598433065362));
#218998=CARTESIAN_POINT('Ctrl Pts',(-60.9595646942809,74.5160851144003,
76.6876160812524));
#218999=CARTESIAN_POINT('Ctrl Pts',(-60.8436842187519,71.1057661783553,
79.1812039750165));
#219000=CARTESIAN_POINT('Ctrl Pts',(-60.7278037432219,66.9922752255877,
80.1442449974989));
#219001=CARTESIAN_POINT('Ctrl Pts',(-60.6119232676929,62.8294618635471,
79.4236613850277));
#219002=CARTESIAN_POINT('Ctrl Pts',(-60.4960427921629,59.2790156194285,
77.1339916933007));
#219003=CARTESIAN_POINT('Ctrl Pts',(-60.3801623166339,56.9052887454224,
73.6391846088869));
#219004=CARTESIAN_POINT('Ctrl Pts',(-60.2642818411039,56.0855910260969,
69.4947484013197));
#219005=CARTESIAN_POINT('Ctrl Pts',(-60.1484013655749,56.9502154506322,
65.3594515033776));
#219006=CARTESIAN_POINT('Ctrl Pts',(-60.0325208900459,59.361727818425,61.8906096318565));
#219007=CARTESIAN_POINT('Ctrl Pts',(-59.9166404145159,62.9368122467912,
59.6396038211846));
#219008=CARTESIAN_POINT('Ctrl Pts',(-59.8007599389869,67.1072001829157,
58.9642370379884));
#219009=CARTESIAN_POINT('Ctrl Pts',(-59.6848794634569,71.209998102294,59.9718605105236));
#219010=CARTESIAN_POINT('Ctrl Pts',(-59.5689989879279,74.5930560815087,
62.5023099842152));
#219011=CARTESIAN_POINT('Ctrl Pts',(-59.4531185123979,76.7186286489653,
66.1533642278691));
#219012=CARTESIAN_POINT('Ctrl Pts',(-59.3372380368689,77.2488507637066,
70.3446790977719));
#219013=CARTESIAN_POINT('Ctrl Pts',(-59.2213575613389,76.0994423031657,
74.4100346812925));
#219014=CARTESIAN_POINT('Ctrl Pts',(-59.1054770858099,73.4531045980525,
77.7032326073399));
#219015=CARTESIAN_POINT('Ctrl Pts',(-58.9895966102799,69.7304796018871,
79.7008108830386));
#219016=CARTESIAN_POINT('Ctrl Pts',(-58.8737161347509,65.5232878073241,
80.0852494781353));
#219017=CARTESIAN_POINT('Ctrl Pts',(-58.7578356592209,61.5002728036194,
78.7954409227264));
#219018=CARTESIAN_POINT('Ctrl Pts',(-58.6419551836919,58.3009028215076,
76.0364034914597));
#219019=CARTESIAN_POINT('Ctrl Pts',(-58.5260747081619,56.433725669026,72.2466930393406));
#219020=CARTESIAN_POINT('Ctrl Pts',(-58.4101942326329,56.1955337939067,
68.0286934589439));
#219021=CARTESIAN_POINT('Ctrl Pts',(-58.2943137571039,57.624188386514,64.0528662639259));
#219022=CARTESIAN_POINT('Ctrl Pts',(-58.1784332815739,60.4926012496316,
60.9511790655875));
#219023=CARTESIAN_POINT('Ctrl Pts',(-58.0625528060449,64.3448310315735,
59.2166527507834));
#219024=CARTESIAN_POINT('Ctrl Pts',(-57.9466723305149,68.5685562369575,
59.1249945869912));
#219025=CARTESIAN_POINT('Ctrl Pts',(-57.8307918549859,72.4924052498076,
60.690773867081));
#219026=CARTESIAN_POINT('Ctrl Pts',(-57.7149113794559,75.4926725200354,
63.6651060840354));
#219027=CARTESIAN_POINT('Ctrl Pts',(-57.5990309039269,77.0924581103469,
67.575213741715));
#219028=CARTESIAN_POINT('Ctrl Pts',(-57.4831504283979,77.0374721262134,
71.7995755125809));
#219029=CARTESIAN_POINT('Ctrl Pts',(-57.3672699528679,75.3364547264357,
75.6667185969866));
#219030=CARTESIAN_POINT('Ctrl Pts',(-57.2513894773389,72.2597868531839,
78.5619509930676));
#219031=CARTESIAN_POINT('Ctrl Pts',(-57.1355090018099,68.2965125094352,
80.0250683177526));
#219032=CARTESIAN_POINT('Ctrl Pts',(-57.0196285262799,64.076603999578,79.8235044369148));
#219033=CARTESIAN_POINT('Ctrl Pts',(-56.9037480507509,60.2708262663669,
77.9892984302229));
#219034=CARTESIAN_POINT('Ctrl Pts',(-56.7878675752219,57.4841171366094,
74.8140018998644));
#219035=CARTESIAN_POINT('Ctrl Pts',(-56.6719870996929,56.1594309505505,
70.8023361189085));
#219036=CARTESIAN_POINT('Ctrl Pts',(-56.5561066241629,56.5073298688805,
66.5919653309315));
#219037=CARTESIAN_POINT('Ctrl Pts',(-56.4402261486339,58.4725144941193,
62.8521384340947));
#219038=CARTESIAN_POINT('Ctrl Pts',(-56.3243456731049,61.7426138472405,
60.1773102058845));
#219039=CARTESIAN_POINT('Ctrl Pts',(-56.2084651975759,65.7978375109195,
58.992651239347));
#219040=CARTESIAN_POINT('Ctrl Pts',(-56.0925847220469,69.9935976079059,
59.4864660203555));
#219041=CARTESIAN_POINT('Ctrl Pts',(-55.9767042465179,73.6629676456614,
61.5802614638165));
#219042=CARTESIAN_POINT('Ctrl Pts',(-55.8608237709879,76.2226921395821,
64.941223576645));
#219043=CARTESIAN_POINT('Ctrl Pts',(-55.7449432954589,77.2658965208973,
69.0351190986164));
#219044=CARTESIAN_POINT('Ctrl Pts',(-55.6290628199299,76.6267608625964,
73.2112130953809));
#219045=CARTESIAN_POINT('Ctrl Pts',(-55.5131823444009,74.4068773602934,
76.8057053079185));
#219046=CARTESIAN_POINT('Ctrl Pts',(-55.3973018688719,70.9591020322142,
79.2472413050085));
#219047=CARTESIAN_POINT('Ctrl Pts',(-55.2814213933429,66.8314672593026,
80.1477364670454));
#219048=CARTESIAN_POINT('Ctrl Pts',(-55.1655409178149,62.6800711209345,
79.3640414392399));
#219049=CARTESIAN_POINT('Ctrl Pts',(-55.0496604422859,59.1647873166941,
77.0207765453072));
#219050=CARTESIAN_POINT('Ctrl Pts',(-54.9337799667569,56.844382791141,73.4902227664913));
#219051=CARTESIAN_POINT('Ctrl Pts',(-54.8565263164039,56.3399124253312,
70.7195859421522));
#219052=CARTESIAN_POINT('Ctrl Pts',(-54.8178994912279,56.3683493792519,
69.3397002336784));
#219053=CARTESIAN_POINT('',(-62.7285891236391,57.5976540486463,69.9231276410268));
#219054=CARTESIAN_POINT('Ctrl Pts',(-65.2384132905482,57.4206397706274,
65.0087087433499));
#219055=CARTESIAN_POINT('Ctrl Pts',(-65.2029278919597,57.979092375435,63.8703843309197));
#219056=CARTESIAN_POINT('Ctrl Pts',(-65.1319570947826,59.5203119770194,
61.8024113142919));
#219057=CARTESIAN_POINT('Ctrl Pts',(-65.0255008990171,62.7950529612741,
59.7419494328987));
#219058=CARTESIAN_POINT('Ctrl Pts',(-64.9190447032515,66.5922763045987,
59.0003860876846));
#219059=CARTESIAN_POINT('Ctrl Pts',(-64.8125885074859,70.4015698547972,
59.6773007910861));
#219060=CARTESIAN_POINT('Ctrl Pts',(-64.7061323117203,73.7108304890285,
61.6817243939746));
#219061=CARTESIAN_POINT('Ctrl Pts',(-64.5996761159548,76.0751935268562,
64.7441915297997));
#219062=CARTESIAN_POINT('Ctrl Pts',(-64.4932199201892,77.1768132902845,
68.4530125546886));
#219063=CARTESIAN_POINT('Ctrl Pts',(-64.3867637244237,76.8675977656186,
72.3096048992952));
#219064=CARTESIAN_POINT('Ctrl Pts',(-64.2803075286581,75.1891151585901,
75.7955215493427));
#219065=CARTESIAN_POINT('Ctrl Pts',(-64.1738513328926,72.367006249171,78.4421459656916));
#219066=CARTESIAN_POINT('Ctrl Pts',(-64.0673951371271,68.7806511388025,
79.8936880956339));
#219067=CARTESIAN_POINT('Ctrl Pts',(-63.9609389413616,64.9121684082349,
79.9550174392734));
#219068=CARTESIAN_POINT('Ctrl Pts',(-63.8544827455961,61.2816042571687,
78.6178806428873));
#219069=CARTESIAN_POINT('Ctrl Pts',(-63.7480265498306,58.3770181385261,
76.0620635928089));
#219070=CARTESIAN_POINT('Ctrl Pts',(-63.6415703540651,56.58888652557,72.6310262841577));
#219071=CARTESIAN_POINT('Ctrl Pts',(-63.5705995568881,56.3013337084174,
70.0679844126329));
#219072=CARTESIAN_POINT('Ctrl Pts',(-63.5351141582999,56.3933756893344,
68.8033975024123));
#219073=CARTESIAN_POINT('Ctrl Pts',(-65.0142851802722,57.8071755591803,
65.1983400256205));
#219074=CARTESIAN_POINT('Ctrl Pts',(-64.9787997816837,58.3423203118127,
64.1075252799264));
#219075=CARTESIAN_POINT('Ctrl Pts',(-64.9078289845066,59.8192148151818,
62.1258622007476));
#219076=CARTESIAN_POINT('Ctrl Pts',(-64.801372788741,62.9572796014205,60.1513967683752));
#219077=CARTESIAN_POINT('Ctrl Pts',(-64.6949165929754,66.5960201663911,
59.4407836751364));
#219078=CARTESIAN_POINT('Ctrl Pts',(-64.5884603972099,70.2463271701436,
60.0894463340285));
#219079=CARTESIAN_POINT('Ctrl Pts',(-64.4820042014443,73.4174708772949,
62.0102123290094));
#219080=CARTESIAN_POINT('Ctrl Pts',(-64.3755480056787,75.6831536981848,
64.9448628324088));
#219081=CARTESIAN_POINT('Ctrl Pts',(-64.2690918099132,76.738795718137,68.4988906815205));
#219082=CARTESIAN_POINT('Ctrl Pts',(-64.1626356141476,76.4424857644709,
72.1945223939759));
#219083=CARTESIAN_POINT('Ctrl Pts',(-64.0561794183821,74.8340571318683,
75.5349491147065));
#219084=CARTESIAN_POINT('Ctrl Pts',(-63.9497232226166,72.1297331458918,
78.0711127145999));
#219085=CARTESIAN_POINT('Ctrl Pts',(-63.843267026851,68.693059913747,79.4620725693219));
#219086=CARTESIAN_POINT('Ctrl Pts',(-63.7368108310855,64.986034078319,79.5208422413553));
#219087=CARTESIAN_POINT('Ctrl Pts',(-63.63035463532,61.5069969357081,78.2395128430028));
#219088=CARTESIAN_POINT('Ctrl Pts',(-63.5238984395549,58.7236380498246,
75.7903666285429));
#219089=CARTESIAN_POINT('Ctrl Pts',(-63.4174422437889,57.010136776047,72.5025287780578));
#219090=CARTESIAN_POINT('Ctrl Pts',(-63.3464714466119,56.7345854045009,
70.0464592808521));
#219091=CARTESIAN_POINT('Ctrl Pts',(-63.3109860480239,56.8227858761024,
68.8346517909851));
#219092=CARTESIAN_POINT('Ctrl Pts',(-64.7901570699962,58.1937113477375,
65.3879713079069));
#219093=CARTESIAN_POINT('Ctrl Pts',(-64.7546716714076,58.7055482481762,
64.3446662289412));
#219094=CARTESIAN_POINT('Ctrl Pts',(-64.6837008742306,60.1181176533299,
62.4493130872116));
#219095=CARTESIAN_POINT('Ctrl Pts',(-64.577244678465,63.1195062415454,60.5608441038514));
#219096=CARTESIAN_POINT('Ctrl Pts',(-64.4707884826994,66.5997640281635,
59.8811812625842));
#219097=CARTESIAN_POINT('Ctrl Pts',(-64.3643322869338,70.0910844854805,
60.5015918769625));
#219098=CARTESIAN_POINT('Ctrl Pts',(-64.2578760911682,73.1241112655526,
62.3387002640363));
#219099=CARTESIAN_POINT('Ctrl Pts',(-64.1514198954027,75.2911138695092,
65.1455341350098));
#219100=CARTESIAN_POINT('Ctrl Pts',(-64.0449636996371,76.3007781459888,
68.5447688083423));
#219101=CARTESIAN_POINT('Ctrl Pts',(-63.9385075038716,76.0173737633253,
72.0794398886478));
#219102=CARTESIAN_POINT('Ctrl Pts',(-63.832051308106,74.4789991051512,75.2743766800647));
#219103=CARTESIAN_POINT('Ctrl Pts',(-63.7255951123405,71.8924600426187,
77.7000794635043));
#219104=CARTESIAN_POINT('Ctrl Pts',(-63.619138916575,68.6054686886978,79.0304570430104));
#219105=CARTESIAN_POINT('Ctrl Pts',(-63.5126827208099,65.0598997484077,
79.0866670434391));
#219106=CARTESIAN_POINT('Ctrl Pts',(-63.4062265250439,61.7323896142594,
77.8611450431157));
#219107=CARTESIAN_POINT('Ctrl Pts',(-63.2997703292789,59.0702579611228,
75.5186696642778));
#219108=CARTESIAN_POINT('Ctrl Pts',(-63.1933141335129,57.4313870265325,
72.3740312719636));
#219109=CARTESIAN_POINT('Ctrl Pts',(-63.1223433363359,57.1678371005937,
70.0249341490751));
#219110=CARTESIAN_POINT('Ctrl Pts',(-63.0868579377479,57.2521960628615,
68.8659060795531));
#219111=CARTESIAN_POINT('Ctrl Pts',(-64.5660289597201,58.5802471362906,
65.5776025901772));
#219112=CARTESIAN_POINT('Ctrl Pts',(-64.5305435611316,59.0687761845539,
64.5818071779478));
#219113=CARTESIAN_POINT('Ctrl Pts',(-64.4595727639545,60.4170204914826,
62.7727639736645));
#219114=CARTESIAN_POINT('Ctrl Pts',(-64.3531165681889,63.2817328816918,
60.9702914393279));
#219115=CARTESIAN_POINT('Ctrl Pts',(-64.2466603724233,66.6035078899466,
60.3215788500322));
#219116=CARTESIAN_POINT('Ctrl Pts',(-64.1402041766578,69.9358418008276,
60.913737419903));
#219117=CARTESIAN_POINT('Ctrl Pts',(-64.0337479808922,72.8307516538193,
62.6671881990702));
#219118=CARTESIAN_POINT('Ctrl Pts',(-63.9272917851266,74.8990740408378,
65.3462054376189));
#219119=CARTESIAN_POINT('Ctrl Pts',(-63.8208355893611,75.8627605738414,
68.5906469351743));
#219120=CARTESIAN_POINT('Ctrl Pts',(-63.7143793935955,75.5922617621774,
71.9643573833286));
#219121=CARTESIAN_POINT('Ctrl Pts',(-63.60792319783,74.1239410784296,75.0138042454287));
#219122=CARTESIAN_POINT('Ctrl Pts',(-63.5014670020649,71.6551869393394,
77.3290462124126));
#219123=CARTESIAN_POINT('Ctrl Pts',(-63.3950108062989,68.5178774636422,
78.5988415166984));
#219124=CARTESIAN_POINT('Ctrl Pts',(-63.2885546105339,65.1337654184909,
78.6524918455206));
#219125=CARTESIAN_POINT('Ctrl Pts',(-63.1820984147679,61.9577822928,77.4827772432284));
#219126=CARTESIAN_POINT('Ctrl Pts',(-63.0756422190029,59.4168778724121,
75.246972700008));
#219127=CARTESIAN_POINT('Ctrl Pts',(-62.9691860232369,57.8526372770187,
72.2455337658675));
#219128=CARTESIAN_POINT('Ctrl Pts',(-62.8982152260599,57.6010887966773,
70.0034090172943));
#219129=CARTESIAN_POINT('Ctrl Pts',(-62.8627298274719,57.6816062496299,
68.897160368125));
#219130=CARTESIAN_POINT('Ctrl Pts',(-64.5675364832709,60.6333197960278,
62.5540045030464));
#219131=CARTESIAN_POINT('Ctrl Pts',(-64.5675364832709,60.316276790239,62.8628731621224));
#219132=CARTESIAN_POINT('Ctrl Pts',(-64.5675364832687,60.0228219393915,
63.1936835736482));
#219133=CARTESIAN_POINT('Ctrl Pts',(-64.5675364832687,59.4938075108645,
63.8842115791695));
#219134=CARTESIAN_POINT('Ctrl Pts',(-64.5675364832709,59.2568109510257,
64.2429885299645));
#219135=CARTESIAN_POINT('Ctrl Pts',(-64.5675364832709,59.0462179431753,
64.6166308207582));
#219136=CARTESIAN_POINT('Ctrl Pts',(-63.5337949169409,56.4405087963681,
69.9703303450313));
#219137=CARTESIAN_POINT('Ctrl Pts',(-63.5394868426676,56.4486993034411,
70.1709662592209));
#219138=CARTESIAN_POINT('Ctrl Pts',(-63.5451666556007,56.462783905414,70.3713185694427));
#219139=CARTESIAN_POINT('Ctrl Pts',(-63.5564167240732,56.5024402153682,
70.7682868434315));
#219140=CARTESIAN_POINT('Ctrl Pts',(-63.5619850785309,56.527848667695,70.9648330212303));
#219141=CARTESIAN_POINT('Ctrl Pts',(-63.5675399484425,56.5589377686512,
71.1605188170944));
#219142=CARTESIAN_POINT('Origin',(-49.5265537491909,65.9734210682048,61.9560808081071));
#219143=CARTESIAN_POINT('',(-47.1840596451126,66.5535285669906,62.195755942179));
#219144=CARTESIAN_POINT('',(-39.7523422906826,68.3939579446667,62.9561411445198));
#219145=CARTESIAN_POINT('',(-47.1840596451109,66.5535285669907,62.1957559421787));
#219146=CARTESIAN_POINT('',(-47.119731784661,69.2594615665078,63.3137295174307));
#219147=CARTESIAN_POINT('Origin',(-113.778845940191,69.2594615665078,63.3137295174307));
#219148=CARTESIAN_POINT('Origin',(-113.778845940191,69.2594615665078,63.3137295174307));
#219149=CARTESIAN_POINT('Origin',(27.1782499005891,77.5774829011345,66.75037338561));
#219150=CARTESIAN_POINT('Origin',(27.1782499005891,75.,72.9888893865801));
#219151=CARTESIAN_POINT('Origin',(27.1782499005891,75.,72.9888893865801));
#219152=CARTESIAN_POINT('',(-39.7523422906826,63.2389921423977,75.4331731464599));
#219153=CARTESIAN_POINT('Origin',(27.1782499005891,72.4225170988655,79.2274053875501));
#219154=CARTESIAN_POINT('Ctrl Pts',(-39.7523422906847,68.3939579446667,
62.9561411445199));
#219155=CARTESIAN_POINT('Ctrl Pts',(-39.7281387736131,67.4261905019625,
63.4318987914185));
#219156=CARTESIAN_POINT('Ctrl Pts',(-39.7067753132048,66.4946705665665,
64.0835294670284));
#219157=CARTESIAN_POINT('Ctrl Pts',(-39.6724659131911,64.7167905326718,
65.8377960430231));
#219158=CARTESIAN_POINT('Ctrl Pts',(-39.6628533608352,63.9426641268814,
67.0147663024293));
#219159=CARTESIAN_POINT('Ctrl Pts',(-39.6628533608352,62.9504704429495,
69.4162628052949));
#219160=CARTESIAN_POINT('Ctrl Pts',(-39.6724659131911,62.6681079916684,
70.7964084967982));
#219161=CARTESIAN_POINT('Ctrl Pts',(-39.7067753132048,62.6893142216513,
73.2939791024836));
#219162=CARTESIAN_POINT('Ctrl Pts',(-39.7281387736131,62.8892464901659,
74.4130765135442));
#219163=CARTESIAN_POINT('Ctrl Pts',(-39.7523422906848,63.2389921423979,
75.4331731464598));
#219164=CARTESIAN_POINT('Origin',(-23.4378585958609,75.,72.9888893865801));
#219165=CARTESIAN_POINT('Ctrl Pts',(-23.3090332587941,86.7759771267022,
77.8543002128612));
#219166=CARTESIAN_POINT('Ctrl Pts',(-23.3534781005806,87.1687858104401,
77.0199591890651));
#219167=CARTESIAN_POINT('Ctrl Pts',(-23.3969857639789,87.4684685784188,
76.1481661238117));
#219168=CARTESIAN_POINT('Ctrl Pts',(-23.4821035727886,87.8768797291089,
74.3427299956353));
#219169=CARTESIAN_POINT('Ctrl Pts',(-23.5241358609362,87.9823712605097,
73.4125249276302));
#219170=CARTESIAN_POINT('Ctrl Pts',(-23.5675316904177,87.9904527821819,
72.490756361305));
#219171=CARTESIAN_POINT('Ctrl Pts',(-38.3758095864366,70.2663422358007,
83.8196273194875));
#219172=CARTESIAN_POINT('Ctrl Pts',(-38.4258466097666,72.1087543535617,
84.7194504420196));
#219173=CARTESIAN_POINT('Ctrl Pts',(-38.525920656419,76.3137202385278,85.5568522331398));
#219174=CARTESIAN_POINT('Ctrl Pts',(-38.6760317264166,82.5445125465804,
83.4636401838068));
#219175=CARTESIAN_POINT('Ctrl Pts',(-38.826142796409,86.9995287031468,78.4421077647583));
#219176=CARTESIAN_POINT('Ctrl Pts',(-38.9262168430666,87.9290806197203,
73.9710084799022));
#219177=CARTESIAN_POINT('Ctrl Pts',(-38.9762538663893,87.7996291647998,
71.7442636422223));
#219178=CARTESIAN_POINT('Ctrl Pts',(-38.4975359461084,70.2663422358007,
83.8196273194875));
#219179=CARTESIAN_POINT('Ctrl Pts',(-38.5475729694384,72.1087543535617,
84.7194504420196));
#219180=CARTESIAN_POINT('Ctrl Pts',(-38.647647016096,76.3137202385278,85.5568522331398));
#219181=CARTESIAN_POINT('Ctrl Pts',(-38.7977580860884,82.5445125465804,
83.4636401838068));
#219182=CARTESIAN_POINT('Ctrl Pts',(-38.947869156086,86.9995287031468,78.4421077647583));
#219183=CARTESIAN_POINT('Ctrl Pts',(-39.0479432027384,87.9290806197203,
73.9710084799022));
#219184=CARTESIAN_POINT('Ctrl Pts',(-39.0979802260676,87.7996291647998,
71.7442636422223));
#219185=CARTESIAN_POINT('Ctrl Pts',(-38.6192623057863,70.2663422358007,
83.8196273194875));
#219186=CARTESIAN_POINT('Ctrl Pts',(-38.6692993291154,72.1087543535617,
84.7194504420196));
#219187=CARTESIAN_POINT('Ctrl Pts',(-38.7693733757677,76.3137202385278,
85.5568522331398));
#219188=CARTESIAN_POINT('Ctrl Pts',(-38.9194844457654,82.5445125465804,
83.4636401838068));
#219189=CARTESIAN_POINT('Ctrl Pts',(-39.0695955157577,86.9995287031468,
78.4421077647583));
#219190=CARTESIAN_POINT('Ctrl Pts',(-39.1696695624154,87.9290806197203,
73.9710084799022));
#219191=CARTESIAN_POINT('Ctrl Pts',(-39.2197065857454,87.7996291647998,
71.7442636422223));
#219192=CARTESIAN_POINT('Ctrl Pts',(-38.7409886654647,70.2663422358007,
83.8196273194875));
#219193=CARTESIAN_POINT('Ctrl Pts',(-38.7910256887871,72.1087543535617,
84.7194504420196));
#219194=CARTESIAN_POINT('Ctrl Pts',(-38.8910997354449,76.3137202385278,
85.5568522331398));
#219195=CARTESIAN_POINT('Ctrl Pts',(-39.0412108054371,82.5445125465804,
83.4636401838068));
#219196=CARTESIAN_POINT('Ctrl Pts',(-39.1913218754349,86.9995287031468,
78.4421077647583));
#219197=CARTESIAN_POINT('Ctrl Pts',(-39.2913959220871,87.9290806197203,
73.9710084799022));
#219198=CARTESIAN_POINT('Ctrl Pts',(-39.341432945417,87.7996291647998,71.7442636422223));
#219199=CARTESIAN_POINT('',(-38.9948861699879,87.8189932010941,72.2582005417311));
#219200=CARTESIAN_POINT('Ctrl Pts',(-38.4175364832709,70.6959992820295,
84.0186998247411));
#219201=CARTESIAN_POINT('Ctrl Pts',(-38.4515840088496,71.9757680822536,
84.5802970070803));
#219202=CARTESIAN_POINT('Ctrl Pts',(-38.485631534427,73.3662634949739,84.9164019237388));
#219203=CARTESIAN_POINT('Ctrl Pts',(-38.5196790600051,74.7814936945516,
85.0027014194011));
#219204=CARTESIAN_POINT('Ctrl Pts',(-38.5318196218692,75.2861321226979,
85.0334738279137));
#219205=CARTESIAN_POINT('Ctrl Pts',(-38.5439601837334,75.7939152826462,
85.0324846378943));
#219206=CARTESIAN_POINT('Ctrl Pts',(-38.5561007455978,76.3009441519617,
84.9986331104709));
#219207=CARTESIAN_POINT('Ctrl Pts',(-38.6061377689272,78.3906510078787,
84.8591148833621));
#219208=CARTESIAN_POINT('Ctrl Pts',(-38.6561747922594,80.4675817772296,
84.1613775335845));
#219209=CARTESIAN_POINT('Ctrl Pts',(-38.7062118155911,82.2485498546661,
82.9755867888542));
#219210=CARTESIAN_POINT('Ctrl Pts',(-38.7562488389227,84.0295179321026,
81.7897960441239));
#219211=CARTESIAN_POINT('Ctrl Pts',(-38.8062858622539,85.5145233176247,
80.1159519044411));
#219212=CARTESIAN_POINT('Ctrl Pts',(-38.8563228855836,86.4894139895291,
78.1612550133857));
#219213=CARTESIAN_POINT('Ctrl Pts',(-38.8900113257555,87.1457788947348,
76.845215711156));
#219214=CARTESIAN_POINT('Ctrl Pts',(-38.9236997659267,87.570915960302,75.4018511422798));
#219215=CARTESIAN_POINT('Ctrl Pts',(-38.9573884812308,87.7391459645685,
73.9195978901167));
#219216=CARTESIAN_POINT('Ctrl Pts',(-38.9698878032681,87.8015633343225,
73.3696463537504));
#219217=CARTESIAN_POINT('Ctrl Pts',(-38.9823871631799,87.8286156719632,
72.8143415954056));
#219218=CARTESIAN_POINT('Ctrl Pts',(-38.9948865750186,87.8189932821606,
72.2582005494317));
#219219=CARTESIAN_POINT('',(-39.2948856689521,87.8189932822379,72.2582005309434));
#219220=CARTESIAN_POINT('',(-38.9948867524609,87.8189932818422,72.2582005310306));
#219221=CARTESIAN_POINT('Ctrl Pts',(-38.7175257490599,70.6956032368047,
84.0185260206293));
#219222=CARTESIAN_POINT('Ctrl Pts',(-38.7475365958835,71.8236405759,84.5135891741795));
#219223=CARTESIAN_POINT('Ctrl Pts',(-38.7773577336901,73.0301799739484,
84.8302771319025));
#219224=CARTESIAN_POINT('Ctrl Pts',(-38.8371612694423,75.5028698793187,
85.0901078006421));
#219225=CARTESIAN_POINT('Ctrl Pts',(-38.8666805284219,76.7508376105969,
85.0253215589555));
#219226=CARTESIAN_POINT('Ctrl Pts',(-38.9333423802022,79.4983315491103,
84.4457335806272));
#219227=CARTESIAN_POINT('Ctrl Pts',(-38.9699089016275,80.9564254020816,
83.8358955289175));
#219228=CARTESIAN_POINT('Ctrl Pts',(-39.0430464798089,83.5596149995887,
82.1026671558932));
#219229=CARTESIAN_POINT('Ctrl Pts',(-39.0796009224147,84.699796910122,80.9726262266061));
#219230=CARTESIAN_POINT('Ctrl Pts',(-39.1461000544408,86.3398863956807,
78.5958132558447));
#219231=CARTESIAN_POINT('Ctrl Pts',(-39.1756663161435,86.9033056696874,
77.4163792493373));
#219232=CARTESIAN_POINT('Ctrl Pts',(-39.2353970967561,87.6582007704773,
74.9007486757214));
#219233=CARTESIAN_POINT('Ctrl Pts',(-39.2652280895187,87.8418252096164,
73.5778073419934));
#219234=CARTESIAN_POINT('Ctrl Pts',(-39.2948856682995,87.8189932818405,
72.2582005309356));
#219235=CARTESIAN_POINT('Ctrl Pts',(-22.1107451997509,74.4260959710669,
84.8149721769878));
#219236=CARTESIAN_POINT('Ctrl Pts',(-22.1554803513709,76.2585471560719,
84.9038985896115));
#219237=CARTESIAN_POINT('Ctrl Pts',(-22.2449506545909,79.9638470256126,
84.2144079552725));
#219238=CARTESIAN_POINT('Ctrl Pts',(-22.3791561094309,84.4696679742973,
80.7979303917429));
#219239=CARTESIAN_POINT('Ctrl Pts',(-22.5133615642709,86.965463317583,75.7241832750654));
#219240=CARTESIAN_POINT('Ctrl Pts',(-22.6475670191109,86.9220147677009,
70.0699504067063));
#219241=CARTESIAN_POINT('Ctrl Pts',(-22.7817724739509,84.3484238108847,
65.0351802123128));
#219242=CARTESIAN_POINT('Ctrl Pts',(-22.9159779287909,79.7908957547364,
61.6883646725776));
#219243=CARTESIAN_POINT('Ctrl Pts',(-23.0501833836309,74.2166310497644,
60.7397722098012));
#219244=CARTESIAN_POINT('Ctrl Pts',(-23.1843888384709,68.8086151774565,
62.3907153943344));
#219245=CARTESIAN_POINT('Ctrl Pts',(-23.3185942933109,64.7145490031636,
66.2908272630259));
#219246=CARTESIAN_POINT('Ctrl Pts',(-23.4527997481509,62.8032847658051,
71.6124171753859));
#219247=CARTESIAN_POINT('Ctrl Pts',(-23.5870052029909,63.4804352829581,
77.226125163765));
#219248=CARTESIAN_POINT('Ctrl Pts',(-23.7212106578309,66.6022941371127,
81.9405972979455));
#219249=CARTESIAN_POINT('Ctrl Pts',(-23.8554161126709,71.5063333088617,
84.7553175337843));
#219250=CARTESIAN_POINT('Ctrl Pts',(-23.9896215675109,77.1518064053908,
85.0729395141451));
#219251=CARTESIAN_POINT('Ctrl Pts',(-24.1238270223509,82.3406182318677,
82.8260567769257));
#219252=CARTESIAN_POINT('Ctrl Pts',(-24.2580324771909,85.9715872915008,
78.4915079084072));
#219253=CARTESIAN_POINT('Ctrl Pts',(-24.3922379320309,87.2741410374378,
72.9891807694126));
#219254=CARTESIAN_POINT('Ctrl Pts',(-24.5264433868709,85.9718485387383,
67.4867917924943));
#219255=CARTESIAN_POINT('Ctrl Pts',(-24.6606488417109,82.3410852838296,
63.1520705335424));
#219256=CARTESIAN_POINT('Ctrl Pts',(-24.7948542965509,77.1523801433417,
60.9049414386413));
#219257=CARTESIAN_POINT('Ctrl Pts',(-24.9290597513909,71.5068919724511,
61.2222953760158));
#219258=CARTESIAN_POINT('Ctrl Pts',(-25.0632652062309,66.6027191668866,
64.0367827707004));
#219259=CARTESIAN_POINT('Ctrl Pts',(-25.1974706610709,63.4806364728584,
68.7511066704762));
#219260=CARTESIAN_POINT('Ctrl Pts',(-25.3316761159109,62.8032194385157,
74.3647825240852));
#219261=CARTESIAN_POINT('Ctrl Pts',(-25.4658815707509,64.7142309491779,
79.6864630932149));
#219262=CARTESIAN_POINT('Ctrl Pts',(-25.6000870255909,68.8081121689346,
83.586769647843));
#219263=CARTESIAN_POINT('Ctrl Pts',(-25.7342924804309,74.2160488136893,
85.2379684505082));
#219264=CARTESIAN_POINT('Ctrl Pts',(-25.8684979352709,79.7903616710785,
84.2896449343191));
#219265=CARTESIAN_POINT('Ctrl Pts',(-26.0027033901109,84.3480369807344,
80.9430297969229));
#219266=CARTESIAN_POINT('Ctrl Pts',(-26.1369088449509,86.9219104419729,
75.9084414716367));
#219267=CARTESIAN_POINT('Ctrl Pts',(-26.2711142997909,86.9654652521441,
70.2539879752974));
#219268=CARTESIAN_POINT('Ctrl Pts',(-26.3605846030209,85.3021658434783,
66.8719649808209));
#219269=CARTESIAN_POINT('Ctrl Pts',(-26.4053197546309,84.1350213486955,
65.456493688071));
#219270=CARTESIAN_POINT('Ctrl Pts',(-22.2602140739609,74.4260959710669,
84.8149721769878));
#219271=CARTESIAN_POINT('Ctrl Pts',(-22.3049492255709,76.2585471560719,
84.9038985896115));
#219272=CARTESIAN_POINT('Ctrl Pts',(-22.3944195288009,79.9638470256126,
84.2144079552725));
#219273=CARTESIAN_POINT('Ctrl Pts',(-22.5286249836409,84.4696679742973,
80.7979303917429));
#219274=CARTESIAN_POINT('Ctrl Pts',(-22.6628304384809,86.965463317583,75.7241832750654));
#219275=CARTESIAN_POINT('Ctrl Pts',(-22.7970358933209,86.9220147677009,
70.0699504067063));
#219276=CARTESIAN_POINT('Ctrl Pts',(-22.9312413481609,84.3484238108847,
65.0351802123128));
#219277=CARTESIAN_POINT('Ctrl Pts',(-23.0654468030009,79.7908957547364,
61.6883646725776));
#219278=CARTESIAN_POINT('Ctrl Pts',(-23.1996522578409,74.2166310497644,
60.7397722098012));
#219279=CARTESIAN_POINT('Ctrl Pts',(-23.3338577126809,68.8086151774565,
62.3907153943344));
#219280=CARTESIAN_POINT('Ctrl Pts',(-23.4680631675209,64.7145490031636,
66.2908272630259));
#219281=CARTESIAN_POINT('Ctrl Pts',(-23.6022686223609,62.8032847658051,
71.6124171753859));
#219282=CARTESIAN_POINT('Ctrl Pts',(-23.7364740772009,63.4804352829581,
77.226125163765));
#219283=CARTESIAN_POINT('Ctrl Pts',(-23.8706795320409,66.6022941371127,
81.9405972979455));
#219284=CARTESIAN_POINT('Ctrl Pts',(-24.0048849868809,71.5063333088617,
84.7553175337843));
#219285=CARTESIAN_POINT('Ctrl Pts',(-24.1390904417209,77.1518064053908,
85.0729395141451));
#219286=CARTESIAN_POINT('Ctrl Pts',(-24.2732958965609,82.3406182318677,
82.8260567769257));
#219287=CARTESIAN_POINT('Ctrl Pts',(-24.4075013514009,85.9715872915008,
78.4915079084072));
#219288=CARTESIAN_POINT('Ctrl Pts',(-24.5417068062409,87.2741410374378,
72.9891807694126));
#219289=CARTESIAN_POINT('Ctrl Pts',(-24.6759122610809,85.9718485387383,
67.4867917924943));
#219290=CARTESIAN_POINT('Ctrl Pts',(-24.8101177159209,82.3410852838296,
63.1520705335424));
#219291=CARTESIAN_POINT('Ctrl Pts',(-24.9443231707609,77.1523801433417,
60.9049414386413));
#219292=CARTESIAN_POINT('Ctrl Pts',(-25.0785286256009,71.5068919724511,
61.2222953760158));
#219293=CARTESIAN_POINT('Ctrl Pts',(-25.2127340804409,66.6027191668866,
64.0367827707004));
#219294=CARTESIAN_POINT('Ctrl Pts',(-25.3469395352809,63.4806364728584,
68.7511066704762));
#219295=CARTESIAN_POINT('Ctrl Pts',(-25.4811449901209,62.8032194385157,
74.3647825240852));
#219296=CARTESIAN_POINT('Ctrl Pts',(-25.6153504449609,64.7142309491779,
79.6864630932149));
#219297=CARTESIAN_POINT('Ctrl Pts',(-25.7495558998009,68.8081121689346,
83.586769647843));
#219298=CARTESIAN_POINT('Ctrl Pts',(-25.8837613546409,74.2160488136893,
85.2379684505082));
#219299=CARTESIAN_POINT('Ctrl Pts',(-26.0179668094809,79.7903616710785,
84.2896449343191));
#219300=CARTESIAN_POINT('Ctrl Pts',(-26.1521722643209,84.3480369807344,
80.9430297969229));
#219301=CARTESIAN_POINT('Ctrl Pts',(-26.2863777191609,86.9219104419729,
75.9084414716367));
#219302=CARTESIAN_POINT('Ctrl Pts',(-26.4205831740009,86.9654652521441,
70.2539879752974));
#219303=CARTESIAN_POINT('Ctrl Pts',(-26.5100534772209,85.3021658434783,
66.8719649808209));
#219304=CARTESIAN_POINT('Ctrl Pts',(-26.5547886288309,84.1350213486955,
65.456493688071));
#219305=CARTESIAN_POINT('Ctrl Pts',(-22.4096829481609,74.4260959710669,
84.8149721769878));
#219306=CARTESIAN_POINT('Ctrl Pts',(-22.4544180997809,76.2585471560719,
84.9038985896115));
#219307=CARTESIAN_POINT('Ctrl Pts',(-22.5438884030009,79.9638470256126,
84.2144079552725));
#219308=CARTESIAN_POINT('Ctrl Pts',(-22.6780938578409,84.4696679742973,
80.7979303917429));
#219309=CARTESIAN_POINT('Ctrl Pts',(-22.8122993126809,86.965463317583,75.7241832750654));
#219310=CARTESIAN_POINT('Ctrl Pts',(-22.9465047675209,86.9220147677009,
70.0699504067063));
#219311=CARTESIAN_POINT('Ctrl Pts',(-23.0807102223609,84.3484238108847,
65.0351802123128));
#219312=CARTESIAN_POINT('Ctrl Pts',(-23.2149156772009,79.7908957547364,
61.6883646725776));
#219313=CARTESIAN_POINT('Ctrl Pts',(-23.3491211320409,74.2166310497644,
60.7397722098012));
#219314=CARTESIAN_POINT('Ctrl Pts',(-23.4833265868809,68.8086151774565,
62.3907153943344));
#219315=CARTESIAN_POINT('Ctrl Pts',(-23.6175320417209,64.7145490031636,
66.2908272630259));
#219316=CARTESIAN_POINT('Ctrl Pts',(-23.7517374965609,62.8032847658051,
71.6124171753859));
#219317=CARTESIAN_POINT('Ctrl Pts',(-23.8859429514009,63.4804352829581,
77.226125163765));
#219318=CARTESIAN_POINT('Ctrl Pts',(-24.0201484062409,66.6022941371127,
81.9405972979455));
#219319=CARTESIAN_POINT('Ctrl Pts',(-24.1543538610809,71.5063333088617,
84.7553175337843));
#219320=CARTESIAN_POINT('Ctrl Pts',(-24.2885593159209,77.1518064053908,
85.0729395141451));
#219321=CARTESIAN_POINT('Ctrl Pts',(-24.4227647707609,82.3406182318677,
82.8260567769257));
#219322=CARTESIAN_POINT('Ctrl Pts',(-24.5569702256009,85.9715872915008,
78.4915079084072));
#219323=CARTESIAN_POINT('Ctrl Pts',(-24.6911756804409,87.2741410374378,
72.9891807694126));
#219324=CARTESIAN_POINT('Ctrl Pts',(-24.8253811352809,85.9718485387383,
67.4867917924943));
#219325=CARTESIAN_POINT('Ctrl Pts',(-24.9595865901209,82.3410852838296,
63.1520705335424));
#219326=CARTESIAN_POINT('Ctrl Pts',(-25.0937920449609,77.1523801433417,
60.9049414386413));
#219327=CARTESIAN_POINT('Ctrl Pts',(-25.2279974998009,71.5068919724511,
61.2222953760158));
#219328=CARTESIAN_POINT('Ctrl Pts',(-25.3622029546409,66.6027191668866,
64.0367827707004));
#219329=CARTESIAN_POINT('Ctrl Pts',(-25.4964084094809,63.4806364728584,
68.7511066704762));
#219330=CARTESIAN_POINT('Ctrl Pts',(-25.6306138643209,62.8032194385157,
74.3647825240852));
#219331=CARTESIAN_POINT('Ctrl Pts',(-25.7648193191609,64.7142309491779,
79.6864630932149));
#219332=CARTESIAN_POINT('Ctrl Pts',(-25.8990247740009,68.8081121689346,
83.586769647843));
#219333=CARTESIAN_POINT('Ctrl Pts',(-26.0332302288409,74.2160488136893,
85.2379684505082));
#219334=CARTESIAN_POINT('Ctrl Pts',(-26.1674356836809,79.7903616710785,
84.2896449343191));
#219335=CARTESIAN_POINT('Ctrl Pts',(-26.3016411385209,84.3480369807344,
80.9430297969229));
#219336=CARTESIAN_POINT('Ctrl Pts',(-26.4358465933609,86.9219104419729,
75.9084414716367));
#219337=CARTESIAN_POINT('Ctrl Pts',(-26.5700520482009,86.9654652521441,
70.2539879752974));
#219338=CARTESIAN_POINT('Ctrl Pts',(-26.6595223514309,85.3021658434783,
66.8719649808209));
#219339=CARTESIAN_POINT('Ctrl Pts',(-26.7042575030409,84.1350213486955,
65.456493688071));
#219340=CARTESIAN_POINT('Ctrl Pts',(-22.5591518223709,74.4260959710669,
84.8149721769878));
#219341=CARTESIAN_POINT('Ctrl Pts',(-22.6038869739809,76.2585471560719,
84.9038985896115));
#219342=CARTESIAN_POINT('Ctrl Pts',(-22.6933572772109,79.9638470256126,
84.2144079552725));
#219343=CARTESIAN_POINT('Ctrl Pts',(-22.8275627320509,84.4696679742973,
80.7979303917429));
#219344=CARTESIAN_POINT('Ctrl Pts',(-22.9617681868909,86.965463317583,75.7241832750654));
#219345=CARTESIAN_POINT('Ctrl Pts',(-23.0959736417309,86.9220147677009,
70.0699504067063));
#219346=CARTESIAN_POINT('Ctrl Pts',(-23.2301790965709,84.3484238108847,
65.0351802123128));
#219347=CARTESIAN_POINT('Ctrl Pts',(-23.3643845514109,79.7908957547364,
61.6883646725776));
#219348=CARTESIAN_POINT('Ctrl Pts',(-23.4985900062509,74.2166310497644,
60.7397722098012));
#219349=CARTESIAN_POINT('Ctrl Pts',(-23.6327954610909,68.8086151774565,
62.3907153943344));
#219350=CARTESIAN_POINT('Ctrl Pts',(-23.7670009159309,64.7145490031636,
66.2908272630259));
#219351=CARTESIAN_POINT('Ctrl Pts',(-23.9012063707709,62.8032847658051,
71.6124171753859));
#219352=CARTESIAN_POINT('Ctrl Pts',(-24.0354118256109,63.4804352829581,
77.226125163765));
#219353=CARTESIAN_POINT('Ctrl Pts',(-24.1696172804509,66.6022941371127,
81.9405972979455));
#219354=CARTESIAN_POINT('Ctrl Pts',(-24.3038227352909,71.5063333088617,
84.7553175337843));
#219355=CARTESIAN_POINT('Ctrl Pts',(-24.4380281901309,77.1518064053908,
85.0729395141451));
#219356=CARTESIAN_POINT('Ctrl Pts',(-24.5722336449709,82.3406182318677,
82.8260567769257));
#219357=CARTESIAN_POINT('Ctrl Pts',(-24.7064390998109,85.9715872915008,
78.4915079084072));
#219358=CARTESIAN_POINT('Ctrl Pts',(-24.8406445546509,87.2741410374378,
72.9891807694126));
#219359=CARTESIAN_POINT('Ctrl Pts',(-24.9748500094909,85.9718485387383,
67.4867917924943));
#219360=CARTESIAN_POINT('Ctrl Pts',(-25.1090554643309,82.3410852838296,
63.1520705335424));
#219361=CARTESIAN_POINT('Ctrl Pts',(-25.2432609191709,77.1523801433417,
60.9049414386413));
#219362=CARTESIAN_POINT('Ctrl Pts',(-25.3774663740109,71.5068919724511,
61.2222953760158));
#219363=CARTESIAN_POINT('Ctrl Pts',(-25.5116718288509,66.6027191668866,
64.0367827707004));
#219364=CARTESIAN_POINT('Ctrl Pts',(-25.6458772836909,63.4806364728584,
68.7511066704762));
#219365=CARTESIAN_POINT('Ctrl Pts',(-25.7800827385309,62.8032194385157,
74.3647825240852));
#219366=CARTESIAN_POINT('Ctrl Pts',(-25.9142881933709,64.7142309491779,
79.6864630932149));
#219367=CARTESIAN_POINT('Ctrl Pts',(-26.0484936482109,68.8081121689346,
83.586769647843));
#219368=CARTESIAN_POINT('Ctrl Pts',(-26.1826991030509,74.2160488136893,
85.2379684505082));
#219369=CARTESIAN_POINT('Ctrl Pts',(-26.3169045578909,79.7903616710785,
84.2896449343191));
#219370=CARTESIAN_POINT('Ctrl Pts',(-26.4511100127309,84.3480369807344,
80.9430297969229));
#219371=CARTESIAN_POINT('Ctrl Pts',(-26.5853154675709,86.9219104419729,
75.9084414716367));
#219372=CARTESIAN_POINT('Ctrl Pts',(-26.7195209224109,86.9654652521441,
70.2539879752974));
#219373=CARTESIAN_POINT('Ctrl Pts',(-26.8089912256309,85.3021658434783,
66.8719649808209));
#219374=CARTESIAN_POINT('Ctrl Pts',(-26.8537263772509,84.1350213486955,
65.456493688071));
#219375=CARTESIAN_POINT('',(-22.5675364832709,77.7955487498991,84.4927878836045));
#219376=CARTESIAN_POINT('Ctrl Pts',(-22.5675364832709,77.7955487498991,
84.4927878836045));
#219377=CARTESIAN_POINT('Ctrl Pts',(-22.57020057496,77.8986189539504,84.4677938383652));
#219378=CARTESIAN_POINT('Ctrl Pts',(-22.5728694661945,78.0013560923501,
84.441425351644));
#219379=CARTESIAN_POINT('Ctrl Pts',(-22.5892107892951,78.6279360739735,
84.2716538955972));
#219380=CARTESIAN_POINT('Ctrl Pts',(-22.6029000963901,79.1424289701199,
84.0937531125356));
#219381=CARTESIAN_POINT('Ctrl Pts',(-22.6289955619504,80.1303737648569,
83.6729279455323));
#219382=CARTESIAN_POINT('Ctrl Pts',(-22.6413046610228,80.6032904996756,
83.4319232181733));
#219383=CARTESIAN_POINT('Ctrl Pts',(-22.6599801162175,81.2852444850775,
83.0250434517598));
#219384=CARTESIAN_POINT('Ctrl Pts',(-22.6662554006117,81.5084025291211,
82.8815572195231));
#219385=CARTESIAN_POINT('Ctrl Pts',(-22.6893343517265,82.2943804377871,
82.338381580107));
#219386=CARTESIAN_POINT('Ctrl Pts',(-22.7069178418768,82.8283053646328,
81.8966499994326));
#219387=CARTESIAN_POINT('Ctrl Pts',(-22.7321799272807,83.5438776000662,
81.1910813674927));
#219388=CARTESIAN_POINT('Ctrl Pts',(-22.7400417607241,83.7591512188104,
80.9612051460361));
#219389=CARTESIAN_POINT('Ctrl Pts',(-22.7616713766157,84.336272923027,80.2927579212079));
#219390=CARTESIAN_POINT('Ctrl Pts',(-22.7748837672195,84.6748683013689,
79.836706571722));
#219391=CARTESIAN_POINT('Ctrl Pts',(-22.7947609375764,85.1290093994207,
79.1240614113783));
#219392=CARTESIAN_POINT('Ctrl Pts',(-22.8013628413749,85.2707399299882,
78.8833333996349));
#219393=CARTESIAN_POINT('Ctrl Pts',(-22.8237826878272,85.7136353626051,
78.066924838789));
#219394=CARTESIAN_POINT('Ctrl Pts',(-22.8402920915841,85.9768545589435,
77.4705540393854));
#219395=CARTESIAN_POINT('Ctrl Pts',(-22.8648029152498,86.2956042084076,
76.5509224532606));
#219396=CARTESIAN_POINT('Ctrl Pts',(-22.8729157189773,86.3890849049698,
76.240732294204));
#219397=CARTESIAN_POINT('Ctrl Pts',(-22.8959687353953,86.6222757459949,
75.332007597257));
#219398=CARTESIAN_POINT('Ctrl Pts',(-22.9102264149159,86.7271676172055,
74.7270547941961));
#219399=CARTESIAN_POINT('Ctrl Pts',(-22.9311662489936,86.8113873864402,
73.8409316989402));
#219400=CARTESIAN_POINT('Ctrl Pts',(-22.9377614229536,86.8279978971228,
73.5625527580444));
#219401=CARTESIAN_POINT('Ctrl Pts',(-22.9606740565043,86.8513498131262,
72.6142548120919));
#219402=CARTESIAN_POINT('Ctrl Pts',(-22.9777573547803,86.8115150475681,
71.9430921213094));
#219403=CARTESIAN_POINT('Ctrl Pts',(-23.0022394040704,86.671992720847,70.9807639012866));
#219404=CARTESIAN_POINT('Ctrl Pts',(-23.0098099922342,86.6171029656124,
70.6830316311699));
#219405=CARTESIAN_POINT('Ctrl Pts',(-23.0313765416616,86.4242586048633,
69.8254003995603));
#219406=CARTESIAN_POINT('Ctrl Pts',(-23.0447944938455,86.2562544730439,
69.2740313351693));
#219407=CARTESIAN_POINT('Ctrl Pts',(-23.065253732438,85.9431262238287,68.4619538974111));
#219408=CARTESIAN_POINT('Ctrl Pts',(-23.0722491575317,85.8262076718994,
68.1895288569865));
#219409=CARTESIAN_POINT('Ctrl Pts',(-23.0965474361065,85.3945048828662,
67.2786381453861));
#219410=CARTESIAN_POINT('Ctrl Pts',(-23.1147579084652,85.0321561695621,
66.6626023543593));
#219411=CARTESIAN_POINT('Ctrl Pts',(-23.1397715132328,84.4528393429395,
65.8542689058154));
#219412=CARTESIAN_POINT('Ctrl Pts',(-23.1468311929836,84.2798722126102,
65.6303568074651));
#219413=CARTESIAN_POINT('Ctrl Pts',(-23.1676747514248,83.7351091915271,
64.9758232126111));
#219414=CARTESIAN_POINT('Ctrl Pts',(-23.1809179103934,83.3397699452139,
64.5661869646594));
#219415=CARTESIAN_POINT('Ctrl Pts',(-23.2013065948245,82.6947535281514,
63.9868464431381));
#219416=CARTESIAN_POINT('Ctrl Pts',(-23.2083909984642,82.4641120566788,
63.7949330534105));
#219417=CARTESIAN_POINT('Ctrl Pts',(-23.2324629811765,81.6734775488004,
63.1858849928466));
#219418=CARTESIAN_POINT('Ctrl Pts',(-23.2503290955504,81.0829579412128,
62.8082314172617));
#219419=CARTESIAN_POINT('Ctrl Pts',(-23.274884231175,80.2177978658097,62.3572729967872));
#219420=CARTESIAN_POINT('Ctrl Pts',(-23.2818169730839,79.967217664736,62.2376943942904));
#219421=CARTESIAN_POINT('Ctrl Pts',(-23.3035186130702,79.1544845790314,
61.8849216123229));
#219422=CARTESIAN_POINT('Ctrl Pts',(-23.3176588018278,78.5780955922533,
61.6868980638989));
#219423=CARTESIAN_POINT('Ctrl Pts',(-23.3388664824491,77.7066199935249,
61.4600378228033));
#219424=CARTESIAN_POINT('Ctrl Pts',(-23.3458199835038,77.4198619529216,
61.396604555484));
#219425=CARTESIAN_POINT('Ctrl Pts',(-23.3682626536289,76.5069885405669,
61.2296514049591));
#219426=CARTESIAN_POINT('Ctrl Pts',(-23.3844526926338,75.8736638451558,
61.1651917383188));
#219427=CARTESIAN_POINT('Ctrl Pts',(-23.4076843716132,74.9528259617888,
61.1458073048551));
#219428=CARTESIAN_POINT('Ctrl Pts',(-23.4148695247683,74.6661283998542,
61.1502002309265));
#219429=CARTESIAN_POINT('Ctrl Pts',(-23.4372061343355,73.7588131708991,
61.197598239086));
#219430=CARTESIAN_POINT('Ctrl Pts',(-23.4516854993141,73.1415158302191,
61.2799207344635));
#219431=CARTESIAN_POINT('Ctrl Pts',(-23.473533726284,72.2341061026627,61.4737526344134));
#219432=CARTESIAN_POINT('Ctrl Pts',(-23.4808192690093,71.9355685750294,
61.5497313157579));
#219433=CARTESIAN_POINT('Ctrl Pts',(-23.5040385331771,71.014023313647,61.8225462972615));
#219434=CARTESIAN_POINT('Ctrl Pts',(-23.5207281916319,70.4027817691001,
62.0593503041463));
#219435=CARTESIAN_POINT('Ctrl Pts',(-23.5441129061023,69.5685973983824,
62.4648501692936));
#219436=CARTESIAN_POINT('Ctrl Pts',(-23.5509830628036,69.3260891034714,
62.59337145393));
#219437=CARTESIAN_POINT('Ctrl Pts',(-23.5725188546093,68.5661799106487,
63.0311669320326));
#219438=CARTESIAN_POINT('Ctrl Pts',(-23.586588727842,68.0679695342834,63.3723514817946));
#219439=CARTESIAN_POINT('Ctrl Pts',(-23.6083405871129,67.3474767903162,
63.95030372947));
#219440=CARTESIAN_POINT('Ctrl Pts',(-23.6159578353336,67.1044412778182,
64.1620087200796));
#219441=CARTESIAN_POINT('Ctrl Pts',(-23.6398805770154,66.3842235118891,
64.8424376056803));
#219442=CARTESIAN_POINT('Ctrl Pts',(-23.6569839558425,65.9366017169724,
65.3425405823433));
#219443=CARTESIAN_POINT('Ctrl Pts',(-23.6804648193498,65.3762271197312,
66.0871527080676));
#219444=CARTESIAN_POINT('Ctrl Pts',(-23.6870485851372,65.2250152201063,
66.3027475337575));
#219445=CARTESIAN_POINT('Ctrl Pts',(-23.7082031998031,64.753963308414,67.0253571545259));
#219446=CARTESIAN_POINT('Ctrl Pts',(-23.7222219941295,64.4655565082912,
67.5526944759199));
#219447=CARTESIAN_POINT('Ctrl Pts',(-23.7441210530631,64.0823007145137,
68.3991972044232));
#219448=CARTESIAN_POINT('Ctrl Pts',(-23.7519297485862,63.958711695808,68.7054045196297));
#219449=CARTESIAN_POINT('Ctrl Pts',(-23.7755298190367,63.6308976035494,
69.6255567349071));
#219450=CARTESIAN_POINT('Ctrl Pts',(-23.792048790264,63.4632551739869,70.2525895074537));
#219451=CARTESIAN_POINT('Ctrl Pts',(-23.8151391213084,63.3001472115414,
71.153731134077));
#219452=CARTESIAN_POINT('Ctrl Pts',(-23.8218753913198,63.2612963769365,
71.4200932362866));
#219453=CARTESIAN_POINT('Ctrl Pts',(-23.843355585872,63.1650974492894,72.2904016805072));
#219454=CARTESIAN_POINT('Ctrl Pts',(-23.8575579717944,63.145631815119,72.898341634899));
#219455=CARTESIAN_POINT('Ctrl Pts',(-23.8798554463621,63.1873990800895,
73.8427727913731));
#219456=CARTESIAN_POINT('Ctrl Pts',(-23.887881609621,63.216813015148,74.1806799322862));
#219457=CARTESIAN_POINT('Ctrl Pts',(-23.9110847210234,63.3405837357239,
75.1323771410192));
#219458=CARTESIAN_POINT('Ctrl Pts',(-23.9269053581018,63.468623089633,75.7418298181613));
#219459=CARTESIAN_POINT('Ctrl Pts',(-23.9495459158704,63.7217406618819,
76.6026846920868));
#219460=CARTESIAN_POINT('Ctrl Pts',(-23.9564812052755,63.8091170388149,
76.8653374683132));
#219461=CARTESIAN_POINT('Ctrl Pts',(-23.9783573497345,64.1204864991392,
77.7003660271091));
#219462=CARTESIAN_POINT('Ctrl Pts',(-23.9927641337887,64.3807005120457,
78.2589304827354));
#219463=CARTESIAN_POINT('Ctrl Pts',(-24.0155119050265,64.8537349412677,
79.0984245577657));
#219464=CARTESIAN_POINT('Ctrl Pts',(-24.0237891876257,65.0385506994134,
79.3951516670683));
#219465=CARTESIAN_POINT('Ctrl Pts',(-24.0466112890865,65.5718426865505,
80.1732424407906));
#219466=CARTESIAN_POINT('Ctrl Pts',(-24.061713459637,65.9442499022712,80.638247657376));
#219467=CARTESIAN_POINT('Ctrl Pts',(-24.0839137958729,66.5441568990323,
81.2812040167609));
#219468=CARTESIAN_POINT('Ctrl Pts',(-24.0910796733781,66.7465124049511,
81.4828824607709));
#219469=CARTESIAN_POINT('Ctrl Pts',(-24.1140575951936,67.4331012610335,
82.1183964911304));
#219470=CARTESIAN_POINT('Ctrl Pts',(-24.1292856506185,67.9468370336629,
82.5197843027144));
#219471=CARTESIAN_POINT('Ctrl Pts',(-24.1528881185346,68.7808017523536,
83.0682211280822));
#219472=CARTESIAN_POINT('Ctrl Pts',(-24.1611669801198,69.0802693316402,
83.2468935918944));
#219473=CARTESIAN_POINT('Ctrl Pts',(-24.1827559596315,69.8637794574601,
83.6690821495143));
#219474=CARTESIAN_POINT('Ctrl Pts',(-24.1964874148006,70.3580881161013,
83.8935996769948));
#219475=CARTESIAN_POINT('Ctrl Pts',(-24.2174768257465,71.1364599998422,
84.1843685432711));
#219476=CARTESIAN_POINT('Ctrl Pts',(-24.2247571552002,71.4113489338992,
84.2756825250916));
#219477=CARTESIAN_POINT('Ctrl Pts',(-24.2483756982722,72.3324484517258,
84.5438270605486));
#219478=CARTESIAN_POINT('Ctrl Pts',(-24.2640946299929,72.9914513912487,
84.6754742522766));
#219479=CARTESIAN_POINT('Ctrl Pts',(-24.2884926428813,74.0156156886253,
84.7918940226994));
#219480=CARTESIAN_POINT('Ctrl Pts',(-24.2970807599793,74.3762971206503,
84.8163932788444));
#219481=CARTESIAN_POINT('Ctrl Pts',(-24.3182126869123,75.2466209141566,
84.8359863747899));
#219482=CARTESIAN_POINT('Ctrl Pts',(-24.3310868478748,75.7566507505651,
84.8148743652156));
#219483=CARTESIAN_POINT('Ctrl Pts',(-24.3515180034847,76.5608378528089,
84.7292196212533));
#219484=CARTESIAN_POINT('Ctrl Pts',(-24.3590613604394,76.8574867488332,
84.6861535064085));
#219485=CARTESIAN_POINT('Ctrl Pts',(-24.3815384824962,77.7544613305933,
84.5202236828188));
#219486=CARTESIAN_POINT('Ctrl Pts',(-24.3960069964872,78.3477178880852,
84.361341433531));
#219487=CARTESIAN_POINT('Ctrl Pts',(-24.4200877479237,79.3072200064098,
84.0234693101181));
#219488=CARTESIAN_POINT('Ctrl Pts',(-24.4296875364305,79.6823105056442,
83.8695157327653));
#219489=CARTESIAN_POINT('Ctrl Pts',(-24.4517726454238,80.5078291005356,
83.4806056486065));
#219490=CARTESIAN_POINT('Ctrl Pts',(-24.4645281627022,80.9532717977727,
83.2349870119567));
#219491=CARTESIAN_POINT('Ctrl Pts',(-24.4851445577003,81.6411742965046,
82.7956074273199));
#219492=CARTESIAN_POINT('Ctrl Pts',(-24.4929344656444,81.8949348538698,
82.6191436156419));
#219493=CARTESIAN_POINT('Ctrl Pts',(-24.5153697889198,82.619984577831,82.070718348575));
#219494=CARTESIAN_POINT('Ctrl Pts',(-24.5295968633422,83.0704217941672,
81.6718532422128));
#219495=CARTESIAN_POINT('Ctrl Pts',(-24.554091465893,83.7903371793909,80.9304241509068));
#219496=CARTESIAN_POINT('Ctrl Pts',(-24.5643657502694,84.0753692732483,
80.6029215596418));
#219497=CARTESIAN_POINT('Ctrl Pts',(-24.5860905187513,84.6271653904445,
79.8945679247614));
#219498=CARTESIAN_POINT('Ctrl Pts',(-24.5976840511342,84.8912036495773,
79.5115417221267));
#219499=CARTESIAN_POINT('Ctrl Pts',(-24.617262056823,85.293140859179,78.8479458411522));
#219500=CARTESIAN_POINT('Ctrl Pts',(-24.6251367322929,85.4439388309394,
78.5751882904976));
#219501=CARTESIAN_POINT('Ctrl Pts',(-24.6472317420049,85.8435223149737,
77.7784500695001));
#219502=CARTESIAN_POINT('Ctrl Pts',(-24.6610648696817,86.064663119611,77.2407094456923));
#219503=CARTESIAN_POINT('Ctrl Pts',(-24.6908945637501,86.456482279828,76.0472767679595));
#219504=CARTESIAN_POINT('Ctrl Pts',(-24.7068825789411,86.6127117295968,
75.3867366115711));
#219505=CARTESIAN_POINT('Ctrl Pts',(-24.7317749488679,86.7608860128367,
74.3879117013379));
#219506=CARTESIAN_POINT('Ctrl Pts',(-24.7401923448889,86.7959664499832,
74.0559075222126));
#219507=CARTESIAN_POINT('Ctrl Pts',(-24.7610996526957,86.8479953481639,
73.2283760432133));
#219508=CARTESIAN_POINT('Ctrl Pts',(-24.7733789330877,86.8476760342599,
72.7345232328296));
#219509=CARTESIAN_POINT('Ctrl Pts',(-24.7975533204227,86.7836960464734,
71.7369892425435));
#219510=CARTESIAN_POINT('Ctrl Pts',(-24.8094922231537,86.7191369403297,
71.2360827207114));
#219511=CARTESIAN_POINT('Ctrl Pts',(-24.8351973708289,86.5135805647042,
70.1752564221972));
#219512=CARTESIAN_POINT('Ctrl Pts',(-24.8489873208505,86.3628986201724,
69.6171097101358));
#219513=CARTESIAN_POINT('Ctrl Pts',(-24.8715693593638,86.0622123163689,
68.7570415397356));
#219514=CARTESIAN_POINT('Ctrl Pts',(-24.8800360304052,85.9384552655299,
68.4458729535653));
#219515=CARTESIAN_POINT('Ctrl Pts',(-24.9001649362168,85.6112311385889,
67.7156793928889));
#219516=CARTESIAN_POINT('Ctrl Pts',(-24.9116058676399,85.396369265071,67.3042388229351));
#219517=CARTESIAN_POINT('Ctrl Pts',(-24.9367735041841,84.8601517743417,
66.4104777396542));
#219518=CARTESIAN_POINT('Ctrl Pts',(-24.9504401609291,84.5264363613093,
65.9367826121221));
#219519=CARTESIAN_POINT('Ctrl Pts',(-24.9762719223674,83.8412346330971,
65.0999867800875));
#219520=CARTESIAN_POINT('Ctrl Pts',(-24.988409640136,83.4974722462777,64.7304245665329));
#219521=CARTESIAN_POINT('Ctrl Pts',(-25.0096077839032,82.8773660160728,
64.1434312757467));
#219522=CARTESIAN_POINT('Ctrl Pts',(-25.0184772157898,82.6123823701233,
63.913945254008));
#219523=CARTESIAN_POINT('Ctrl Pts',(-25.0395422051444,81.9532506677364,
63.3929967902393));
#219524=CARTESIAN_POINT('Ctrl Pts',(-25.0514814805335,81.5511328915323,
63.1146464292182));
#219525=CARTESIAN_POINT('Ctrl Pts',(-25.0840133009892,80.3941703566912,
62.4152363686961));
#219526=CARTESIAN_POINT('Ctrl Pts',(-25.1043194792746,79.6056888110137,
62.0491341885759));
#219527=CARTESIAN_POINT('Ctrl Pts',(-25.1367303308557,78.3488610258597,
61.6238004627972));
#219528=CARTESIAN_POINT('Ctrl Pts',(-25.1483805833474,77.9017929008133,
61.5009928872115));
#219529=CARTESIAN_POINT('Ctrl Pts',(-25.1736387791005,76.9166702380028,
61.2922240109876));
#219530=CARTESIAN_POINT('Ctrl Pts',(-25.1869032847806,76.3787629153572,
61.2172565919378));
#219531=CARTESIAN_POINT('Ctrl Pts',(-25.2253210748964,74.7863988798278,
61.1055687752883));
#219532=CARTESIAN_POINT('Ctrl Pts',(-25.250090444864,73.7242219547311,61.1721868803465));
#219533=CARTESIAN_POINT('Ctrl Pts',(-25.2866111132704,72.2845467613406,
61.4573505048091));
#219534=CARTESIAN_POINT('Ctrl Pts',(-25.2970871456356,71.8831317764291,
61.5589234989088));
#219535=CARTESIAN_POINT('Ctrl Pts',(-25.3184977186717,71.0566922455767,
61.8158529900833));
#219536=CARTESIAN_POINT('Ctrl Pts',(-25.3294252814237,70.6336872745983,
61.9747898835024));
#219537=CARTESIAN_POINT('Ctrl Pts',(-25.3664389521094,69.224983734498,62.5976549392384));
#219538=CARTESIAN_POINT('Ctrl Pts',(-25.3922393395229,68.2890682628324,
63.1752085088464));
#219539=CARTESIAN_POINT('Ctrl Pts',(-25.4259722928531,67.2491754939645,
64.0348422237022));
#219540=CARTESIAN_POINT('Ctrl Pts',(-25.4325115690716,67.0540968903417,
64.2072922574925));
#219541=CARTESIAN_POINT('Ctrl Pts',(-25.4584055637037,66.2959902400183,
64.9243007064588));
#219542=CARTESIAN_POINT('Ctrl Pts',(-25.4771545578628,65.7814875746081,
65.5197326738897));
#219543=CARTESIAN_POINT('Ctrl Pts',(-25.5148345335165,64.8751005493501,
66.8039004480212));
#219544=CARTESIAN_POINT('Ctrl Pts',(-25.5338126922381,64.4839903217007,
67.493477634905));
#219545=CARTESIAN_POINT('Ctrl Pts',(-25.5649471766414,63.9795411951626,
68.6360369703729));
#219546=CARTESIAN_POINT('Ctrl Pts',(-25.5764187225231,63.8191580945081,
69.0661282181788));
#219547=CARTESIAN_POINT('Ctrl Pts',(-25.603688483182,63.4919624499032,70.1319500539696));
#219548=CARTESIAN_POINT('Ctrl Pts',(-25.6193638008781,63.3521684057306,
70.7735126728818));
#219549=CARTESIAN_POINT('Ctrl Pts',(-25.6676404655836,63.0864418801701,
72.7654883718108));
#219550=CARTESIAN_POINT('Ctrl Pts',(-25.706840999802,63.1059826913564,74.3538296879236));
#219551=CARTESIAN_POINT('Ctrl Pts',(-25.7677255171453,63.7638553875792,
76.7915398688821));
#219552=CARTESIAN_POINT('Ctrl Pts',(-25.7857162873499,64.0285142642929,
77.4989934914382));
#219553=CARTESIAN_POINT('Ctrl Pts',(-25.8216296569917,64.6722868814089,
78.8228079190137));
#219554=CARTESIAN_POINT('Ctrl Pts',(-25.8397202960589,65.0455123990101,
79.4404836250716));
#219555=CARTESIAN_POINT('Ctrl Pts',(-25.8779933757973,65.9757398435127,
80.6982002111685));
#219556=CARTESIAN_POINT('Ctrl Pts',(-25.8981363569753,66.5480633616065,
81.3205005295193));
#219557=CARTESIAN_POINT('Ctrl Pts',(-25.9560699763327,68.3473269415652,
82.9051067066646));
#219558=CARTESIAN_POINT('Ctrl Pts',(-25.9943208487966,69.6965948309391,
83.6873917917103));
#219559=CARTESIAN_POINT('Ctrl Pts',(-26.0504698449138,71.8964316437276,
84.4389540762596));
#219560=CARTESIAN_POINT('Ctrl Pts',(-26.0690068428248,72.6478528993156,
84.6172928635994));
#219561=CARTESIAN_POINT('Ctrl Pts',(-26.0987433017722,73.8478147827651,
84.7809478793954));
#219562=CARTESIAN_POINT('Ctrl Pts',(-26.1097342408935,74.2886635798881,
84.8159239396859));
#219563=CARTESIAN_POINT('Ctrl Pts',(-26.1470592789864,75.8092294267076,
84.8494497159255));
#219564=CARTESIAN_POINT('Ctrl Pts',(-26.1729518813649,76.8897272377984,
84.72474497924));
#219565=CARTESIAN_POINT('Ctrl Pts',(-26.2178106992323,78.6797282706776,
84.2682050190598));
#219566=CARTESIAN_POINT('Ctrl Pts',(-26.2368585546459,79.4076525968821,
84.0054976991742));
#219567=CARTESIAN_POINT('Ctrl Pts',(-26.2902157122182,81.3708528596096,
83.0654858951152));
#219568=CARTESIAN_POINT('Ctrl Pts',(-26.3238790172103,82.5270414745748,
82.2333806609559));
#219569=CARTESIAN_POINT('Ctrl Pts',(-26.3765014687122,84.0251050977193,
80.6895409789442));
#219570=CARTESIAN_POINT('Ctrl Pts',(-26.3948351634072,84.4913388247058,
80.1056895027049));
#219571=CARTESIAN_POINT('Ctrl Pts',(-26.4317390531022,85.3210198323614,
78.8383967304916));
#219572=CARTESIAN_POINT('Ctrl Pts',(-26.4503794465544,85.6797463911431,
78.1542057638403));
#219573=CARTESIAN_POINT('Ctrl Pts',(-26.5123917579555,86.6405138063311,
75.7924075027471));
#219574=CARTESIAN_POINT('Ctrl Pts',(-26.5502886691223,86.8455265760331,
74.2307446510401));
#219575=CARTESIAN_POINT('Ctrl Pts',(-26.6012489913111,86.8339025086032,
72.1366724849289));
#219576=CARTESIAN_POINT('Ctrl Pts',(-26.6203470832269,86.7522129909423,
71.3519615397537));
#219577=CARTESIAN_POINT('Ctrl Pts',(-26.6587218863114,86.4333670988627,
69.8126333019412));
#219578=CARTESIAN_POINT('Ctrl Pts',(-26.6778923634462,86.1958740644985,
69.0608841198639));
#219579=CARTESIAN_POINT('Ctrl Pts',(-26.6970005540986,85.8880596524678,
68.34079083356));
#219580=CARTESIAN_POINT('',(-22.5673849603904,86.330959246387,76.420933693241));
#219581=CARTESIAN_POINT('Ctrl Pts',(-22.5675364832709,86.3312297555765,
76.4210531081684));
#219582=CARTESIAN_POINT('Ctrl Pts',(-22.5675364832709,86.2741961678896,
76.6088225515153));
#219583=CARTESIAN_POINT('Ctrl Pts',(-22.5675364832709,86.2126796921151,
76.7945020356719));
#219584=CARTESIAN_POINT('Ctrl Pts',(-22.5675364832709,86.1467811019396,
76.9781622505484));
#219585=CARTESIAN_POINT('Ctrl Pts',(-22.5675364832709,86.0815911235665,
77.1598475552553));
#219586=CARTESIAN_POINT('Ctrl Pts',(-22.5675364832709,86.0121124400483,
77.3395571455578));
#219587=CARTESIAN_POINT('Ctrl Pts',(-22.5675364832709,85.9383902127073,
77.517347311963));
#219588=CARTESIAN_POINT('Ctrl Pts',(-22.5675364832709,85.8644998030371,
77.6955430706213));
#219589=CARTESIAN_POINT('Ctrl Pts',(-22.5675364832709,85.7863462811828,
77.8718110268535));
#219590=CARTESIAN_POINT('Ctrl Pts',(-22.5675364832709,85.7039258441626,
78.0461899470055));
#219591=CARTESIAN_POINT('Ctrl Pts',(-22.5675364832709,85.6216695539327,
78.220221577807));
#219592=CARTESIAN_POINT('Ctrl Pts',(-22.5675364832709,85.5351631316391,
78.3923720716048));
#219593=CARTESIAN_POINT('Ctrl Pts',(-22.5675364832709,85.444356675763,78.5626563901228));
#219594=CARTESIAN_POINT('Ctrl Pts',(-22.5675364832709,85.3519074893335,
78.7360212302853));
#219595=CARTESIAN_POINT('Ctrl Pts',(-22.5675364832709,85.2550012483283,
78.9074522897057));
#219596=CARTESIAN_POINT('Ctrl Pts',(-22.5675364832709,85.1535389696411,
79.0769339040888));
#219597=CARTESIAN_POINT('Ctrl Pts',(-22.5675364832709,85.1330135891876,
79.1112193021707));
#219598=CARTESIAN_POINT('Ctrl Pts',(-22.5675364832709,85.112301611534,79.1454248056277));
#219599=CARTESIAN_POINT('Ctrl Pts',(-22.5675364832709,85.0914019942509,
79.1795501013667));
#219600=CARTESIAN_POINT('Ctrl Pts',(-22.5675364832709,85.0825999660734,
79.1939222217069));
#219601=CARTESIAN_POINT('Ctrl Pts',(-22.5675364832709,85.0737635427412,
79.2082819117213));
#219602=CARTESIAN_POINT('Ctrl Pts',(-22.5675364832709,85.0648962129969,
79.222623373383));
#219603=CARTESIAN_POINT('Ctrl Pts',(-22.5675364832709,84.9624524331881,
79.3883095024615));
#219604=CARTESIAN_POINT('Ctrl Pts',(-22.5675364832709,84.8563336126465,
79.5508453778107));
#219605=CARTESIAN_POINT('Ctrl Pts',(-22.5675364832709,84.7465736948364,
79.7102890244569));
#219606=CARTESIAN_POINT('Ctrl Pts',(-22.5675364832709,84.6366989413994,
79.8698994880202));
#219607=CARTESIAN_POINT('Ctrl Pts',(-22.5675364832709,84.5231752483645,
80.0264116209949));
#219608=CARTESIAN_POINT('Ctrl Pts',(-22.5675364832709,84.4059903046976,
80.1798598391719));
#219609=CARTESIAN_POINT('Ctrl Pts',(-22.5675364832709,84.317637523426,80.2955536854363));
#219610=CARTESIAN_POINT('Ctrl Pts',(-22.5675364832709,84.2272025167764,
80.4095053825114));
#219611=CARTESIAN_POINT('Ctrl Pts',(-22.5675364832709,84.1346637067308,
80.5217187995516));
#219612=CARTESIAN_POINT('Ctrl Pts',(-22.5675364832709,84.012033104306,80.6704218023783));
#219613=CARTESIAN_POINT('Ctrl Pts',(-22.5675364832709,83.8857092626351,
80.8160736234435));
#219614=CARTESIAN_POINT('Ctrl Pts',(-22.5675364832709,83.7556896189918,
80.9587217968264));
#219615=CARTESIAN_POINT('Ctrl Pts',(-22.5675364832709,83.6254862248831,
81.1015715679642));
#219616=CARTESIAN_POINT('Ctrl Pts',(-22.5675364832709,83.4915762569568,
81.2414094809198));
#219617=CARTESIAN_POINT('Ctrl Pts',(-22.5675364832709,83.3539211456636,
81.3782455399667));
#219618=CARTESIAN_POINT('Ctrl Pts',(-22.5675364832709,83.2896251453197,
81.4421589770841));
#219619=CARTESIAN_POINT('Ctrl Pts',(-22.5675364832709,83.2245116076313,
81.5054169551686));
#219620=CARTESIAN_POINT('Ctrl Pts',(-22.5675364832709,83.1585742143027,
81.5680174025649));
#219621=CARTESIAN_POINT('Ctrl Pts',(-22.5675364832709,83.1405216939231,
81.5851563247355));
#219622=CARTESIAN_POINT('Ctrl Pts',(-22.5675364832709,83.1224029438513,
81.6022500915066));
#219623=CARTESIAN_POINT('Ctrl Pts',(-22.5675364832709,83.1042427730916,
81.6192753723487));
#219624=CARTESIAN_POINT('Ctrl Pts',(-22.5675364832709,82.9650663051577,
81.7497542364821));
#219625=CARTESIAN_POINT('Ctrl Pts',(-22.5675364832709,82.8232381806961,
81.8764274622056));
#219626=CARTESIAN_POINT('Ctrl Pts',(-22.5675364832709,82.6787893153765,
81.999396709168));
#219627=CARTESIAN_POINT('Ctrl Pts',(-22.5675364832709,82.5335582360053,
82.1230318545621));
#219628=CARTESIAN_POINT('Ctrl Pts',(-22.5675364832709,82.3856776242889,
82.2429230596935));
#219629=CARTESIAN_POINT('Ctrl Pts',(-22.5675364832709,82.2351403062011,
82.3591374574759));
#219630=CARTESIAN_POINT('Ctrl Pts',(-22.5675364832709,82.0844127264509,
82.4754987367413));
#219631=CARTESIAN_POINT('Ctrl Pts',(-22.5675364832709,81.931021378805,82.5881741645978));
#219632=CARTESIAN_POINT('Ctrl Pts',(-22.5675364832709,81.7749255723342,
82.6971910900871));
#219633=CARTESIAN_POINT('Ctrl Pts',(-22.5675364832709,81.6196215858302,
82.8056550104683));
#219634=CARTESIAN_POINT('Ctrl Pts',(-22.5675364832709,81.4616401560816,
82.9104976774395));
#219635=CARTESIAN_POINT('Ctrl Pts',(-22.5675364832709,81.3009133123836,
83.0117028803056));
#219636=CARTESIAN_POINT('Ctrl Pts',(-22.5675364832709,81.1803681796102,
83.0876067824552));
#219637=CARTESIAN_POINT('Ctrl Pts',(-22.5675364832709,81.058278152601,83.16146375779));
#219638=CARTESIAN_POINT('Ctrl Pts',(-22.5675364832709,80.9346059377799,
83.2332496877048));
#219639=CARTESIAN_POINT('Ctrl Pts',(-22.5675364832709,80.8809466249279,
83.2643964062887));
#219640=CARTESIAN_POINT('Ctrl Pts',(-22.5675364832709,80.8269893718125,
83.2951530448035));
#219641=CARTESIAN_POINT('Ctrl Pts',(-22.5675364832709,80.7727307612443,
83.325516709298));
#219642=CARTESIAN_POINT('Ctrl Pts',(-22.5675364832709,80.7409297866078,
83.3433128547273));
#219643=CARTESIAN_POINT('Ctrl Pts',(-22.5675364832709,80.7090252876808,
83.3609739976518));
#219644=CARTESIAN_POINT('Ctrl Pts',(-22.5675364832709,80.6770165441255,
83.3784994627323));
#219645=CARTESIAN_POINT('Ctrl Pts',(-22.5675364832709,80.6572219751036,
83.3893374085446));
#219646=CARTESIAN_POINT('Ctrl Pts',(-22.5675364832709,80.6373836646383,
83.400125523986));
#219647=CARTESIAN_POINT('Ctrl Pts',(-22.5675364832709,80.6175267978189,
83.4108500412261));
#219648=CARTESIAN_POINT('Ctrl Pts',(-22.5675364832709,80.4393377980143,
83.507088335906));
#219649=CARTESIAN_POINT('Ctrl Pts',(-22.5675364832709,80.2592938419621,
83.5984099220634));
#219650=CARTESIAN_POINT('Ctrl Pts',(-22.5675364832709,80.0774194424533,
83.6848466134901));
#219651=CARTESIAN_POINT('Ctrl Pts',(-22.5675364832709,79.9816186497369,
83.7303764053729));
#219652=CARTESIAN_POINT('Ctrl Pts',(-22.5675364832709,79.8853094574927,
83.7745501568457));
#219653=CARTESIAN_POINT('Ctrl Pts',(-22.5675364832709,79.7884922163416,
83.8173676866023));
#219654=CARTESIAN_POINT('Ctrl Pts',(-22.5675364832709,79.6051464451119,
83.8984525525005));
#219655=CARTESIAN_POINT('Ctrl Pts',(-22.5675364832709,79.4199800239593,
83.9746766474747));
#219656=CARTESIAN_POINT('Ctrl Pts',(-22.5675364832709,79.2330235033904,
84.0461131619167));
#219657=CARTESIAN_POINT('Ctrl Pts',(-22.5675364832709,79.0453490386799,
84.1178240044586));
#219658=CARTESIAN_POINT('Ctrl Pts',(-22.5675364832709,78.8558702756082,
84.1847105346891));
#219659=CARTESIAN_POINT('Ctrl Pts',(-22.5675364832709,78.6645986034204,
84.2467978873678));
#219660=CARTESIAN_POINT('Ctrl Pts',(-22.5675364832709,78.4733713416908,
84.30887082428));
#219661=CARTESIAN_POINT('Ctrl Pts',(-22.5675364832709,78.2803515695058,
84.3661469096114));
#219662=CARTESIAN_POINT('Ctrl Pts',(-22.5675364832709,78.0855376558692,
84.4186009739626));
#219663=CARTESIAN_POINT('Ctrl Pts',(-22.5675364832709,77.9893128513891,
84.4445097090841));
#219664=CARTESIAN_POINT('Ctrl Pts',(-22.5675364832709,77.892650173136,84.4692412399597));
#219665=CARTESIAN_POINT('Ctrl Pts',(-22.5675364832709,77.7955487498991,
84.4927878836045));
#219666=CARTESIAN_POINT('',(-22.5675364837383,86.3349224095373,76.4088722770814));
#219667=CARTESIAN_POINT('Ctrl Pts',(-22.5673829558621,86.3309582618541,
76.4209333437238));
#219668=CARTESIAN_POINT('Ctrl Pts',(-22.5674341318949,86.3322817703421,
76.4169137400224));
#219669=CARTESIAN_POINT('Ctrl Pts',(-22.5674853079278,86.3336031532802,
76.4128933831607));
#219670=CARTESIAN_POINT('Ctrl Pts',(-22.5675364839606,86.3349224096848,
76.4088722753861));
#219671=CARTESIAN_POINT('Ctrl Pts',(-22.5675364837383,86.3349224095373,
76.4088722770814));
#219672=CARTESIAN_POINT('Ctrl Pts',(-22.5862680853234,86.5592443815844,
75.6674670848345));
#219673=CARTESIAN_POINT('Ctrl Pts',(-22.6057724255725,86.7082163959447,
74.9097552024436));
#219674=CARTESIAN_POINT('Ctrl Pts',(-22.6429310858987,86.8542170642046,
73.4058157535164));
#219675=CARTESIAN_POINT('Ctrl Pts',(-22.6606405257108,86.8569370758779,
72.6625676819964));
#219676=CARTESIAN_POINT('Ctrl Pts',(-22.6917079591717,86.7417407420671,
71.3752055763466));
#219677=CARTESIAN_POINT('Ctrl Pts',(-22.7050393165119,86.6541791296153,
70.828225798091));
#219678=CARTESIAN_POINT('Ctrl Pts',(-22.7250377762276,86.4692968267006,
70.0378179720206));
#219679=CARTESIAN_POINT('Ctrl Pts',(-22.7314888115047,86.4019218698674,
69.7878453758678));
#219680=CARTESIAN_POINT('Ctrl Pts',(-22.7709634204644,85.9375775027767,
68.2665105161627));
#219681=CARTESIAN_POINT('Ctrl Pts',(-22.8027640999299,85.3320805150328,
67.058188819128));
#219682=CARTESIAN_POINT('Ctrl Pts',(-22.8537481998869,84.0928908798262,
65.3669320568875));
#219683=CARTESIAN_POINT('Ctrl Pts',(-22.8725290298923,83.5843297564767,
64.7993630234584));
#219684=CARTESIAN_POINT('Ctrl Pts',(-22.9239292449124,82.0380819403647,
63.3764671688534));
#219685=CARTESIAN_POINT('Ctrl Pts',(-22.9604267297466,80.7640570361906,
62.5103550986123));
#219686=CARTESIAN_POINT('Ctrl Pts',(-23.0202928869871,78.4706153454157,
61.6432305647928));
#219687=CARTESIAN_POINT('Ctrl Pts',(-23.0392730866337,77.7207900189858,
61.4414365269494));
#219688=CARTESIAN_POINT('Ctrl Pts',(-23.0930290504125,75.5544958242202,
61.0779603516221));
#219689=CARTESIAN_POINT('Ctrl Pts',(-23.1299594944175,73.9801568529781,
61.0706562319372));
#219690=CARTESIAN_POINT('Ctrl Pts',(-23.1905021030076,71.5870961726182,
61.6282648933797));
#219691=CARTESIAN_POINT('Ctrl Pts',(-23.209090806836,70.8699378838349,61.8685784075968));
#219692=CARTESIAN_POINT('Ctrl Pts',(-23.2410740979785,69.6615834129092,
62.4056935084534));
#219693=CARTESIAN_POINT('Ctrl Pts',(-23.2545074008348,69.157778146997,62.6745433313228));
#219694=CARTESIAN_POINT('Ctrl Pts',(-23.2863973120801,68.049292023537,63.3759610656699));
#219695=CARTESIAN_POINT('Ctrl Pts',(-23.304848079247,67.4618353137888,63.8305898999364));
#219696=CARTESIAN_POINT('Ctrl Pts',(-23.3350930669858,66.5677869315017,
64.6654052882002));
#219697=CARTESIAN_POINT('Ctrl Pts',(-23.3469809107229,66.2342709156701,
65.0169928637897));
#219698=CARTESIAN_POINT('Ctrl Pts',(-23.3689390275803,65.6479137832039,
65.7159828751924));
#219699=CARTESIAN_POINT('Ctrl Pts',(-23.3790075514597,65.3902080122086,
66.05931915499));
#219700=CARTESIAN_POINT('Ctrl Pts',(-23.3969914175802,64.9729130265417,
66.6842488965277));
#219701=CARTESIAN_POINT('Ctrl Pts',(-23.4048424767607,64.8051745741039,
66.9596772122863));
#219702=CARTESIAN_POINT('Ctrl Pts',(-23.4296186292682,64.3175556008988,
67.8394688951344));
#219703=CARTESIAN_POINT('Ctrl Pts',(-23.4468326360178,64.0380624442595,
68.4665319016422));
#219704=CARTESIAN_POINT('Ctrl Pts',(-23.4767056660225,63.641609652087,69.6102254268264));
#219705=CARTESIAN_POINT('Ctrl Pts',(-23.4894017651609,63.5020116401143,
70.119178511537));
#219706=CARTESIAN_POINT('Ctrl Pts',(-23.509717800407,63.3305870527547,70.960607381492));
#219707=CARTESIAN_POINT('Ctrl Pts',(-23.5175437050303,63.2780012942616,
71.2888547719588));
#219708=CARTESIAN_POINT('Ctrl Pts',(-23.537280129187,63.1830131244648,72.1037210969697));
#219709=CARTESIAN_POINT('Ctrl Pts',(-23.549400167054,63.1571013464539,72.5918834219285));
#219710=CARTESIAN_POINT('Ctrl Pts',(-23.5734791553166,63.1652689824181,
73.5553851328984));
#219711=CARTESIAN_POINT('Ctrl Pts',(-23.5854383058723,63.1979133534347,
74.0310234500722));
#219712=CARTESIAN_POINT('Ctrl Pts',(-23.6099759330427,63.3252210027845,
75.01885650904));
#219713=CARTESIAN_POINT('Ctrl Pts',(-23.6223585606802,63.4253801393107,
75.5304187723416));
#219714=CARTESIAN_POINT('Ctrl Pts',(-23.6423017686356,63.6419834592016,
76.3472594597781));
#219715=CARTESIAN_POINT('Ctrl Pts',(-23.64996574602,63.7382098911753,76.6579018594108));
#219716=CARTESIAN_POINT('Ctrl Pts',(-23.6713796367493,64.0366083519891,
77.4955707899602));
#219717=CARTESIAN_POINT('Ctrl Pts',(-23.6855188631018,64.2643953263507,
78.0123852988475));
#219718=CARTESIAN_POINT('Ctrl Pts',(-23.7091552450763,64.7041018085207,
78.8448886272887));
#219719=CARTESIAN_POINT('Ctrl Pts',(-23.7186618439811,64.897017806972,79.1713809851635));
#219720=CARTESIAN_POINT('Ctrl Pts',(-23.7427639934684,65.434825799796,79.9901439374208));
#219721=CARTESIAN_POINT('Ctrl Pts',(-23.7568771368583,65.8025691386141,
80.4674901565216));
#219722=CARTESIAN_POINT('Ctrl Pts',(-23.778152865229,66.4046745762888,81.1368390030206));
#219723=CARTESIAN_POINT('Ctrl Pts',(-23.7852645329274,66.613437030011,81.3518844373747));
#219724=CARTESIAN_POINT('Ctrl Pts',(-23.8051161905732,67.2061691993328,
81.917120638316));
#219725=CARTESIAN_POINT('Ctrl Pts',(-23.8181956316294,67.6056788130504,
82.2499055715368));
#219726=CARTESIAN_POINT('Ctrl Pts',(-23.8397098155045,68.2971284007469,
82.7532298693984));
#219727=CARTESIAN_POINT('Ctrl Pts',(-23.8481703871645,68.5779558868143,
82.9399204995111));
#219728=CARTESIAN_POINT('Ctrl Pts',(-23.871197050066,69.3780515501284,83.4243581701984));
#219729=CARTESIAN_POINT('Ctrl Pts',(-23.885277863819,69.9132899593637,83.6958827846302));
#219730=CARTESIAN_POINT('Ctrl Pts',(-23.9073163037073,70.7736847555396,
84.053440516099));
#219731=CARTESIAN_POINT('Ctrl Pts',(-23.9152294424713,71.0868725140369,
84.168361390285));
#219732=CARTESIAN_POINT('Ctrl Pts',(-23.9341886438321,71.8321747515983,
84.4061841008895));
#219733=CARTESIAN_POINT('Ctrl Pts',(-23.9454211520969,72.2665804198338,
84.517476771334));
#219734=CARTESIAN_POINT('Ctrl Pts',(-23.9652782132134,73.0404647072046,
84.66967294));
#219735=CARTESIAN_POINT('Ctrl Pts',(-23.9738842404024,73.3782672473474,
84.7210490326943));
#219736=CARTESIAN_POINT('Ctrl Pts',(-23.9968051979931,74.3002900610801,
84.8210702035737));
#219737=CARTESIAN_POINT('Ctrl Pts',(-24.0107033113074,74.8876684986167,
84.8413692782648));
#219738=CARTESIAN_POINT('Ctrl Pts',(-24.0340122827481,75.8702392977051,
84.8028056628792));
#219739=CARTESIAN_POINT('Ctrl Pts',(-24.043432404758,76.2664083199661,84.7673381145656));
#219740=CARTESIAN_POINT('Ctrl Pts',(-24.0646309551325,77.1334984705464,
84.6450363719972));
#219741=CARTESIAN_POINT('Ctrl Pts',(-24.0765713079441,77.6009858284274,
84.5493528448032));
#219742=CARTESIAN_POINT('Ctrl Pts',(-24.0997554081107,78.4910206834455,
84.3103135667122));
#219743=CARTESIAN_POINT('Ctrl Pts',(-24.1108807937146,78.9141664301559,
84.1706526422075));
#219744=CARTESIAN_POINT('Ctrl Pts',(-24.1385332276154,79.9731164787605,
83.7543074460724));
#219745=CARTESIAN_POINT('Ctrl Pts',(-24.1548409783277,80.5960774404369,
83.4445873668435));
#219746=CARTESIAN_POINT('Ctrl Pts',(-24.1798141076855,81.4855472211131,
82.9004178078973));
#219747=CARTESIAN_POINT('Ctrl Pts',(-24.1882658800546,81.7757939264851,
82.7046570188048));
#219748=CARTESIAN_POINT('Ctrl Pts',(-24.2064651621941,82.3680756726774,
82.2650889548938));
#219749=CARTESIAN_POINT('Ctrl Pts',(-24.2162594926789,82.6677628545046,
82.0184893106646));
#219750=CARTESIAN_POINT('Ctrl Pts',(-24.2503354667517,83.6759547075801,
81.1023758653179));
#219751=CARTESIAN_POINT('Ctrl Pts',(-24.2734890978271,84.3165658354487,
80.3575421127005));
#219752=CARTESIAN_POINT('Ctrl Pts',(-24.3359484975005,85.7610812345458,
78.1900043195256));
#219753=CARTESIAN_POINT('Ctrl Pts',(-24.3698713517959,86.2160492920742,
76.9116039690565));
#219754=CARTESIAN_POINT('Ctrl Pts',(-24.4133074766063,86.6618899759425,
75.1700668662206));
#219755=CARTESIAN_POINT('Ctrl Pts',(-24.4319587440237,86.7814690924183,
74.3940693434564));
#219756=CARTESIAN_POINT('Ctrl Pts',(-24.4613547807652,86.8459689720956,
73.1896082034861));
#219757=CARTESIAN_POINT('Ctrl Pts',(-24.4718526033559,86.8455610485519,
72.7660588280728));
#219758=CARTESIAN_POINT('Ctrl Pts',(-24.5046971488066,86.7721213111656,
71.4411529564219));
#219759=CARTESIAN_POINT('Ctrl Pts',(-24.5265462495201,86.6185082957646,
70.5461094578341));
#219760=CARTESIAN_POINT('Ctrl Pts',(-24.5670051429742,86.1518862619208,
68.9404605247924));
#219761=CARTESIAN_POINT('Ctrl Pts',(-24.5856817309166,85.8651065517316,
68.2206283273154));
#219762=CARTESIAN_POINT('Ctrl Pts',(-24.6232006790467,85.1612979160907,
66.8653478737751));
#219763=CARTESIAN_POINT('Ctrl Pts',(-24.6416611232624,84.7487848589079,
66.2297978498545));
#219764=CARTESIAN_POINT('Ctrl Pts',(-24.6882468904586,83.5623680174767,
64.7326308652746));
#219765=CARTESIAN_POINT('Ctrl Pts',(-24.7260382386136,82.4438732841827,
63.5847792685476));
#219766=CARTESIAN_POINT('Ctrl Pts',(-24.7917113773775,80.1048899714854,
62.2801640674017));
#219767=CARTESIAN_POINT('Ctrl Pts',(-24.8105835909982,79.3983530500854,
61.9711661347939));
#219768=CARTESIAN_POINT('Ctrl Pts',(-24.8476505405666,77.9512541423471,
61.4982879163466));
#219769=CARTESIAN_POINT('Ctrl Pts',(-24.8656179042796,77.2118140491652,
61.332268975595));
#219770=CARTESIAN_POINT('Ctrl Pts',(-24.9052918234955,75.5975429275466,
61.1330685277027));
#219771=CARTESIAN_POINT('Ctrl Pts',(-24.9268693700258,74.7252280093247,
61.1221140290984));
#219772=CARTESIAN_POINT('Ctrl Pts',(-24.9577085382453,73.4737815980774,
61.242481028318));
#219773=CARTESIAN_POINT('Ctrl Pts',(-24.967217719536,73.0871932428302,61.2988750337921));
#219774=CARTESIAN_POINT('Ctrl Pts',(-24.9905520650349,72.1351244908571,
61.4862146028957));
#219775=CARTESIAN_POINT('Ctrl Pts',(-25.0042103174994,71.5757510543634,
61.6397751316705));
#219776=CARTESIAN_POINT('Ctrl Pts',(-25.0335288217218,70.4461743726575,
62.0429563473559));
#219777=CARTESIAN_POINT('Ctrl Pts',(-25.0489253600611,69.8810709729959,
62.2963153262076));
#219778=CARTESIAN_POINT('Ctrl Pts',(-25.0800666050386,68.7772565000667,
62.8976245619141));
#219779=CARTESIAN_POINT('Ctrl Pts',(-25.0957726872494,68.2400647626968,
63.2487373898093));
#219780=CARTESIAN_POINT('Ctrl Pts',(-25.1193718523531,67.4564988289902,
63.8566578125516));
#219781=CARTESIAN_POINT('Ctrl Pts',(-25.1276624343069,67.1879359315394,
64.0849197521976));
#219782=CARTESIAN_POINT('Ctrl Pts',(-25.1454609563539,66.6454867103185,
64.5900982371163));
#219783=CARTESIAN_POINT('Ctrl Pts',(-25.1550148296095,66.3742407038714,
64.8694283428638));
#219784=CARTESIAN_POINT('Ctrl Pts',(-25.1821367707909,65.651765776175,65.6906711367853));
#219785=CARTESIAN_POINT('Ctrl Pts',(-25.1999107406031,65.233294526125,66.261769242973));
#219786=CARTESIAN_POINT('Ctrl Pts',(-25.2283952223487,64.630334717106,67.2584876519789));
#219787=CARTESIAN_POINT('Ctrl Pts',(-25.2393089263833,64.4150568461714,
67.6656532103755));
#219788=CARTESIAN_POINT('Ctrl Pts',(-25.261057263207,64.0330799276992,68.5030414663998));
#219789=CARTESIAN_POINT('Ctrl Pts',(-25.2719955468723,63.8668808019813,
68.9323993214274));
#219790=CARTESIAN_POINT('Ctrl Pts',(-25.2937880673866,63.5965624296136,
69.7767493402305));
#219791=CARTESIAN_POINT('Ctrl Pts',(-25.3044379286782,63.4890325077483,
70.1883156831887));
#219792=CARTESIAN_POINT('Ctrl Pts',(-25.3293736091068,63.2891448861663,
71.1638320986694));
#219793=CARTESIAN_POINT('Ctrl Pts',(-25.3436387852029,63.2147405508323,
71.7315450266966));
#219794=CARTESIAN_POINT('Ctrl Pts',(-25.3658368888776,63.1605775869907,
72.6541834421041));
#219795=CARTESIAN_POINT('Ctrl Pts',(-25.3741450297437,63.1555385000925,
73.007689085589));
#219796=CARTESIAN_POINT('Ctrl Pts',(-25.3932547504681,63.1802915989499,
73.8167754615166));
#219797=CARTESIAN_POINT('Ctrl Pts',(-25.4041146979201,63.2206674555497,
74.2716084565794));
#219798=CARTESIAN_POINT('Ctrl Pts',(-25.424894620039,63.3446571966042,75.1053687246365));
#219799=CARTESIAN_POINT('Ctrl Pts',(-25.4345780693059,63.4200964155568,
75.4834915305247));
#219800=CARTESIAN_POINT('Ctrl Pts',(-25.4567619973944,63.6347127373887,
76.3401422706014));
#219801=CARTESIAN_POINT('Ctrl Pts',(-25.4692500578771,63.7861020015207,
76.8156577037989));
#219802=CARTESIAN_POINT('Ctrl Pts',(-25.4890094659493,64.0819679904328,
77.5769828960174));
#219803=CARTESIAN_POINT('Ctrl Pts',(-25.4965644957773,64.2093291045492,
77.8694937917293));
#219804=CARTESIAN_POINT('Ctrl Pts',(-25.5177272011169,64.5997762794745,
78.6759683205503));
#219805=CARTESIAN_POINT('Ctrl Pts',(-25.5313223378866,64.8895155036546,
79.1778737046292));
#219806=CARTESIAN_POINT('Ctrl Pts',(-25.553961967557,65.4070878364213,79.93673654872));
#219807=CARTESIAN_POINT('Ctrl Pts',(-25.562477621451,65.6101301943096,80.2082748200485));
#219808=CARTESIAN_POINT('Ctrl Pts',(-25.5838503196473,66.1473713131949,
80.8660090615544));
#219809=CARTESIAN_POINT('Ctrl Pts',(-25.596696390321,66.4958853551464,81.2405495881967));
#219810=CARTESIAN_POINT('Ctrl Pts',(-25.6174987374245,67.1198671630634,
81.8305356652852));
#219811=CARTESIAN_POINT('Ctrl Pts',(-25.6257626286478,67.3833471538268,
82.0587208875555));
#219812=CARTESIAN_POINT('Ctrl Pts',(-25.6481489502373,68.1250610693869,
82.6461857161893));
#219813=CARTESIAN_POINT('Ctrl Pts',(-25.6622524342847,68.6223957292458,
82.9825882016476));
#219814=CARTESIAN_POINT('Ctrl Pts',(-25.6849535707228,69.4223463877076,
83.4376350608614));
#219815=CARTESIAN_POINT('Ctrl Pts',(-25.6930171765534,69.7074615873909,
83.5846073202147));
#219816=CARTESIAN_POINT('Ctrl Pts',(-25.7146507220582,70.4865706602702,
83.946966015049));
#219817=CARTESIAN_POINT('Ctrl Pts',(-25.7281391359254,70.9906139565075,
84.1408019798077));
#219818=CARTESIAN_POINT('Ctrl Pts',(-25.7520876074811,71.938816783935,84.4337245706673));
#219819=CARTESIAN_POINT('Ctrl Pts',(-25.762810865982,72.3799073071065,84.5429585790459));
#219820=CARTESIAN_POINT('Ctrl Pts',(-25.7851622316922,73.3050912650405,
84.7165901495142));
#219821=CARTESIAN_POINT('Ctrl Pts',(-25.7968063426039,73.7901466473484,
84.7770486933696));
#219822=CARTESIAN_POINT('Ctrl Pts',(-25.8166416512065,74.5925067179341,
84.8260692378714));
#219823=CARTESIAN_POINT('Ctrl Pts',(-25.8245878850798,74.9084143096501,
84.8324891107669));
#219824=CARTESIAN_POINT('Ctrl Pts',(-25.846126398411,75.7648310579256,84.8155658720624));
#219825=CARTESIAN_POINT('Ctrl Pts',(-25.8595502609576,76.3048734411851,
84.7677371052777));
#219826=CARTESIAN_POINT('Ctrl Pts',(-25.8870929365118,77.4331091242953,
84.5901671073612));
#219827=CARTESIAN_POINT('Ctrl Pts',(-25.9012958491276,78.0200692131477,
84.4518600552283));
#219828=CARTESIAN_POINT('Ctrl Pts',(-25.9262597884438,79.0123812129266,
84.1367233640231));
#219829=CARTESIAN_POINT('Ctrl Pts',(-25.9369484716107,79.4245662099935,
83.9800739201575));
#219830=CARTESIAN_POINT('Ctrl Pts',(-25.9593084055024,80.2444445516244,
83.6136503722892));
#219831=CARTESIAN_POINT('Ctrl Pts',(-25.970864562363,80.6503056040749,83.4029204272697));
#219832=CARTESIAN_POINT('Ctrl Pts',(-25.9938343662642,81.4514752177107,
82.9265531223943));
#219833=CARTESIAN_POINT('Ctrl Pts',(-26.005310034174,81.8456631486792,82.6589885236724));
#219834=CARTESIAN_POINT('Ctrl Pts',(-26.0343820127005,82.8058647548344,
81.9199778941042));
#219835=CARTESIAN_POINT('Ctrl Pts',(-26.0518964723227,83.3478025042898,
81.4170463577296));
#219836=CARTESIAN_POINT('Ctrl Pts',(-26.0820442935122,84.165826779719,80.5001478590155));
#219837=CARTESIAN_POINT('Ctrl Pts',(-26.0944271911139,84.469305924103,80.112925251043));
#219838=CARTESIAN_POINT('Ctrl Pts',(-26.1225191227799,85.1145478269457,
79.1752815467396));
#219839=CARTESIAN_POINT('Ctrl Pts',(-26.1381663634797,85.4379364210402,
78.6116580075921));
#219840=CARTESIAN_POINT('Ctrl Pts',(-26.1721088657875,86.0376628276095,
77.3370325344322));
#219841=CARTESIAN_POINT('Ctrl Pts',(-26.1904008122117,86.2958999687812,
76.6173315306904));
#219842=CARTESIAN_POINT('Ctrl Pts',(-26.2163069038108,86.5528168983806,
75.5971963120996));
#219843=CARTESIAN_POINT('Ctrl Pts',(-26.2235318340171,86.613186429361,75.3127304874102));
#219844=CARTESIAN_POINT('Ctrl Pts',(-26.2587554148366,86.8580316646618,
73.9047778024851));
#219845=CARTESIAN_POINT('Ctrl Pts',(-26.286223815663,86.890533153244,72.75432961077));
#219846=CARTESIAN_POINT('Ctrl Pts',(-26.3415801754294,86.6292934641588,
70.4878602924608));
#219847=CARTESIAN_POINT('Ctrl Pts',(-26.3693494802877,86.3347180294922,
69.3856928759218));
#219848=CARTESIAN_POINT('Ctrl Pts',(-26.3971183084764,85.8880607550622,
68.3407934129425));
#219849=CARTESIAN_POINT('Ctrl Pts',(-31.6489087198709,70.0959712176063,
60.8783100640841));
#219850=CARTESIAN_POINT('Ctrl Pts',(-31.6814645153009,68.7303325189268,
61.4313085050616));
#219851=CARTESIAN_POINT('Ctrl Pts',(-31.7465761061609,66.1882700076009,
63.0035716608669));
#219852=CARTESIAN_POINT('Ctrl Pts',(-31.8442434924509,63.3737498322777,
66.4939579958501));
#219853=CARTESIAN_POINT('Ctrl Pts',(-31.9419108787409,61.8771905500222,
70.7205438274275));
#219854=CARTESIAN_POINT('Ctrl Pts',(-32.0395782650309,61.8681403166308,
75.2042647157331));
#219855=CARTESIAN_POINT('Ctrl Pts',(-32.1372456513209,63.3476500679026,
79.4368608152641));
#219856=CARTESIAN_POINT('Ctrl Pts',(-32.2349130376109,66.1480040818002,
82.9385512545613));
#219857=CARTESIAN_POINT('Ctrl Pts',(-32.3325804239009,69.9517715767027,
85.3124031224554));
#219858=CARTESIAN_POINT('Ctrl Pts',(-32.4302478101809,74.3277781103001,
86.2893299487034));
#219859=CARTESIAN_POINT('Ctrl Pts',(-32.5279151964709,78.7799840116568,
85.7585926810094));
#219860=CARTESIAN_POINT('Ctrl Pts',(-32.6255825827609,82.8037119089286,
83.7803527627689));
#219861=CARTESIAN_POINT('Ctrl Pts',(-32.7232499690509,85.9428543612762,
80.5788524819328));
#219862=CARTESIAN_POINT('Ctrl Pts',(-32.8209173553409,87.8415756099131,
76.5169961329518));
#219863=CARTESIAN_POINT('Ctrl Pts',(-32.9185847416309,88.2846471586345,
72.0552131952207));
#219864=CARTESIAN_POINT('Ctrl Pts',(-33.0162521279209,87.2218448769265,
67.6992666057196));
#219865=CARTESIAN_POINT('Ctrl Pts',(-33.1139195142109,84.7736421296089,
63.9429222806305));
#219866=CARTESIAN_POINT('Ctrl Pts',(-33.2115869005009,81.2175535848858,
61.2119785531442));
#219867=CARTESIAN_POINT('Ctrl Pts',(-33.3092542867909,76.9566776927288,
59.8160000388975));
#219868=CARTESIAN_POINT('Ctrl Pts',(-33.4069216730809,72.4740036830308,
59.9132271101949));
#219869=CARTESIAN_POINT('Ctrl Pts',(-33.5045890593709,68.2776625886137,
61.4926386461447));
#219870=CARTESIAN_POINT('Ctrl Pts',(-33.6022564456609,64.8433283330666,
64.3752013257362));
#219871=CARTESIAN_POINT('Ctrl Pts',(-33.6999238319509,62.56029797625,68.2341638508804));
#219872=CARTESIAN_POINT('Ctrl Pts',(-33.7975912182409,61.6873631614363,
72.6320956590941));
#219873=CARTESIAN_POINT('Ctrl Pts',(-33.8952586045309,62.3234749316971,
77.0704716229308));
#219874=CARTESIAN_POINT('Ctrl Pts',(-33.9929259908209,64.3965271891681,
81.0461820900504));
#219875=CARTESIAN_POINT('Ctrl Pts',(-34.0905933771109,67.6715302419011,
84.1085625995897));
#219876=CARTESIAN_POINT('Ctrl Pts',(-34.1882607634009,71.7772479303871,
85.9104787028145));
#219877=CARTESIAN_POINT('Ctrl Pts',(-34.2859281496909,76.2482788970921,
86.247675196548));
#219878=CARTESIAN_POINT('Ctrl Pts',(-34.3835955359809,80.5778118998904,
85.081929358769));
#219879=CARTESIAN_POINT('Ctrl Pts',(-34.4812629222709,84.2750751200944,
82.5453836640971));
#219880=CARTESIAN_POINT('Ctrl Pts',(-34.5789303085609,86.9209673304724,
78.9255668466804));
#219881=CARTESIAN_POINT('Ctrl Pts',(-34.6765976948509,88.2155648830812,
74.6328012395938));
#219882=CARTESIAN_POINT('Ctrl Pts',(-34.7742650811409,88.0121193884434,
70.1536909137269));
#219883=CARTESIAN_POINT('Ctrl Pts',(-34.8719324674309,86.333692298055,65.995962942479));
#219884=CARTESIAN_POINT('Ctrl Pts',(-34.9695998537209,83.3705407863494,
62.6309142802354));
#219885=CARTESIAN_POINT('Ctrl Pts',(-35.0672672400109,79.4585512538933,
60.4399881567567));
#219886=CARTESIAN_POINT('Ctrl Pts',(-35.1649346263009,75.0411651102624,
59.6715357908677));
#219887=CARTESIAN_POINT('Ctrl Pts',(-35.2626020125909,70.6191127183272,
60.4126646754531));
#219888=CARTESIAN_POINT('Ctrl Pts',(-35.3602693988809,66.6936533809556,
62.5793645557409));
#219889=CARTESIAN_POINT('Ctrl Pts',(-35.4579367851709,63.7097553700125,
65.9260303652965));
#219890=CARTESIAN_POINT('Ctrl Pts',(-35.5556041714609,62.005656794,70.0733026524509));
#219891=CARTESIAN_POINT('Ctrl Pts',(-35.6532715577509,61.7745248044076,
74.5510696611246));
#219892=CARTESIAN_POINT('Ctrl Pts',(-35.7509389440409,63.0425592400513,
78.8517565888796));
#219893=CARTESIAN_POINT('Ctrl Pts',(-35.8486063303309,65.6660227588901,
82.4878614479098));
#219894=CARTESIAN_POINT('Ctrl Pts',(-35.9462737166209,69.3475341048888,
85.0472155832));
#219895=CARTESIAN_POINT('Ctrl Pts',(-36.0439411029109,73.6697775958153,
86.239704822428));
#219896=CARTESIAN_POINT('Ctrl Pts',(-36.1416084892009,78.142807711568,85.9301552074927));
#219897=CARTESIAN_POINT('Ctrl Pts',(-36.2392758754909,82.2595865975891,
84.1536555637811));
#219898=CARTESIAN_POINT('Ctrl Pts',(-36.3369432617809,85.5534590604176,
81.111580025743));
#219899=CARTESIAN_POINT('Ctrl Pts',(-36.4346106480709,87.6510500090054,
77.1487613832987));
#219900=CARTESIAN_POINT('Ctrl Pts',(-36.5322780343609,88.3145881816426,
72.7144027516668));
#219901=CARTESIAN_POINT('Ctrl Pts',(-36.6299454206509,87.4688585758041,
68.3111584007035));
#219902=CARTESIAN_POINT('Ctrl Pts',(-36.7276128069509,85.2097284031102,
64.4381556582015));
#219903=CARTESIAN_POINT('Ctrl Pts',(-36.8252801932409,81.793280114859,61.534416607706));
#219904=CARTESIAN_POINT('Ctrl Pts',(-36.9229475795309,77.6067833162661,
59.9290929831489));
#219905=CARTESIAN_POINT('Ctrl Pts',(-37.0206149658209,73.124796038894,59.8041553558838));
#219906=CARTESIAN_POINT('Ctrl Pts',(-37.1182823521109,68.8553714613998,
61.1737659619935));
#219907=CARTESIAN_POINT('Ctrl Pts',(-37.2159497384009,65.2824678824627,
63.8826733471558));
#219908=CARTESIAN_POINT('Ctrl Pts',(-37.3136171246909,62.8110896717617,
67.6238108193035));
#219909=CARTESIAN_POINT('Ctrl Pts',(-37.4112845109809,61.7213790587936,
71.9731037866268));
#219910=CARTESIAN_POINT('Ctrl Pts',(-37.5089518972709,62.1368576487401,
76.4375406365595));
#219911=CARTESIAN_POINT('Ctrl Pts',(-37.6066192835609,64.010436330763,80.5110572786137));
#219912=CARTESIAN_POINT('Ctrl Pts',(-37.7042866698509,67.1297096286665,
83.7319036844192));
#219913=CARTESIAN_POINT('Ctrl Pts',(-37.8019540561409,71.1411948124404,
85.7349781226078));
#219914=CARTESIAN_POINT('Ctrl Pts',(-37.8670656470009,74.1069290187816,
86.1071526244663));
#219915=CARTESIAN_POINT('Ctrl Pts',(-37.8996214424309,75.5788379419391,
86.0418804791266));
#219916=CARTESIAN_POINT('Ctrl Pts',(-31.8730368301509,70.2575692325718,
61.2773790062616));
#219917=CARTESIAN_POINT('Ctrl Pts',(-31.9055926255809,68.9369311879788,
61.8121549909076));
#219918=CARTESIAN_POINT('Ctrl Pts',(-31.9707042164409,66.4786349582126,
63.3326087841967));
#219919=CARTESIAN_POINT('Ctrl Pts',(-32.0683716027309,63.7568591148654,
66.7079795823175));
#219920=CARTESIAN_POINT('Ctrl Pts',(-32.1660389890109,62.3096145940082,
70.7952905623853));
#219921=CARTESIAN_POINT('Ctrl Pts',(-32.2637063753009,62.3008625847488,
75.1312634607482));
#219922=CARTESIAN_POINT('Ctrl Pts',(-32.3613737615909,63.7316193923605,
79.224386657865));
#219923=CARTESIAN_POINT('Ctrl Pts',(-32.4590411478809,66.4396958789624,
82.610689066389));
#219924=CARTESIAN_POINT('Ctrl Pts',(-32.5567085341709,70.1181212717175,
84.9063175455788));
#219925=CARTESIAN_POINT('Ctrl Pts',(-32.6543759204609,74.3499292288595,
85.8510525877097));
#219926=CARTESIAN_POINT('Ctrl Pts',(-32.7520433067509,78.6554256250739,
85.3378042240803));
#219927=CARTESIAN_POINT('Ctrl Pts',(-32.8497106930409,82.5465632644516,
83.4247514525909));
#219928=CARTESIAN_POINT('Ctrl Pts',(-32.9473780793309,85.5822644011988,
80.32874730835));
#219929=CARTESIAN_POINT('Ctrl Pts',(-33.0450454656209,87.4184188097211,
76.4007376295671));
#219930=CARTESIAN_POINT('Ctrl Pts',(-33.1427128519109,87.8468902233397,
72.0859797803774));
#219931=CARTESIAN_POINT('Ctrl Pts',(-33.2403802382009,86.8191095017967,
67.8735707501784));
#219932=CARTESIAN_POINT('Ctrl Pts',(-33.3380476244909,84.4515801603142,
64.2410058345146));
#219933=CARTESIAN_POINT('Ctrl Pts',(-33.4357150107809,81.0126721778146,
61.6000524200778));
#219934=CARTESIAN_POINT('Ctrl Pts',(-33.5333823970709,76.8922010664508,
60.250074320352));
#219935=CARTESIAN_POINT('Ctrl Pts',(-33.6310497833609,72.5572405498546,
60.3440975560973));
#219936=CARTESIAN_POINT('Ctrl Pts',(-33.7287171696509,68.4991776795392,
61.8714641754451));
#219937=CARTESIAN_POINT('Ctrl Pts',(-33.8263845559409,65.1780119274846,
64.6590403800947));
#219938=CARTESIAN_POINT('Ctrl Pts',(-33.9240519422309,62.9702122004541,
68.390842011297));
#219939=CARTESIAN_POINT('Ctrl Pts',(-34.0217193285209,62.1260424152783,
72.6438527593594));
#219940=CARTESIAN_POINT('Ctrl Pts',(-34.1193867148109,62.7411929710006,
76.9359749434432));
#219941=CARTESIAN_POINT('Ctrl Pts',(-34.2170541010909,64.7459338166531,
80.780677427527));
#219942=CARTESIAN_POINT('Ctrl Pts',(-34.3147214873809,67.9130186625803,
83.7421460881763));
#219943=CARTESIAN_POINT('Ctrl Pts',(-34.4123888736709,71.8834443579084,
85.484685283491));
#219944=CARTESIAN_POINT('Ctrl Pts',(-34.5100562599609,76.2071454941548,
85.8107704468362));
#219945=CARTESIAN_POINT('Ctrl Pts',(-34.6077236462509,80.3940113206321,
84.6834383749048));
#219946=CARTESIAN_POINT('Ctrl Pts',(-34.7053910325409,83.9694419775097,
82.2304771711338));
#219947=CARTESIAN_POINT('Ctrl Pts',(-34.8030584188309,86.5281465003784,
78.729940895939));
#219948=CARTESIAN_POINT('Ctrl Pts',(-34.9007258051209,87.7800843533953,
74.5786309025152));
#219949=CARTESIAN_POINT('Ctrl Pts',(-34.9983931914109,87.5833428137125,
70.2471166389011));
#219950=CARTESIAN_POINT('Ctrl Pts',(-35.0960605777009,85.9602234097461,
66.2263945085208));
#219951=CARTESIAN_POINT('Ctrl Pts',(-35.1937279639909,83.0947139437118,
62.9722312444263));
#219952=CARTESIAN_POINT('Ctrl Pts',(-35.2913953502809,79.3116326561084,
60.8535007234067));
#219953=CARTESIAN_POINT('Ctrl Pts',(-35.3890627365809,75.0398086337074,
60.1103704717333));
#219954=CARTESIAN_POINT('Ctrl Pts',(-35.4867301228709,70.7634721256552,
60.8270776080123));
#219955=CARTESIAN_POINT('Ctrl Pts',(-35.5843975091609,66.967364891402,62.9223801912565));
#219956=CARTESIAN_POINT('Ctrl Pts',(-35.6820648954509,64.0817925667024,
66.1587663561376));
#219957=CARTESIAN_POINT('Ctrl Pts',(-35.7797322817409,62.433847606303,70.1693773391154));
#219958=CARTESIAN_POINT('Ctrl Pts',(-35.8773996680309,62.2103318996323,
74.4995925506424));
#219959=CARTESIAN_POINT('Ctrl Pts',(-35.9750670543209,63.4365819459936,
78.6585628406411));
#219960=CARTESIAN_POINT('Ctrl Pts',(-36.0727344406109,65.9735968496646,
82.1748504323778));
#219961=CARTESIAN_POINT('Ctrl Pts',(-36.1704018269009,69.5337946895659,
84.6498684909033));
#219962=CARTESIAN_POINT('Ctrl Pts',(-36.2680692131909,73.7136112088471,
85.8030627132265));
#219963=CARTESIAN_POINT('Ctrl Pts',(-36.3657365994809,78.0392456179921,
85.5037134061586));
#219964=CARTESIAN_POINT('Ctrl Pts',(-36.4634039857709,82.0203680212412,
83.7857531448031));
#219965=CARTESIAN_POINT('Ctrl Pts',(-36.5610713720609,85.2057004907068,
80.8439203643352));
#219966=CARTESIAN_POINT('Ctrl Pts',(-36.6587387583509,87.2341714262334,
77.0116848923229));
#219967=CARTESIAN_POINT('Ctrl Pts',(-36.7564061446409,87.8758446269618,
72.7234476609321));
#219968=CARTESIAN_POINT('Ctrl Pts',(-36.8540735309309,87.0579835821749,
68.4652994295259));
#219969=CARTESIAN_POINT('Ctrl Pts',(-36.9517409172209,84.873296478161,64.7199202355244));
#219970=CARTESIAN_POINT('Ctrl Pts',(-37.0494083035109,81.5694273133449,
61.9118654657189));
#219971=CARTESIAN_POINT('Ctrl Pts',(-37.1470756898009,77.520884348699,60.3594406153311));
#219972=CARTESIAN_POINT('Ctrl Pts',(-37.2447430760909,73.1865879351576,
60.238619944442));
#219973=CARTESIAN_POINT('Ctrl Pts',(-37.3424104623809,69.0578498355331,
61.5630990137956));
#219974=CARTESIAN_POINT('Ctrl Pts',(-37.4400778486709,65.602680909391,64.1827422295159));
#219975=CARTESIAN_POINT('Ctrl Pts',(-37.5377452349609,63.2127397845698,
67.8006013898867));
#219976=CARTESIAN_POINT('Ctrl Pts',(-37.6354126212509,62.1589374176099,
72.0065760486925));
#219977=CARTESIAN_POINT('Ctrl Pts',(-37.7330800075509,62.5607251182124,
76.3239003581206));
#219978=CARTESIAN_POINT('Ctrl Pts',(-37.8307473938409,64.3725654603181,
80.2631860989099));
#219979=CARTESIAN_POINT('Ctrl Pts',(-37.9284147801309,67.3890521728565,
83.3778988728009));
#219980=CARTESIAN_POINT('Ctrl Pts',(-38.0260821664209,71.2683505217792,
85.3149678148183));
#219981=CARTESIAN_POINT('Ctrl Pts',(-38.0911937572809,74.1363575772585,
85.6748783876892));
#219982=CARTESIAN_POINT('Ctrl Pts',(-38.1237495527109,75.5597640199593,
85.6117570961773));
#219983=CARTESIAN_POINT('Ctrl Pts',(-32.0971649404209,70.4191672475379,
61.6764479484404));
#219984=CARTESIAN_POINT('Ctrl Pts',(-32.1297207358509,69.1435298570313,
62.1930014767527));
#219985=CARTESIAN_POINT('Ctrl Pts',(-32.1948323267109,66.7689999088247,
63.6616459075254));
#219986=CARTESIAN_POINT('Ctrl Pts',(-32.2924997130009,64.1399683974443,
66.9220011687802));
#219987=CARTESIAN_POINT('Ctrl Pts',(-32.3901670992909,62.7420386379846,
70.8700372973402));
#219988=CARTESIAN_POINT('Ctrl Pts',(-32.4878344855809,62.7335848528663,
75.0582622057643));
#219989=CARTESIAN_POINT('Ctrl Pts',(-32.5855018718709,64.1155887168238,
79.0119125004583));
#219990=CARTESIAN_POINT('Ctrl Pts',(-32.6831692581609,66.7313876761263,
82.2828268782175));
#219991=CARTESIAN_POINT('Ctrl Pts',(-32.7808366444509,70.2844709667367,
84.500231968704));
#219992=CARTESIAN_POINT('Ctrl Pts',(-32.8785040307409,74.3720803474283,
85.4127752267091));
#219993=CARTESIAN_POINT('Ctrl Pts',(-32.9761714170309,78.5308672385013,
84.9170157671447));
#219994=CARTESIAN_POINT('Ctrl Pts',(-33.0738388033209,82.2894146199872,
83.0691501424084));
#219995=CARTESIAN_POINT('Ctrl Pts',(-33.1715061896109,85.2216744411351,
80.0786421347599));
#219996=CARTESIAN_POINT('Ctrl Pts',(-33.2691735759009,86.9952620095349,
76.2844791261685));
#219997=CARTESIAN_POINT('Ctrl Pts',(-33.3668409621909,87.4091332880509,
72.1167463655193));
#219998=CARTESIAN_POINT('Ctrl Pts',(-33.4645083484809,86.4163741266587,
68.0478748946176));
#219999=CARTESIAN_POINT('Ctrl Pts',(-33.5621757347709,84.1295181910076,
64.5390893883722));
#220000=CARTESIAN_POINT('Ctrl Pts',(-33.6598431210609,80.8077907707222,
61.9881262869919));
#220001=CARTESIAN_POINT('Ctrl Pts',(-33.7575105073509,76.8277244401432,
60.684148601805));
#220002=CARTESIAN_POINT('Ctrl Pts',(-33.8551778936409,72.6404774166431,
60.7749680020176));
#220003=CARTESIAN_POINT('Ctrl Pts',(-33.9528452799309,68.7206927704309,
62.2502897047617));
#220004=CARTESIAN_POINT('Ctrl Pts',(-34.0505126662209,65.5126955218893,
64.9428794344855));
#220005=CARTESIAN_POINT('Ctrl Pts',(-34.1481800525109,63.3801264246425,
68.5475201717517));
#220006=CARTESIAN_POINT('Ctrl Pts',(-34.2458474388009,62.5647216691142,
72.6556098596656));
#220007=CARTESIAN_POINT('Ctrl Pts',(-34.3435148250909,63.1589110103241,
76.8014782640017));
#220008=CARTESIAN_POINT('Ctrl Pts',(-34.4411822113809,65.0953404441711,
80.5151727650388));
#220009=CARTESIAN_POINT('Ctrl Pts',(-34.5388495976709,68.1545070833008,
83.3757295768015));
#220010=CARTESIAN_POINT('Ctrl Pts',(-34.6365169839609,71.9896407854853,
85.0588918641796));
#220011=CARTESIAN_POINT('Ctrl Pts',(-34.7341843702509,76.1660120912788,
85.3738656971174));
#220012=CARTESIAN_POINT('Ctrl Pts',(-34.8318517565409,80.2102107414312,
84.2849473910145));
#220013=CARTESIAN_POINT('Ctrl Pts',(-34.9295191428309,83.6638088349665,
81.9155706781228));
#220014=CARTESIAN_POINT('Ctrl Pts',(-35.0271865291209,86.1353256703195,
78.5343149451388));
#220015=CARTESIAN_POINT('Ctrl Pts',(-35.1248539154109,87.3446038237169,
74.5244605653662));
#220016=CARTESIAN_POINT('Ctrl Pts',(-35.2225213017009,87.1545662389771,
70.3405423640075));
#220017=CARTESIAN_POINT('Ctrl Pts',(-35.3201886879909,85.5867545214038,
66.4568260744839));
#220018=CARTESIAN_POINT('Ctrl Pts',(-35.4178560742809,82.818887101022,63.3135482085524));
#220019=CARTESIAN_POINT('Ctrl Pts',(-35.5155234605709,79.1647140582467,
61.2670132900358));
#220020=CARTESIAN_POINT('Ctrl Pts',(-35.6131908468609,75.0384521570716,
60.5492051525981));
#220021=CARTESIAN_POINT('Ctrl Pts',(-35.7108582331509,70.9078315329049,
61.2414905405987));
#220022=CARTESIAN_POINT('Ctrl Pts',(-35.8085256194409,67.2410764017834,
63.2653958268243));
#220023=CARTESIAN_POINT('Ctrl Pts',(-35.9061930057309,64.4538297633518,
66.3915023470505));
#220024=CARTESIAN_POINT('Ctrl Pts',(-36.0038603920209,62.8620384185835,
70.2654520258604));
#220025=CARTESIAN_POINT('Ctrl Pts',(-36.1015277783109,62.6461389948745,
74.4481154402485));
#220026=CARTESIAN_POINT('Ctrl Pts',(-36.1991951646009,63.8306046519742,
78.4653690924802));
#220027=CARTESIAN_POINT('Ctrl Pts',(-36.2968625508909,66.2811709404978,
81.8618394169132));
#220028=CARTESIAN_POINT('Ctrl Pts',(-36.3945299371809,69.7200552743181,
84.2525213986484));
#220029=CARTESIAN_POINT('Ctrl Pts',(-36.4921973234709,73.7574448219614,
85.3664206040375));
#220030=CARTESIAN_POINT('Ctrl Pts',(-36.5898647097609,77.935683524501,85.0772716047947));
#220031=CARTESIAN_POINT('Ctrl Pts',(-36.6875320960509,81.7811494449743,
83.4178507257861));
#220032=CARTESIAN_POINT('Ctrl Pts',(-36.7851994823409,84.8579419210346,
80.5762607028601));
#220033=CARTESIAN_POINT('Ctrl Pts',(-36.8828668686309,86.8172928434819,
76.8746084012713));
#220034=CARTESIAN_POINT('Ctrl Pts',(-36.9805342549209,87.4371010722797,
72.7324925701221));
#220035=CARTESIAN_POINT('Ctrl Pts',(-37.0782016412109,86.6471085885194,
68.6194404582812));
#220036=CARTESIAN_POINT('Ctrl Pts',(-37.1758690275009,84.5368645531706,
65.0016848127869));
#220037=CARTESIAN_POINT('Ctrl Pts',(-37.2735364137909,81.3455745117745,
62.2893143236978));
#220038=CARTESIAN_POINT('Ctrl Pts',(-37.3712038000809,77.4349853810736,
60.7897882475));
#220039=CARTESIAN_POINT('Ctrl Pts',(-37.4688711863709,73.2483798313682,
60.6730845330001));
#220040=CARTESIAN_POINT('Ctrl Pts',(-37.5665385726609,69.2603282096219,
61.9524320656215));
#220041=CARTESIAN_POINT('Ctrl Pts',(-37.6642059589509,65.9228939362941,
64.4828111119111));
#220042=CARTESIAN_POINT('Ctrl Pts',(-37.7618733452409,63.6143898973541,
67.9773919605015));
#220043=CARTESIAN_POINT('Ctrl Pts',(-37.8595407315309,62.5964957764151,
72.040048310785));
#220044=CARTESIAN_POINT('Ctrl Pts',(-37.9572081178209,62.9845925876825,
76.2102600797003));
#220045=CARTESIAN_POINT('Ctrl Pts',(-38.0548755041109,64.734694589886,80.0153149192114));
#220046=CARTESIAN_POINT('Ctrl Pts',(-38.1525428904009,67.648394717053,83.0238940611853));
#220047=CARTESIAN_POINT('Ctrl Pts',(-38.2502102766909,71.39550623112,84.8949575070187));
#220048=CARTESIAN_POINT('Ctrl Pts',(-38.3153218675509,74.1657861357241,
85.2426041509183));
#220049=CARTESIAN_POINT('Ctrl Pts',(-38.3478776629809,75.5406900979627,
85.1816337132427));
#220050=CARTESIAN_POINT('Ctrl Pts',(-32.3212930507009,70.5807652625035,
62.0755168906179));
#220051=CARTESIAN_POINT('Ctrl Pts',(-32.3538488461309,69.3501285260828,
62.5738479625974));
#220052=CARTESIAN_POINT('Ctrl Pts',(-32.4189604369909,67.0593648594363,
63.9906830308551));
#220053=CARTESIAN_POINT('Ctrl Pts',(-32.5166278232809,64.5230776800325,
67.1360227552467));
#220054=CARTESIAN_POINT('Ctrl Pts',(-32.6142952095709,63.1744626819709,
70.9447840322971));
#220055=CARTESIAN_POINT('Ctrl Pts',(-32.7119625958609,63.1663071209847,
74.9852609507785));
#220056=CARTESIAN_POINT('Ctrl Pts',(-32.8096299821509,64.4995580412843,
78.7994383430527));
#220057=CARTESIAN_POINT('Ctrl Pts',(-32.9072973684309,67.0230794732875,
81.9549646900448));
#220058=CARTESIAN_POINT('Ctrl Pts',(-33.0049647547209,70.4508206617514,
84.0941463918273));
#220059=CARTESIAN_POINT('Ctrl Pts',(-33.1026321410109,74.3942314659886,
84.9744978657157));
#220060=CARTESIAN_POINT('Ctrl Pts',(-33.2002995273009,78.4063088519184,
84.4962273102157));
#220061=CARTESIAN_POINT('Ctrl Pts',(-33.2979669135909,82.0322659755195,
82.7135488322343));
#220062=CARTESIAN_POINT('Ctrl Pts',(-33.3956342998809,84.8610844810572,
79.828536961178));
#220063=CARTESIAN_POINT('Ctrl Pts',(-33.4933016861709,86.5721052093522,
76.1682206227876));
#220064=CARTESIAN_POINT('Ctrl Pts',(-33.5909690724609,86.9713763527652,
72.1475129506798));
#220065=CARTESIAN_POINT('Ctrl Pts',(-33.6886364587509,86.0136387515289,
68.2221790390765));
#220066=CARTESIAN_POINT('Ctrl Pts',(-33.7863038450409,83.8074562217176,
64.8371729422474));
#220067=CARTESIAN_POINT('Ctrl Pts',(-33.8839712313309,80.602909363651,62.3762001539254));
#220068=CARTESIAN_POINT('Ctrl Pts',(-33.9816386176209,76.7632478138661,
61.1182228832598));
#220069=CARTESIAN_POINT('Ctrl Pts',(-34.0793060039109,72.723714283464,61.2058384479297));
#220070=CARTESIAN_POINT('Ctrl Pts',(-34.1769733902009,68.9422078613542,
62.6291152340622));
#220071=CARTESIAN_POINT('Ctrl Pts',(-34.2746407764909,65.8473791163074,
65.226718488844));
#220072=CARTESIAN_POINT('Ctrl Pts',(-34.3723081627809,63.7900406488467,
68.7041983321679));
#220073=CARTESIAN_POINT('Ctrl Pts',(-34.4699755490709,63.0034009229566,
72.66736695993));
#220074=CARTESIAN_POINT('Ctrl Pts',(-34.5676429353609,63.5766290496323,
76.666981584516));
#220075=CARTESIAN_POINT('Ctrl Pts',(-34.6653103216509,65.4447470716599,
80.2496681025062));
#220076=CARTESIAN_POINT('Ctrl Pts',(-34.7629777079409,68.3959955039791,
83.0093130653877));
#220077=CARTESIAN_POINT('Ctrl Pts',(-34.8606450942309,72.0958372130047,
84.6330984448554));
#220078=CARTESIAN_POINT('Ctrl Pts',(-34.9583124805209,76.1248786883367,
84.9369609474145));
#220079=CARTESIAN_POINT('Ctrl Pts',(-35.0559798668109,80.0264101621715,
83.8864564071508));
#220080=CARTESIAN_POINT('Ctrl Pts',(-35.1536472531009,83.3581756923815,
81.6006641851604));
#220081=CARTESIAN_POINT('Ctrl Pts',(-35.2513146393909,85.7425048402344,
78.338688994402));
#220082=CARTESIAN_POINT('Ctrl Pts',(-35.3489820256809,86.909123294031,74.4702902282876));
#220083=CARTESIAN_POINT('Ctrl Pts',(-35.4466494119709,86.7257896642541,
70.4339680891861));
#220084=CARTESIAN_POINT('Ctrl Pts',(-35.5443167982609,85.2132856330985,
66.6872576405197));
#220085=CARTESIAN_POINT('Ctrl Pts',(-35.6419841845509,82.5430602583853,
63.6548651727437));
#220086=CARTESIAN_POINT('Ctrl Pts',(-35.7396515708509,79.0177954604591,
61.6805258566955));
#220087=CARTESIAN_POINT('Ctrl Pts',(-35.8373189571409,75.0370956805214,
60.9880398334549));
#220088=CARTESIAN_POINT('Ctrl Pts',(-35.9349863434309,71.0521909402342,
61.6559034731574));
#220089=CARTESIAN_POINT('Ctrl Pts',(-36.0326537297209,67.5147879122209,
63.6084114623352));
#220090=CARTESIAN_POINT('Ctrl Pts',(-36.1303211160109,64.8258669600518,
66.6242383378935));
#220091=CARTESIAN_POINT('Ctrl Pts',(-36.2279885023009,63.2902292308876,
70.3615267125221));
#220092=CARTESIAN_POINT('Ctrl Pts',(-36.3256558885909,63.0819460901088,
74.3966383297692));
#220093=CARTESIAN_POINT('Ctrl Pts',(-36.4233232748809,64.2246273579156,
78.2721753442413));
#220094=CARTESIAN_POINT('Ctrl Pts',(-36.5209906611709,66.5887450312666,
81.5488284013896));
#220095=CARTESIAN_POINT('Ctrl Pts',(-36.6186580474609,69.9063158589901,
83.8551743063605));
#220096=CARTESIAN_POINT('Ctrl Pts',(-36.7163254337509,73.8012784349875,
84.9297784948445));
#220097=CARTESIAN_POINT('Ctrl Pts',(-36.8139928200409,77.8321214309277,
84.6508298034519));
#220098=CARTESIAN_POINT('Ctrl Pts',(-36.9116602063309,81.5419308686238,
83.0499483068092));
#220099=CARTESIAN_POINT('Ctrl Pts',(-37.0093275926209,84.510183351323,80.3086010414542));
#220100=CARTESIAN_POINT('Ctrl Pts',(-37.1069949789109,86.4004142607001,
76.7375319102928));
#220101=CARTESIAN_POINT('Ctrl Pts',(-37.2046623652009,86.9983575175985,
72.7415374793883));
#220102=CARTESIAN_POINT('Ctrl Pts',(-37.3023297514909,86.2362335948903,
68.7735814871058));
#220103=CARTESIAN_POINT('Ctrl Pts',(-37.3999971377809,84.2004326282222,
65.2834493901101));
#220104=CARTESIAN_POINT('Ctrl Pts',(-37.4976645240709,81.1217217102652,
62.6667631817018));
#220105=CARTESIAN_POINT('Ctrl Pts',(-37.5953319103609,77.3490864135083,
61.220135879683));
#220106=CARTESIAN_POINT('Ctrl Pts',(-37.6929992966509,73.3101717276327,
61.1075491215587));
#220107=CARTESIAN_POINT('Ctrl Pts',(-37.7906666829409,69.4628065837551,
62.3417651174235));
#220108=CARTESIAN_POINT('Ctrl Pts',(-37.8883340692309,66.2431069632321,
64.7828799942742));
#220109=CARTESIAN_POINT('Ctrl Pts',(-37.9860014555209,64.0160400101624,
68.1541825310843));
#220110=CARTESIAN_POINT('Ctrl Pts',(-38.0836688418109,63.0340541352225,
72.0735205728459));
#220111=CARTESIAN_POINT('Ctrl Pts',(-38.1813362281009,63.4084600571474,
76.0966198012584));
#220112=CARTESIAN_POINT('Ctrl Pts',(-38.2790036143909,65.0968237194401,
79.7674437395072));
#220113=CARTESIAN_POINT('Ctrl Pts',(-38.3766710006809,67.907737261243,82.669889249567));
#220114=CARTESIAN_POINT('Ctrl Pts',(-38.4743383869709,71.5226619404589,
84.4749471992292));
#220115=CARTESIAN_POINT('Ctrl Pts',(-38.5394499778309,74.195214694201,84.8103299141412));
#220116=CARTESIAN_POINT('Ctrl Pts',(-38.5720057732609,75.5216161759791,
84.7515103303026));
#220117=CARTESIAN_POINT('',(-37.8135594354587,70.2739654383489,85.0994033094111));
#220118=CARTESIAN_POINT('Ctrl Pts',(-37.8135412566021,70.2734991756117,
85.0992154535004));
#220119=CARTESIAN_POINT('Ctrl Pts',(-37.914194608833,70.3438095733745,84.9191033777816));
#220120=CARTESIAN_POINT('Ctrl Pts',(-38.0148481000433,70.4141195120353,
84.738990837336));
#220121=CARTESIAN_POINT('Ctrl Pts',(-38.2164814619069,70.5549662664303,
84.3781812921325));
#220122=CARTESIAN_POINT('Ctrl Pts',(-38.3174616206795,70.625503279821,84.1974837704057));
#220123=CARTESIAN_POINT('Ctrl Pts',(-38.4184416307608,70.6960396334767,
84.0167862995286));
#220124=CARTESIAN_POINT('',(-31.8032830015106,65.6643078538855,63.942145982536));
#220125=CARTESIAN_POINT('Ctrl Pts',(-36.4473639743914,87.0149197055719,
77.9529305295058));
#220126=CARTESIAN_POINT('Ctrl Pts',(-36.4543242139158,87.1337046269196,
77.665424594093));
#220127=CARTESIAN_POINT('Ctrl Pts',(-36.4612901076495,87.2421954633006,
77.3735933081721));
#220128=CARTESIAN_POINT('Ctrl Pts',(-36.4851178847728,87.5794817571952,
76.3557248300557));
#220129=CARTESIAN_POINT('Ctrl Pts',(-36.5017295071393,87.7549428334773,
75.6138431779786));
#220130=CARTESIAN_POINT('Ctrl Pts',(-36.5357271191037,87.9752973710121,
74.099549431073));
#220131=CARTESIAN_POINT('Ctrl Pts',(-36.5530472978884,88.0182807436117,
73.3298801212865));
#220132=CARTESIAN_POINT('Ctrl Pts',(-36.5916188607997,87.9609665594104,
71.58976080149));
#220133=CARTESIAN_POINT('Ctrl Pts',(-36.6128788214405,87.8201909513787,
70.6252211721631));
#220134=CARTESIAN_POINT('Ctrl Pts',(-36.6439275780304,87.4672144669563,
69.2817701998118));
#220135=CARTESIAN_POINT('Ctrl Pts',(-36.6532862550123,87.3417882891993,
68.8834745078011));
#220136=CARTESIAN_POINT('Ctrl Pts',(-36.6809277077594,86.9117980094235,
67.7171882447898));
#220137=CARTESIAN_POINT('Ctrl Pts',(-36.6989352535155,86.5530137947842,
66.9714444563634));
#220138=CARTESIAN_POINT('Ctrl Pts',(-36.7364462999144,85.680867030899,65.5283614602584));
#220139=CARTESIAN_POINT('Ctrl Pts',(-36.7557849234076,85.1637830132544,
64.8379432567854));
#220140=CARTESIAN_POINT('Ctrl Pts',(-36.7839680363835,84.300566023742,63.8964053745483));
#220141=CARTESIAN_POINT('Ctrl Pts',(-36.79313620763,84.0042231131444,63.6028486954881));
#220142=CARTESIAN_POINT('Ctrl Pts',(-36.8208522435962,83.0733987976403,
62.7654993629996));
#220143=CARTESIAN_POINT('Ctrl Pts',(-36.8396187225315,82.4001330837469,
62.2680924422089));
#220144=CARTESIAN_POINT('Ctrl Pts',(-36.8761199441608,80.991966806184,61.4239852534392));
#220145=CARTESIAN_POINT('Ctrl Pts',(-36.8937173024056,80.2630028772171,
61.0745500786368));
#220146=CARTESIAN_POINT('Ctrl Pts',(-36.9307904571172,78.6992531278834,
60.4966544983454));
#220147=CARTESIAN_POINT('Ctrl Pts',(-36.9501392419649,77.8645104056248,
60.2792475243341));
#220148=CARTESIAN_POINT('Ctrl Pts',(-36.9783085147289,76.6035404801462,
60.0814635701045));
#220149=CARTESIAN_POINT('Ctrl Pts',(-36.9874532249925,76.1897955949716,
60.0367710386153));
#220150=CARTESIAN_POINT('Ctrl Pts',(-37.0151750161543,74.9392545890132,
59.9621232756562));
#220151=CARTESIAN_POINT('Ctrl Pts',(-37.0339691243248,74.1010274283916,
59.9930378008006));
#220152=CARTESIAN_POINT('Ctrl Pts',(-37.0719391167667,72.4094517773143,
60.2199522860539));
#220153=CARTESIAN_POINT('Ctrl Pts',(-37.0908982866283,71.561074100533,60.4218495763451));
#220154=CARTESIAN_POINT('Ctrl Pts',(-37.1294214814689,69.9265064525839,
60.9889023507669));
#220155=CARTESIAN_POINT('Ctrl Pts',(-37.1487274281533,69.1437612082903,
61.3508266538269));
#220156=CARTESIAN_POINT('Ctrl Pts',(-37.1769356443394,68.0416056556518,
61.9999770084488));
#220157=CARTESIAN_POINT('Ctrl Pts',(-37.1861529674104,67.6911753126028,
62.2298685958544));
#220158=CARTESIAN_POINT('Ctrl Pts',(-37.214477195763,66.6574182380909,62.9818891792332));
#220159=CARTESIAN_POINT('Ctrl Pts',(-37.2338260991683,66.0142366260856,
63.5551852269181));
#220160=CARTESIAN_POINT('Ctrl Pts',(-37.2732001920621,64.8116847703535,
64.8624684866943));
#220161=CARTESIAN_POINT('Ctrl Pts',(-37.2932388578807,64.264126164404,65.6009596366178));
#220162=CARTESIAN_POINT('Ctrl Pts',(-37.3230050221112,63.5874803930889,
66.7496754353562));
#220163=CARTESIAN_POINT('Ctrl Pts',(-37.3323422503652,63.3934987902411,
67.1184103729201));
#220164=CARTESIAN_POINT('Ctrl Pts',(-37.3686321206999,62.7058503688647,
68.5933925755802));
#220165=CARTESIAN_POINT('Ctrl Pts',(-37.3949739782692,62.3500174026053,
69.7571023938164));
#220166=CARTESIAN_POINT('Ctrl Pts',(-37.4314600837915,62.0946346744905,
71.3678326654396));
#220167=CARTESIAN_POINT('Ctrl Pts',(-37.4408579427422,62.0490146141995,
71.7854526511129));
#220168=CARTESIAN_POINT('Ctrl Pts',(-37.4619584631861,61.9915130619058,
72.736770787313));
#220169=CARTESIAN_POINT('Ctrl Pts',(-37.4736509812777,61.9921173651715,
73.270469430752));
#220170=CARTESIAN_POINT('Ctrl Pts',(-37.5039566961825,62.077828664538,74.6370913696173));
#220171=CARTESIAN_POINT('Ctrl Pts',(-37.5227388742895,62.2105472640685,
75.464564129881));
#220172=CARTESIAN_POINT('Ctrl Pts',(-37.5600406728055,62.6343126277398,
77.0873268194587));
#220173=CARTESIAN_POINT('Ctrl Pts',(-37.5783792083311,62.9252991418412,
77.8785743582914));
#220174=CARTESIAN_POINT('Ctrl Pts',(-37.6162434269404,63.6644474380039,
79.4111631043095));
#220175=CARTESIAN_POINT('Ctrl Pts',(-37.6355728942984,64.1142489189937,
80.147156340735));
#220176=CARTESIAN_POINT('Ctrl Pts',(-37.6675712385135,64.9895008496932,
81.3038198263665));
#220177=CARTESIAN_POINT('Ctrl Pts',(-37.6805474167461,65.3771686591776,
81.7495558744315));
#220178=CARTESIAN_POINT('Ctrl Pts',(-37.7134056908055,66.420115336078,82.7956509277219));
#220179=CARTESIAN_POINT('Ctrl Pts',(-37.7333333337727,67.109129135656,83.3581304716378));
#220180=CARTESIAN_POINT('Ctrl Pts',(-37.7629134085071,68.229296810036,84.0958152528438));
#220181=CARTESIAN_POINT('Ctrl Pts',(-37.7729023062673,68.6213877917966,
84.3255348210361));
#220182=CARTESIAN_POINT('Ctrl Pts',(-37.7931080409524,69.4308381406786,
84.7444656957888));
#220183=CARTESIAN_POINT('Ctrl Pts',(-37.8033123696457,69.8477910971911,
84.933087944667));
#220184=CARTESIAN_POINT('Ctrl Pts',(-37.8135449901797,70.2738124000625,
85.099345644302));
#220185=CARTESIAN_POINT('Ctrl Pts',(-37.7678684231509,69.7754278285013,
84.9428528583425));
#220186=CARTESIAN_POINT('Ctrl Pts',(-37.8179054464809,71.812510839228,85.9277583999696));
#220187=CARTESIAN_POINT('Ctrl Pts',(-37.9179794931409,76.4517787269631,
86.8316803850283));
#220188=CARTESIAN_POINT('Ctrl Pts',(-38.0680905631309,83.2977536927465,
84.5014189876434));
#220189=CARTESIAN_POINT('Ctrl Pts',(-38.2182016331209,88.1688027886436,
78.9684584806007));
#220190=CARTESIAN_POINT('Ctrl Pts',(-38.3182756797809,89.1697068583504,
74.0638248418015));
#220191=CARTESIAN_POINT('Ctrl Pts',(-38.3683127031109,89.0196937392787,
71.6256255348517));
#220192=CARTESIAN_POINT('Ctrl Pts',(-37.9919965334309,69.9478523514013,
84.5483408522442));
#220193=CARTESIAN_POINT('Ctrl Pts',(-38.0420335567609,71.9165608444039,
85.5033627821869));
#220194=CARTESIAN_POINT('Ctrl Pts',(-38.1421076034109,76.4032882596886,
86.3839207906894));
#220195=CARTESIAN_POINT('Ctrl Pts',(-38.2922186734109,83.0331917990117,
84.1369185523978));
#220196=CARTESIAN_POINT('Ctrl Pts',(-38.4423297434009,87.7581170900009,
78.7835876157209));
#220197=CARTESIAN_POINT('Ctrl Pts',(-38.5424037900609,88.7339600476783,
74.0312248270542));
#220198=CARTESIAN_POINT('Ctrl Pts',(-38.5924408133809,88.5911688293687,
71.6672949557471));
#220199=CARTESIAN_POINT('Ctrl Pts',(-38.2161246437009,70.1202768743014,
84.1538288461459));
#220200=CARTESIAN_POINT('Ctrl Pts',(-38.2661616670309,72.0206108495836,
85.078967164395));
#220201=CARTESIAN_POINT('Ctrl Pts',(-38.3662357136909,76.354797792418,85.9361611963414));
#220202=CARTESIAN_POINT('Ctrl Pts',(-38.5163467836809,82.7686299052744,
83.7724181171587));
#220203=CARTESIAN_POINT('Ctrl Pts',(-38.6664578536809,87.347431391376,78.5987167508506));
#220204=CARTESIAN_POINT('Ctrl Pts',(-38.7665319003309,88.2982132370069,
73.9986248123051));
#220205=CARTESIAN_POINT('Ctrl Pts',(-38.8165689236609,88.1626439194586,
71.7089643766425));
#220206=CARTESIAN_POINT('Ctrl Pts',(-38.4402527539809,70.2927013972014,
83.7593168400476));
#220207=CARTESIAN_POINT('Ctrl Pts',(-38.4902897773109,72.1246608547595,
84.6545715466124));
#220208=CARTESIAN_POINT('Ctrl Pts',(-38.5903638239709,76.3063073251473,
85.4884016019933));
#220209=CARTESIAN_POINT('Ctrl Pts',(-38.7404748939609,82.50406801154,83.4079176819123));
#220210=CARTESIAN_POINT('Ctrl Pts',(-38.8905859639509,86.9367456927425,
78.4138458859747));
#220211=CARTESIAN_POINT('Ctrl Pts',(-38.9906600106109,87.8624664263344,
73.9660247975587));
#220212=CARTESIAN_POINT('Ctrl Pts',(-39.0406970339409,87.7341190095482,
71.7506337975389));
#220213=CARTESIAN_POINT('Ctrl Pts',(-38.9114901698969,87.9789324622055,
72.2490839199139));
#220214=CARTESIAN_POINT('Ctrl Pts',(-38.9253796493603,87.9522946700216,
72.2506022870319));
#220215=CARTESIAN_POINT('Ctrl Pts',(-38.9392691288105,87.9256568778308,
72.2521206541503));
#220216=CARTESIAN_POINT('Ctrl Pts',(-38.9670676750248,87.8723437280596,
72.2551595296326));
#220217=CARTESIAN_POINT('Ctrl Pts',(-38.9809767417889,87.8456683704791,
72.2566800379965));
#220218=CARTESIAN_POINT('Ctrl Pts',(-38.9948858085393,87.8189930128915,
72.2582005463608));
#220219=CARTESIAN_POINT('Ctrl Pts',(-38.6651607695591,87.0149202732382,
77.9529291555314));
#220220=CARTESIAN_POINT('Ctrl Pts',(-38.61247162501,86.5348402930432,79.1149107179875));
#220221=CARTESIAN_POINT('Ctrl Pts',(-38.5579303068348,85.888739014892,80.2010992341742));
#220222=CARTESIAN_POINT('Ctrl Pts',(-38.4509479952484,84.2940740611299,
82.1673583393616));
#220223=CARTESIAN_POINT('Ctrl Pts',(-38.3992043907891,83.350151501424,83.0337413163218));
#220224=CARTESIAN_POINT('Ctrl Pts',(-38.3094997884851,81.6049979618063,
84.2169638927091));
#220225=CARTESIAN_POINT('Ctrl Pts',(-38.2735339351583,80.8712054740595,
84.617501870553));
#220226=CARTESIAN_POINT('Ctrl Pts',(-38.166422504845,78.5525910761281,85.6073284218056));
#220227=CARTESIAN_POINT('Ctrl Pts',(-38.0982006061265,76.8869101288329,
85.9613759922045));
#220228=CARTESIAN_POINT('Ctrl Pts',(-37.9903150495058,74.367121750432,86.0001753956269));
#220229=CARTESIAN_POINT('Ctrl Pts',(-37.9546993734579,73.5347687972715,
85.9328938291296));
#220230=CARTESIAN_POINT('Ctrl Pts',(-37.8839532152002,71.8806570845743,
85.6374986271245));
#220231=CARTESIAN_POINT('Ctrl Pts',(-37.8490190852945,71.0632872725336,
85.4074198623627));
#220232=CARTESIAN_POINT('Ctrl Pts',(-37.8135657720877,70.2741279641925,
85.0994687906042));
#220233=CARTESIAN_POINT('Origin',(-39.1448867524609,88.9773118829169,72.1921758070624));
#220234=CARTESIAN_POINT('Ctrl Pts',(-39.2948856686008,87.8189932824241,
72.2582005309974));
#220235=CARTESIAN_POINT('Ctrl Pts',(-39.3087857943346,87.8456514869417,
72.2566810003664));
#220236=CARTESIAN_POINT('Ctrl Pts',(-39.3226859200676,87.8723096914597,
72.2551614697354));
#220237=CARTESIAN_POINT('Ctrl Pts',(-39.3504844252439,87.925622751396,72.2521225993737));
#220238=CARTESIAN_POINT('Ctrl Pts',(-39.3643828046871,87.9522776068144,
72.250603259643));
#220239=CARTESIAN_POINT('Ctrl Pts',(-39.3782811841296,87.9789324622331,
72.2490839199123));
#220240=CARTESIAN_POINT('Ctrl Pts',(-38.6717262017909,70.2927013972015,
83.7593168400477));
#220241=CARTESIAN_POINT('Ctrl Pts',(-38.7217632251209,72.1246608547595,
84.6545715466124));
#220242=CARTESIAN_POINT('Ctrl Pts',(-38.8218372717809,76.3063073251473,
85.4884016019933));
#220243=CARTESIAN_POINT('Ctrl Pts',(-38.9719483417709,82.50406801154,83.4079176819123));
#220244=CARTESIAN_POINT('Ctrl Pts',(-39.1220594117609,86.9367456927426,
78.4138458859746));
#220245=CARTESIAN_POINT('Ctrl Pts',(-39.2221334584209,87.8624664263348,
73.9660247975578));
#220246=CARTESIAN_POINT('Ctrl Pts',(-39.2721704817509,87.7341190095482,
71.7506337975389));
#220247=CARTESIAN_POINT('Ctrl Pts',(-38.8958543120709,70.1202768743015,
84.153828846146));
#220248=CARTESIAN_POINT('Ctrl Pts',(-38.9458913354009,72.0206108495836,
85.078967164395));
#220249=CARTESIAN_POINT('Ctrl Pts',(-39.0459653820509,76.354797792418,85.9361611963414));
#220250=CARTESIAN_POINT('Ctrl Pts',(-39.1960764520509,82.7686299052747,
83.7724181171578));
#220251=CARTESIAN_POINT('Ctrl Pts',(-39.3461875220409,87.347431391376,78.5987167508506));
#220252=CARTESIAN_POINT('Ctrl Pts',(-39.4462615687009,88.2982132370069,
73.9986248123051));
#220253=CARTESIAN_POINT('Ctrl Pts',(-39.4962985920209,88.1626439194586,
71.7089643766425));
#220254=CARTESIAN_POINT('Ctrl Pts',(-39.1199824223409,69.9478523514015,
84.5483408522443));
#220255=CARTESIAN_POINT('Ctrl Pts',(-39.1700194456709,71.9165608444039,
85.5033627821869));
#220256=CARTESIAN_POINT('Ctrl Pts',(-39.2700934923309,76.4032882596886,
86.3839207906894));
#220257=CARTESIAN_POINT('Ctrl Pts',(-39.4202045623209,83.0331917990117,
84.1369185523978));
#220258=CARTESIAN_POINT('Ctrl Pts',(-39.5703156323209,87.758117090001,78.7835876157208));
#220259=CARTESIAN_POINT('Ctrl Pts',(-39.6703896789709,88.7339600476783,
74.0312248270542));
#220260=CARTESIAN_POINT('Ctrl Pts',(-39.7204267023009,88.5911688293687,
71.6672949557471));
#220261=CARTESIAN_POINT('Ctrl Pts',(-39.3441105326209,69.7754278285015,
84.9428528583426));
#220262=CARTESIAN_POINT('Ctrl Pts',(-39.3941475559509,71.812510839228,85.9277583999696));
#220263=CARTESIAN_POINT('Ctrl Pts',(-39.4942216026109,76.4517787269631,
86.8316803850283));
#220264=CARTESIAN_POINT('Ctrl Pts',(-39.6443326726009,83.2977536927465,
84.5014189876434));
#220265=CARTESIAN_POINT('Ctrl Pts',(-39.7944437425909,88.1688027886436,
78.9684584806006));
#220266=CARTESIAN_POINT('Ctrl Pts',(-39.8945177892509,89.1697068583508,
74.0638248418006));
#220267=CARTESIAN_POINT('Ctrl Pts',(-39.9445548125809,89.0196937392787,
71.6256255348517));
#220268=CARTESIAN_POINT('Ctrl Pts',(-38.7166027955229,70.6961178052446,
84.016824453434));
#220269=CARTESIAN_POINT('Ctrl Pts',(-38.8175043475842,70.6256382812911,
84.1973835573518));
#220270=CARTESIAN_POINT('Ctrl Pts',(-38.9184059185855,70.5551581924261,
84.3779424805074));
#220271=CARTESIAN_POINT('Ctrl Pts',(-39.120038274912,70.4143162025418,84.7387542827717));
#220272=CARTESIAN_POINT('Ctrl Pts',(-39.2207694758059,70.3439540131132,
84.9190079062487));
#220273=CARTESIAN_POINT('Ctrl Pts',(-39.3215005357773,70.2735913682008,
85.0992610619776));
#220274=CARTESIAN_POINT('Ctrl Pts',(-32.5527664985109,70.5807652625035,
62.0755168906179));
#220275=CARTESIAN_POINT('Ctrl Pts',(-32.5853222939409,69.3501285260828,
62.5738479625974));
#220276=CARTESIAN_POINT('Ctrl Pts',(-32.6504338848009,67.0593648594363,
63.9906830308551));
#220277=CARTESIAN_POINT('Ctrl Pts',(-32.7481012710909,64.5230776800325,
67.1360227552467));
#220278=CARTESIAN_POINT('Ctrl Pts',(-32.8457686573809,63.1744626819709,
70.9447840322971));
#220279=CARTESIAN_POINT('Ctrl Pts',(-32.9434360436709,63.1663071209847,
74.9852609507785));
#220280=CARTESIAN_POINT('Ctrl Pts',(-33.0411034299609,64.4995580412843,
78.7994383430527));
#220281=CARTESIAN_POINT('Ctrl Pts',(-33.1387708162509,67.0230794732875,
81.9549646900448));
#220282=CARTESIAN_POINT('Ctrl Pts',(-33.2364382025409,70.4508206617514,
84.0941463918273));
#220283=CARTESIAN_POINT('Ctrl Pts',(-33.3341055888209,74.3942314659886,
84.9744978657157));
#220284=CARTESIAN_POINT('Ctrl Pts',(-33.4317729751109,78.4063088519184,
84.4962273102157));
#220285=CARTESIAN_POINT('Ctrl Pts',(-33.5294403614009,82.0322659755195,
82.7135488322343));
#220286=CARTESIAN_POINT('Ctrl Pts',(-33.6271077476909,84.8610844810572,
79.828536961178));
#220287=CARTESIAN_POINT('Ctrl Pts',(-33.7247751339809,86.5721052093522,
76.1682206227876));
#220288=CARTESIAN_POINT('Ctrl Pts',(-33.8224425202709,86.9713763527652,
72.1475129506798));
#220289=CARTESIAN_POINT('Ctrl Pts',(-33.9201099065609,86.0136387515289,
68.2221790390765));
#220290=CARTESIAN_POINT('Ctrl Pts',(-34.0177772928509,83.8074562217176,
64.8371729422474));
#220291=CARTESIAN_POINT('Ctrl Pts',(-34.1154446791409,80.602909363651,62.3762001539254));
#220292=CARTESIAN_POINT('Ctrl Pts',(-34.2131120654309,76.7632478138661,
61.1182228832598));
#220293=CARTESIAN_POINT('Ctrl Pts',(-34.3107794517209,72.723714283464,61.2058384479297));
#220294=CARTESIAN_POINT('Ctrl Pts',(-34.4084468380109,68.9422078613546,
62.6291152340613));
#220295=CARTESIAN_POINT('Ctrl Pts',(-34.5061142243009,65.8473791163074,
65.226718488844));
#220296=CARTESIAN_POINT('Ctrl Pts',(-34.6037816105909,63.7900406488467,
68.7041983321679));
#220297=CARTESIAN_POINT('Ctrl Pts',(-34.7014489968809,63.0034009229566,
72.66736695993));
#220298=CARTESIAN_POINT('Ctrl Pts',(-34.7991163831709,63.5766290496323,
76.666981584516));
#220299=CARTESIAN_POINT('Ctrl Pts',(-34.8967837694509,65.4447470716599,
80.2496681025062));
#220300=CARTESIAN_POINT('Ctrl Pts',(-34.9944511557409,68.3959955039791,
83.0093130653877));
#220301=CARTESIAN_POINT('Ctrl Pts',(-35.0921185420309,72.0958372130047,
84.6330984448554));
#220302=CARTESIAN_POINT('Ctrl Pts',(-35.1897859283209,76.1248786883367,
84.9369609474145));
#220303=CARTESIAN_POINT('Ctrl Pts',(-35.2874533146109,80.0264101621715,
83.8864564071508));
#220304=CARTESIAN_POINT('Ctrl Pts',(-35.3851207009009,83.3581756923815,
81.6006641851604));
#220305=CARTESIAN_POINT('Ctrl Pts',(-35.4827880871909,85.7425048402343,
78.3386889944021));
#220306=CARTESIAN_POINT('Ctrl Pts',(-35.5804554734809,86.909123294031,74.4702902282876));
#220307=CARTESIAN_POINT('Ctrl Pts',(-35.6781228597709,86.7257896642541,
70.4339680891861));
#220308=CARTESIAN_POINT('Ctrl Pts',(-35.7757902460609,85.2132856330985,
66.6872576405197));
#220309=CARTESIAN_POINT('Ctrl Pts',(-35.8734576323509,82.5430602583853,
63.6548651727437));
#220310=CARTESIAN_POINT('Ctrl Pts',(-35.9711250186409,79.017795460459,61.6805258566955));
#220311=CARTESIAN_POINT('Ctrl Pts',(-36.0687924049309,75.0370956805214,
60.9880398334549));
#220312=CARTESIAN_POINT('Ctrl Pts',(-36.1664597912209,71.0521909402342,
61.6559034731574));
#220313=CARTESIAN_POINT('Ctrl Pts',(-36.2641271775109,67.5147879122209,
63.6084114623352));
#220314=CARTESIAN_POINT('Ctrl Pts',(-36.3617945638009,64.8258669600518,
66.6242383378935));
#220315=CARTESIAN_POINT('Ctrl Pts',(-36.4594619500909,63.2902292308876,
70.3615267125221));
#220316=CARTESIAN_POINT('Ctrl Pts',(-36.5571293363809,63.0819460901088,
74.3966383297692));
#220317=CARTESIAN_POINT('Ctrl Pts',(-36.6547967226709,64.2246273579156,
78.2721753442413));
#220318=CARTESIAN_POINT('Ctrl Pts',(-36.7524641089609,66.5887450312666,
81.5488284013896));
#220319=CARTESIAN_POINT('Ctrl Pts',(-36.8501314952509,69.9063158589901,
83.8551743063605));
#220320=CARTESIAN_POINT('Ctrl Pts',(-36.9477988815409,73.8012784349875,
84.9297784948445));
#220321=CARTESIAN_POINT('Ctrl Pts',(-37.0454662678409,77.8321214309277,
84.6508298034519));
#220322=CARTESIAN_POINT('Ctrl Pts',(-37.1431336541309,81.5419308686238,
83.0499483068092));
#220323=CARTESIAN_POINT('Ctrl Pts',(-37.2408010404209,84.510183351323,80.3086010414542));
#220324=CARTESIAN_POINT('Ctrl Pts',(-37.3384684267109,86.4004142607001,
76.7375319102928));
#220325=CARTESIAN_POINT('Ctrl Pts',(-37.4361358130009,86.9983575175985,
72.7415374793883));
#220326=CARTESIAN_POINT('Ctrl Pts',(-37.5338031992909,86.2362335948903,
68.7735814871058));
#220327=CARTESIAN_POINT('Ctrl Pts',(-37.6314705855809,84.2004326282222,
65.2834493901101));
#220328=CARTESIAN_POINT('Ctrl Pts',(-37.7291379718709,81.1217217102652,
62.6667631817018));
#220329=CARTESIAN_POINT('Ctrl Pts',(-37.8268053581609,77.3490864135083,
61.220135879683));
#220330=CARTESIAN_POINT('Ctrl Pts',(-37.9244727444509,73.3101717276327,
61.1075491215587));
#220331=CARTESIAN_POINT('Ctrl Pts',(-38.0221401307409,69.4628065837551,
62.3417651174235));
#220332=CARTESIAN_POINT('Ctrl Pts',(-38.1198075170309,66.2431069632321,
64.7828799942742));
#220333=CARTESIAN_POINT('Ctrl Pts',(-38.2174749033309,64.0160400101624,
68.1541825310843));
#220334=CARTESIAN_POINT('Ctrl Pts',(-38.3151422896209,63.0340541352225,
72.0735205728459));
#220335=CARTESIAN_POINT('Ctrl Pts',(-38.4128096759109,63.4084600571474,
76.0966198012584));
#220336=CARTESIAN_POINT('Ctrl Pts',(-38.5104770622009,65.0968237194401,
79.7674437395072));
#220337=CARTESIAN_POINT('Ctrl Pts',(-38.6081444484909,67.907737261243,82.669889249567));
#220338=CARTESIAN_POINT('Ctrl Pts',(-38.7058118347809,71.5226619404589,
84.4749471992292));
#220339=CARTESIAN_POINT('Ctrl Pts',(-38.7709234256409,74.195214694201,84.8103299141412));
#220340=CARTESIAN_POINT('Ctrl Pts',(-38.8034792210709,75.5216161759791,
84.7515103303026));
#220341=CARTESIAN_POINT('Ctrl Pts',(-32.7768946087909,70.4191672475379,
61.6764479484404));
#220342=CARTESIAN_POINT('Ctrl Pts',(-32.8094504042209,69.1435298570313,
62.1930014767527));
#220343=CARTESIAN_POINT('Ctrl Pts',(-32.8745619950809,66.7689999088247,
63.6616459075254));
#220344=CARTESIAN_POINT('Ctrl Pts',(-32.9722293813709,64.1399683974443,
66.9220011687802));
#220345=CARTESIAN_POINT('Ctrl Pts',(-33.0698967676509,62.7420386379846,
70.8700372973402));
#220346=CARTESIAN_POINT('Ctrl Pts',(-33.1675641539409,62.7335848528663,
75.0582622057643));
#220347=CARTESIAN_POINT('Ctrl Pts',(-33.2652315402309,64.1155887168238,
79.0119125004583));
#220348=CARTESIAN_POINT('Ctrl Pts',(-33.3628989265209,66.7313876761263,
82.2828268782175));
#220349=CARTESIAN_POINT('Ctrl Pts',(-33.4605663128109,70.2844709667367,
84.500231968704));
#220350=CARTESIAN_POINT('Ctrl Pts',(-33.5582336991009,74.3720803474283,
85.4127752267091));
#220351=CARTESIAN_POINT('Ctrl Pts',(-33.6559010853909,78.5308672385013,
84.9170157671447));
#220352=CARTESIAN_POINT('Ctrl Pts',(-33.7535684716809,82.2894146199872,
83.0691501424084));
#220353=CARTESIAN_POINT('Ctrl Pts',(-33.8512358579709,85.2216744411351,
80.0786421347599));
#220354=CARTESIAN_POINT('Ctrl Pts',(-33.9489032442609,86.9952620095349,
76.2844791261685));
#220355=CARTESIAN_POINT('Ctrl Pts',(-34.0465706305509,87.4091332880509,
72.1167463655193));
#220356=CARTESIAN_POINT('Ctrl Pts',(-34.1442380168409,86.4163741266587,
68.0478748946176));
#220357=CARTESIAN_POINT('Ctrl Pts',(-34.2419054031309,84.1295181910076,
64.5390893883722));
#220358=CARTESIAN_POINT('Ctrl Pts',(-34.3395727894109,80.8077907707222,
61.9881262869919));
#220359=CARTESIAN_POINT('Ctrl Pts',(-34.4372401757009,76.8277244401432,
60.684148601805));
#220360=CARTESIAN_POINT('Ctrl Pts',(-34.5349075619909,72.6404774166431,
60.7749680020176));
#220361=CARTESIAN_POINT('Ctrl Pts',(-34.6325749482809,68.7206927704309,
62.2502897047617));
#220362=CARTESIAN_POINT('Ctrl Pts',(-34.7302423345709,65.5126955218893,
64.9428794344855));
#220363=CARTESIAN_POINT('Ctrl Pts',(-34.8279097208609,63.3801264246424,
68.5475201717518));
#220364=CARTESIAN_POINT('Ctrl Pts',(-34.9255771071509,62.5647216691142,
72.6556098596656));
#220365=CARTESIAN_POINT('Ctrl Pts',(-35.0232444934409,63.1589110103241,
76.8014782640017));
#220366=CARTESIAN_POINT('Ctrl Pts',(-35.1209118797309,65.0953404441711,
80.5151727650388));
#220367=CARTESIAN_POINT('Ctrl Pts',(-35.2185792660209,68.1545070833008,
83.3757295768015));
#220368=CARTESIAN_POINT('Ctrl Pts',(-35.3162466523109,71.9896407854853,
85.0588918641796));
#220369=CARTESIAN_POINT('Ctrl Pts',(-35.4139140386009,76.1660120912788,
85.3738656971174));
#220370=CARTESIAN_POINT('Ctrl Pts',(-35.5115814248909,80.2102107414312,
84.2849473910145));
#220371=CARTESIAN_POINT('Ctrl Pts',(-35.6092488111809,83.6638088349665,
81.9155706781228));
#220372=CARTESIAN_POINT('Ctrl Pts',(-35.7069161974709,86.1353256703195,
78.5343149451388));
#220373=CARTESIAN_POINT('Ctrl Pts',(-35.8045835837609,87.3446038237173,
74.5244605653653));
#220374=CARTESIAN_POINT('Ctrl Pts',(-35.9022509700509,87.1545662389771,
70.3405423640075));
#220375=CARTESIAN_POINT('Ctrl Pts',(-35.9999183563409,85.5867545214038,
66.4568260744839));
#220376=CARTESIAN_POINT('Ctrl Pts',(-36.0975857426309,82.818887101022,63.3135482085524));
#220377=CARTESIAN_POINT('Ctrl Pts',(-36.1952531289209,79.1647140582467,
61.2670132900358));
#220378=CARTESIAN_POINT('Ctrl Pts',(-36.2929205152109,75.0384521570716,
60.5492051525981));
#220379=CARTESIAN_POINT('Ctrl Pts',(-36.3905879015009,70.9078315329049,
61.2414905405987));
#220380=CARTESIAN_POINT('Ctrl Pts',(-36.4882552877909,67.2410764017834,
63.2653958268243));
#220381=CARTESIAN_POINT('Ctrl Pts',(-36.5859226740809,64.4538297633518,
66.3915023470505));
#220382=CARTESIAN_POINT('Ctrl Pts',(-36.6835900603709,62.8620384185835,
70.2654520258604));
#220383=CARTESIAN_POINT('Ctrl Pts',(-36.7812574466609,62.6461389948745,
74.4481154402485));
#220384=CARTESIAN_POINT('Ctrl Pts',(-36.8789248329509,63.8306046519742,
78.4653690924802));
#220385=CARTESIAN_POINT('Ctrl Pts',(-36.9765922192409,66.2811709404978,
81.8618394169132));
#220386=CARTESIAN_POINT('Ctrl Pts',(-37.0742596055309,69.7200552743181,
84.2525213986484));
#220387=CARTESIAN_POINT('Ctrl Pts',(-37.1719269918209,73.7574448219614,
85.3664206040375));
#220388=CARTESIAN_POINT('Ctrl Pts',(-37.2695943781109,77.935683524501,85.0772716047947));
#220389=CARTESIAN_POINT('Ctrl Pts',(-37.3672617644009,81.7811494449743,
83.4178507257861));
#220390=CARTESIAN_POINT('Ctrl Pts',(-37.4649291506909,84.8579419210346,
80.5762607028601));
#220391=CARTESIAN_POINT('Ctrl Pts',(-37.5625965369809,86.8172928434819,
76.8746084012713));
#220392=CARTESIAN_POINT('Ctrl Pts',(-37.6602639232709,87.4371010722797,
72.7324925701221));
#220393=CARTESIAN_POINT('Ctrl Pts',(-37.7579313095609,86.6471085885194,
68.6194404582812));
#220394=CARTESIAN_POINT('Ctrl Pts',(-37.8555986958509,84.5368645531706,
65.0016848127869));
#220395=CARTESIAN_POINT('Ctrl Pts',(-37.9532660821509,81.3455745117745,
62.2893143236978));
#220396=CARTESIAN_POINT('Ctrl Pts',(-38.0509334684409,77.4349853810736,
60.7897882475));
#220397=CARTESIAN_POINT('Ctrl Pts',(-38.1486008547309,73.2483798313682,
60.6730845330001));
#220398=CARTESIAN_POINT('Ctrl Pts',(-38.2462682410209,69.2603282096219,
61.9524320656215));
#220399=CARTESIAN_POINT('Ctrl Pts',(-38.3439356273109,65.9228939362941,
64.4828111119111));
#220400=CARTESIAN_POINT('Ctrl Pts',(-38.4416030136009,63.6143898973541,
67.9773919605015));
#220401=CARTESIAN_POINT('Ctrl Pts',(-38.5392703998909,62.5964957764151,
72.040048310785));
#220402=CARTESIAN_POINT('Ctrl Pts',(-38.6369377861809,62.9845925876825,
76.2102600797003));
#220403=CARTESIAN_POINT('Ctrl Pts',(-38.7346051724709,64.7346945898851,
80.0153149192111));
#220404=CARTESIAN_POINT('Ctrl Pts',(-38.8322725587709,67.648394717053,83.0238940611853));
#220405=CARTESIAN_POINT('Ctrl Pts',(-38.9299399450609,71.39550623112,84.8949575070187));
#220406=CARTESIAN_POINT('Ctrl Pts',(-38.9950515359209,74.1657861357241,
85.2426041509183));
#220407=CARTESIAN_POINT('Ctrl Pts',(-39.0276073313509,75.5406900979627,
85.1816337132427));
#220408=CARTESIAN_POINT('Ctrl Pts',(-33.0010227190609,70.2575692325718,
61.2773790062616));
#220409=CARTESIAN_POINT('Ctrl Pts',(-33.0335785144909,68.9369311879788,
61.8121549909076));
#220410=CARTESIAN_POINT('Ctrl Pts',(-33.0986901053509,66.4786349582126,
63.3326087841967));
#220411=CARTESIAN_POINT('Ctrl Pts',(-33.1963574916409,63.7568591148654,
66.7079795823175));
#220412=CARTESIAN_POINT('Ctrl Pts',(-33.2940248779309,62.3096145940082,
70.7952905623853));
#220413=CARTESIAN_POINT('Ctrl Pts',(-33.3916922642209,62.3008625847488,
75.1312634607482));
#220414=CARTESIAN_POINT('Ctrl Pts',(-33.4893596505109,63.7316193923605,
79.224386657865));
#220415=CARTESIAN_POINT('Ctrl Pts',(-33.5870270368009,66.4396958789624,
82.610689066389));
#220416=CARTESIAN_POINT('Ctrl Pts',(-33.6846944230909,70.1181212717175,
84.9063175455788));
#220417=CARTESIAN_POINT('Ctrl Pts',(-33.7823618093809,74.3499292288595,
85.8510525877097));
#220418=CARTESIAN_POINT('Ctrl Pts',(-33.8800291956709,78.6554256250739,
85.3378042240803));
#220419=CARTESIAN_POINT('Ctrl Pts',(-33.9776965819609,82.5465632644516,
83.4247514525909));
#220420=CARTESIAN_POINT('Ctrl Pts',(-34.0753639682509,85.5822644011988,
80.32874730835));
#220421=CARTESIAN_POINT('Ctrl Pts',(-34.1730313545409,87.4184188097211,
76.4007376295671));
#220422=CARTESIAN_POINT('Ctrl Pts',(-34.2706987408209,87.8468902233397,
72.0859797803774));
#220423=CARTESIAN_POINT('Ctrl Pts',(-34.3683661271109,86.8191095017967,
67.8735707501784));
#220424=CARTESIAN_POINT('Ctrl Pts',(-34.4660335134009,84.4515801603142,
64.2410058345146));
#220425=CARTESIAN_POINT('Ctrl Pts',(-34.5637008996909,81.0126721778146,
61.6000524200778));
#220426=CARTESIAN_POINT('Ctrl Pts',(-34.6613682859809,76.8922010664508,
60.250074320352));
#220427=CARTESIAN_POINT('Ctrl Pts',(-34.7590356722709,72.5572405498546,
60.3440975560973));
#220428=CARTESIAN_POINT('Ctrl Pts',(-34.8567030585609,68.4991776795392,
61.8714641754451));
#220429=CARTESIAN_POINT('Ctrl Pts',(-34.9543704448509,65.1780119274846,
64.6590403800947));
#220430=CARTESIAN_POINT('Ctrl Pts',(-35.0520378311409,62.9702122004541,
68.390842011297));
#220431=CARTESIAN_POINT('Ctrl Pts',(-35.1497052174309,62.1260424152783,
72.6438527593594));
#220432=CARTESIAN_POINT('Ctrl Pts',(-35.2473726037209,62.7411929710006,
76.9359749434432));
#220433=CARTESIAN_POINT('Ctrl Pts',(-35.3450399900109,64.7459338166531,
80.780677427527));
#220434=CARTESIAN_POINT('Ctrl Pts',(-35.4427073763009,67.9130186625803,
83.7421460881763));
#220435=CARTESIAN_POINT('Ctrl Pts',(-35.5403747625909,71.8834443579084,
85.484685283491));
#220436=CARTESIAN_POINT('Ctrl Pts',(-35.6380421488809,76.2071454941548,
85.8107704468362));
#220437=CARTESIAN_POINT('Ctrl Pts',(-35.7357095351709,80.3940113206321,
84.6834383749048));
#220438=CARTESIAN_POINT('Ctrl Pts',(-35.8333769214609,83.9694419775097,
82.2304771711338));
#220439=CARTESIAN_POINT('Ctrl Pts',(-35.9310443077509,86.5281465003784,
78.729940895939));
#220440=CARTESIAN_POINT('Ctrl Pts',(-36.0287116940409,87.7800843533953,
74.5786309025152));
#220441=CARTESIAN_POINT('Ctrl Pts',(-36.1263790803309,87.5833428137125,
70.2471166389011));
#220442=CARTESIAN_POINT('Ctrl Pts',(-36.2240464666209,85.9602234097461,
66.2263945085208));
#220443=CARTESIAN_POINT('Ctrl Pts',(-36.3217138529109,83.0947139437118,
62.9722312444263));
#220444=CARTESIAN_POINT('Ctrl Pts',(-36.4193812392009,79.3116326561084,
60.8535007234067));
#220445=CARTESIAN_POINT('Ctrl Pts',(-36.5170486254909,75.0398086337074,
60.1103704717333));
#220446=CARTESIAN_POINT('Ctrl Pts',(-36.6147160117809,70.7634721256552,
60.8270776080123));
#220447=CARTESIAN_POINT('Ctrl Pts',(-36.7123833980709,66.967364891402,62.9223801912565));
#220448=CARTESIAN_POINT('Ctrl Pts',(-36.8100507843609,64.0817925667024,
66.1587663561376));
#220449=CARTESIAN_POINT('Ctrl Pts',(-36.9077181706509,62.433847606303,70.1693773391154));
#220450=CARTESIAN_POINT('Ctrl Pts',(-37.0053855569409,62.2103318996323,
74.4995925506424));
#220451=CARTESIAN_POINT('Ctrl Pts',(-37.1030529432309,63.4365819459936,
78.6585628406411));
#220452=CARTESIAN_POINT('Ctrl Pts',(-37.2007203295209,65.9735968496646,
82.1748504323778));
#220453=CARTESIAN_POINT('Ctrl Pts',(-37.2983877158209,69.5337946895659,
84.6498684909033));
#220454=CARTESIAN_POINT('Ctrl Pts',(-37.3960551021109,73.7136112088471,
85.8030627132265));
#220455=CARTESIAN_POINT('Ctrl Pts',(-37.4937224884009,78.0392456179921,
85.5037134061586));
#220456=CARTESIAN_POINT('Ctrl Pts',(-37.5913898746909,82.0203680212412,
83.7857531448031));
#220457=CARTESIAN_POINT('Ctrl Pts',(-37.6890572609809,85.2057004907068,
80.8439203643352));
#220458=CARTESIAN_POINT('Ctrl Pts',(-37.7867246472709,87.2341714262334,
77.0116848923229));
#220459=CARTESIAN_POINT('Ctrl Pts',(-37.8843920335609,87.8758446269618,
72.7234476609321));
#220460=CARTESIAN_POINT('Ctrl Pts',(-37.9820594198509,87.0579835821749,
68.4652994295259));
#220461=CARTESIAN_POINT('Ctrl Pts',(-38.0797268061409,84.873296478161,64.7199202355244));
#220462=CARTESIAN_POINT('Ctrl Pts',(-38.1773941924309,81.5694273133449,
61.9118654657189));
#220463=CARTESIAN_POINT('Ctrl Pts',(-38.2750615787209,77.520884348699,60.3594406153311));
#220464=CARTESIAN_POINT('Ctrl Pts',(-38.3727289650109,73.1865879351576,
60.238619944442));
#220465=CARTESIAN_POINT('Ctrl Pts',(-38.4703963513009,69.0578498355331,
61.5630990137956));
#220466=CARTESIAN_POINT('Ctrl Pts',(-38.5680637375909,65.602680909391,64.1827422295159));
#220467=CARTESIAN_POINT('Ctrl Pts',(-38.6657311238809,63.2127397845698,
67.8006013898867));
#220468=CARTESIAN_POINT('Ctrl Pts',(-38.7633985101709,62.1589374176099,
72.0065760486925));
#220469=CARTESIAN_POINT('Ctrl Pts',(-38.8610658964609,62.5607251182124,
76.3239003581206));
#220470=CARTESIAN_POINT('Ctrl Pts',(-38.9587332827509,64.3725654603181,
80.2631860989099));
#220471=CARTESIAN_POINT('Ctrl Pts',(-39.0564006690409,67.3890521728565,
83.3778988728009));
#220472=CARTESIAN_POINT('Ctrl Pts',(-39.1540680553309,71.2683505217792,
85.3149678148183));
#220473=CARTESIAN_POINT('Ctrl Pts',(-39.2191796461909,74.1363575772585,
85.6748783876892));
#220474=CARTESIAN_POINT('Ctrl Pts',(-39.2517354416209,75.5597640199593,
85.6117570961773));
#220475=CARTESIAN_POINT('Ctrl Pts',(-33.2251508293409,70.0959712176063,
60.8783100640841));
#220476=CARTESIAN_POINT('Ctrl Pts',(-33.2577066247709,68.7303325189268,
61.4313085050616));
#220477=CARTESIAN_POINT('Ctrl Pts',(-33.3228182156309,66.1882700076009,
63.0035716608669));
#220478=CARTESIAN_POINT('Ctrl Pts',(-33.4204856019209,63.3737498322777,
66.4939579958501));
#220479=CARTESIAN_POINT('Ctrl Pts',(-33.5181529882109,61.8771905500222,
70.7205438274275));
#220480=CARTESIAN_POINT('Ctrl Pts',(-33.6158203745009,61.8681403166308,
75.2042647157331));
#220481=CARTESIAN_POINT('Ctrl Pts',(-33.7134877607909,63.3476500679026,
79.4368608152641));
#220482=CARTESIAN_POINT('Ctrl Pts',(-33.8111551470709,66.1480040818002,
82.9385512545613));
#220483=CARTESIAN_POINT('Ctrl Pts',(-33.9088225333609,69.9517715767027,
85.3124031224554));
#220484=CARTESIAN_POINT('Ctrl Pts',(-34.0064899196509,74.3277781103001,
86.2893299487034));
#220485=CARTESIAN_POINT('Ctrl Pts',(-34.1041573059409,78.7799840116568,
85.7585926810094));
#220486=CARTESIAN_POINT('Ctrl Pts',(-34.2018246922309,82.8037119089286,
83.7803527627689));
#220487=CARTESIAN_POINT('Ctrl Pts',(-34.2994920785209,85.9428543612762,
80.5788524819328));
#220488=CARTESIAN_POINT('Ctrl Pts',(-34.3971594648109,87.8415756099131,
76.5169961329518));
#220489=CARTESIAN_POINT('Ctrl Pts',(-34.4948268511009,88.2846471586345,
72.0552131952207));
#220490=CARTESIAN_POINT('Ctrl Pts',(-34.5924942373909,87.2218448769265,
67.6992666057196));
#220491=CARTESIAN_POINT('Ctrl Pts',(-34.6901616236809,84.7736421296089,
63.9429222806305));
#220492=CARTESIAN_POINT('Ctrl Pts',(-34.7878290099709,81.2175535848858,
61.2119785531442));
#220493=CARTESIAN_POINT('Ctrl Pts',(-34.8854963962609,76.9566776927288,
59.8160000388975));
#220494=CARTESIAN_POINT('Ctrl Pts',(-34.9831637825509,72.4740036830308,
59.9132271101949));
#220495=CARTESIAN_POINT('Ctrl Pts',(-35.0808311688409,68.2776625886137,
61.4926386461447));
#220496=CARTESIAN_POINT('Ctrl Pts',(-35.1784985551309,64.8433283330666,
64.3752013257362));
#220497=CARTESIAN_POINT('Ctrl Pts',(-35.2761659414209,62.56029797625,68.2341638508804));
#220498=CARTESIAN_POINT('Ctrl Pts',(-35.3738333277109,61.6873631614363,
72.6320956590941));
#220499=CARTESIAN_POINT('Ctrl Pts',(-35.4715007140009,62.3234749316971,
77.0704716229308));
#220500=CARTESIAN_POINT('Ctrl Pts',(-35.5691681002909,64.3965271891681,
81.0461820900504));
#220501=CARTESIAN_POINT('Ctrl Pts',(-35.6668354865809,67.6715302419011,
84.1085625995897));
#220502=CARTESIAN_POINT('Ctrl Pts',(-35.7645028728709,71.7772479303871,
85.9104787028145));
#220503=CARTESIAN_POINT('Ctrl Pts',(-35.8621702591609,76.2482788970921,
86.247675196548));
#220504=CARTESIAN_POINT('Ctrl Pts',(-35.9598376454509,80.5778118998904,
85.081929358769));
#220505=CARTESIAN_POINT('Ctrl Pts',(-36.0575050317409,84.2750751200944,
82.5453836640971));
#220506=CARTESIAN_POINT('Ctrl Pts',(-36.1551724180309,86.9209673304724,
78.9255668466804));
#220507=CARTESIAN_POINT('Ctrl Pts',(-36.2528398043209,88.2155648830812,
74.6328012395938));
#220508=CARTESIAN_POINT('Ctrl Pts',(-36.3505071906109,88.0121193884434,
70.1536909137269));
#220509=CARTESIAN_POINT('Ctrl Pts',(-36.4481745769009,86.333692298055,65.995962942479));
#220510=CARTESIAN_POINT('Ctrl Pts',(-36.5458419631909,83.3705407863494,
62.6309142802354));
#220511=CARTESIAN_POINT('Ctrl Pts',(-36.6435093494809,79.4585512538933,
60.4399881567567));
#220512=CARTESIAN_POINT('Ctrl Pts',(-36.7411767357709,75.0411651102624,
59.6715357908677));
#220513=CARTESIAN_POINT('Ctrl Pts',(-36.8388441220609,70.6191127183272,
60.4126646754531));
#220514=CARTESIAN_POINT('Ctrl Pts',(-36.9365115083509,66.6936533809556,
62.5793645557409));
#220515=CARTESIAN_POINT('Ctrl Pts',(-37.0341788946409,63.7097553700125,
65.9260303652965));
#220516=CARTESIAN_POINT('Ctrl Pts',(-37.1318462809309,62.005656794,70.0733026524509));
#220517=CARTESIAN_POINT('Ctrl Pts',(-37.2295136672209,61.7745248044076,
74.5510696611246));
#220518=CARTESIAN_POINT('Ctrl Pts',(-37.3271810535109,63.0425592400513,
78.8517565888796));
#220519=CARTESIAN_POINT('Ctrl Pts',(-37.4248484398009,65.6660227588901,
82.4878614479098));
#220520=CARTESIAN_POINT('Ctrl Pts',(-37.5225158260909,69.3475341048888,
85.0472155832));
#220521=CARTESIAN_POINT('Ctrl Pts',(-37.6201832123809,73.6697775958153,
86.239704822428));
#220522=CARTESIAN_POINT('Ctrl Pts',(-37.7178505986709,78.142807711568,85.9301552074927));
#220523=CARTESIAN_POINT('Ctrl Pts',(-37.8155179849609,82.2595865975891,
84.1536555637811));
#220524=CARTESIAN_POINT('Ctrl Pts',(-37.9131853712509,85.5534590604176,
81.111580025743));
#220525=CARTESIAN_POINT('Ctrl Pts',(-38.0108527575409,87.6510500090054,
77.1487613832987));
#220526=CARTESIAN_POINT('Ctrl Pts',(-38.1085201438309,88.3145881816426,
72.7144027516668));
#220527=CARTESIAN_POINT('Ctrl Pts',(-38.2061875301209,87.4688585758041,
68.3111584007035));
#220528=CARTESIAN_POINT('Ctrl Pts',(-38.3038549164109,85.2097284031102,
64.4381556582015));
#220529=CARTESIAN_POINT('Ctrl Pts',(-38.4015223027009,81.793280114859,61.534416607706));
#220530=CARTESIAN_POINT('Ctrl Pts',(-38.4991896889909,77.6067833162661,
59.9290929831489));
#220531=CARTESIAN_POINT('Ctrl Pts',(-38.5968570752809,73.124796038894,59.8041553558838));
#220532=CARTESIAN_POINT('Ctrl Pts',(-38.6945244615809,68.8553714613998,
61.1737659619935));
#220533=CARTESIAN_POINT('Ctrl Pts',(-38.7921918478709,65.2824678824627,
63.8826733471558));
#220534=CARTESIAN_POINT('Ctrl Pts',(-38.8898592341609,62.8110896717617,
67.6238108193034));
#220535=CARTESIAN_POINT('Ctrl Pts',(-38.9875266204509,61.7213790587936,
71.9731037866268));
#220536=CARTESIAN_POINT('Ctrl Pts',(-39.0851940067409,62.1368576487401,
76.4375406365595));
#220537=CARTESIAN_POINT('Ctrl Pts',(-39.1828613930309,64.010436330763,80.5110572786137));
#220538=CARTESIAN_POINT('Ctrl Pts',(-39.2805287793209,67.1297096286665,
83.7319036844192));
#220539=CARTESIAN_POINT('Ctrl Pts',(-39.3781961656109,71.1411948124404,
85.7349781226078));
#220540=CARTESIAN_POINT('Ctrl Pts',(-39.4433077564709,74.1069290187816,
86.1071526244663));
#220541=CARTESIAN_POINT('Ctrl Pts',(-39.4758635519009,75.5788379419391,
86.0418804791266));
#220542=CARTESIAN_POINT('Ctrl Pts',(-37.9553013376164,87.0149197239272,
77.9529304850788));
#220543=CARTESIAN_POINT('Ctrl Pts',(-37.9473977182868,86.8780015006863,
78.2843261017427));
#220544=CARTESIAN_POINT('Ctrl Pts',(-37.9394869538629,86.7273493680408,
78.6101129500371));
#220545=CARTESIAN_POINT('Ctrl Pts',(-37.9144970719214,86.2123909976008,
79.6124821634823));
#220546=CARTESIAN_POINT('Ctrl Pts',(-37.8972347154438,85.8016507088589,
80.2630920822533));
#220547=CARTESIAN_POINT('Ctrl Pts',(-37.861062749303,84.8147782119131,81.5567570438918));
#220548=CARTESIAN_POINT('Ctrl Pts',(-37.8423268283133,84.2272138908917,
82.1865390631675));
#220549=CARTESIAN_POINT('Ctrl Pts',(-37.8109352049774,83.1683559811119,
83.1171154920924));
#220550=CARTESIAN_POINT('Ctrl Pts',(-37.7985801514998,82.7322228035195,
83.4538658241038));
#220551=CARTESIAN_POINT('Ctrl Pts',(-37.7691043490261,81.6361366088174,
84.1941557057341));
#220552=CARTESIAN_POINT('Ctrl Pts',(-37.752257135375,80.9589745053308,84.5684803366103));
#220553=CARTESIAN_POINT('Ctrl Pts',(-37.7176808869081,79.5333123286061,
85.19820586662));
#220554=CARTESIAN_POINT('Ctrl Pts',(-37.6999867825758,78.7866758654998,
85.4500052364488));
#220555=CARTESIAN_POINT('Ctrl Pts',(-37.6640158185303,77.2101795397193,
85.8267863844493));
#220556=CARTESIAN_POINT('Ctrl Pts',(-37.6457917771104,76.3816799860254,
85.9421693852411));
#220557=CARTESIAN_POINT('Ctrl Pts',(-37.6179096810754,75.1310310523308,
85.994921893685));
#220558=CARTESIAN_POINT('Ctrl Pts',(-37.6085662507976,74.7136034370356,
85.9924283920031));
#220559=CARTESIAN_POINT('Ctrl Pts',(-37.5800024872725,73.4378254535915,
85.9233392433153));
#220560=CARTESIAN_POINT('Ctrl Pts',(-37.5612098452054,72.5853703586956,
85.7916214301034));
#220561=CARTESIAN_POINT('Ctrl Pts',(-37.5247937388324,70.9944744540827,
85.3811504603076));
#220562=CARTESIAN_POINT('Ctrl Pts',(-37.5072061451635,70.2559520398793,
85.1176307511489));
#220563=CARTESIAN_POINT('Ctrl Pts',(-37.4706993708442,68.7656494933135,
84.4287851334567));
#220564=CARTESIAN_POINT('Ctrl Pts',(-37.4519645638645,68.023333774558,83.9918197602286));
#220565=CARTESIAN_POINT('Ctrl Pts',(-37.4235242747022,66.9920845151175,
83.2381830196114));
#220566=CARTESIAN_POINT('Ctrl Pts',(-37.4141649327465,66.6666862632069,
82.9754108736812));
#220567=CARTESIAN_POINT('Ctrl Pts',(-37.3855787197163,65.7119637817133,
82.1252268095932));
#220568=CARTESIAN_POINT('Ctrl Pts',(-37.3667763651694,65.1278034430708,
81.4906548248999));
#220569=CARTESIAN_POINT('Ctrl Pts',(-37.3288886089769,64.0999456460148,
80.1240580683699));
#220570=CARTESIAN_POINT('Ctrl Pts',(-37.3097662096208,63.6570533065481,
79.3966479349764));
#220571=CARTESIAN_POINT('Ctrl Pts',(-37.272377703877,62.9253191437379,77.877807166774));
#220572=CARTESIAN_POINT('Ctrl Pts',(-37.254105190141,62.6358835506584,77.0910921468174));
#220573=CARTESIAN_POINT('Ctrl Pts',(-37.2261945528014,62.3185864199717,
75.8793905009494));
#220574=CARTESIAN_POINT('Ctrl Pts',(-37.2168704007062,62.2325462548658,
75.4719058965277));
#220575=CARTESIAN_POINT('Ctrl Pts',(-37.1883348797388,62.0290488504922,
74.211526283995));
#220576=CARTESIAN_POINT('Ctrl Pts',(-37.1695527699318,61.976573836333,73.3505341020265));
#220577=CARTESIAN_POINT('Ctrl Pts',(-37.1324546123145,62.0406925031923,
71.6786460362011));
#220578=CARTESIAN_POINT('Ctrl Pts',(-37.1141663102993,62.1479090448059,
70.8713107952548));
#220579=CARTESIAN_POINT('Ctrl Pts',(-37.0776055317186,62.516745874674,69.2651664320858));
#220580=CARTESIAN_POINT('Ctrl Pts',(-37.0593609631848,62.7817337808106,
68.4709556012001));
#220581=CARTESIAN_POINT('Ctrl Pts',(-37.0287563265744,63.3398217425991,
67.215660861289));
#220582=CARTESIAN_POINT('Ctrl Pts',(-37.0166706476576,63.5889203893348,
66.7377147055205));
#220583=CARTESIAN_POINT('Ctrl Pts',(-36.9874851404225,64.265238862123,65.615967360191));
#220584=CARTESIAN_POINT('Ctrl Pts',(-36.9706554575621,64.7215535366351,
64.9921015471903));
#220585=CARTESIAN_POINT('Ctrl Pts',(-36.9368299488605,65.7273512419191,
63.8463945870026));
#220586=CARTESIAN_POINT('Ctrl Pts',(-36.9198965793821,66.2724671296937,
63.3246570379016));
#220587=CARTESIAN_POINT('Ctrl Pts',(-36.8938644179974,67.1856908905406,
62.591225377354));
#220588=CARTESIAN_POINT('Ctrl Pts',(-36.8846757297518,67.5241519284592,
62.3452743724052));
#220589=CARTESIAN_POINT('Ctrl Pts',(-36.8533476324862,68.7122918766856,
61.5665594371299));
#220590=CARTESIAN_POINT('Ctrl Pts',(-36.8309230429486,69.6114607858468,
61.1158732118304));
#220591=CARTESIAN_POINT('Ctrl Pts',(-36.789449487936,71.3612978449459,60.478934483044));
#220592=CARTESIAN_POINT('Ctrl Pts',(-36.7707178993297,72.1963470791442,
60.2657349591826));
#220593=CARTESIAN_POINT('Ctrl Pts',(-36.7386712593778,73.6205739630213,
60.0492377450129));
#220594=CARTESIAN_POINT('Ctrl Pts',(-36.7256353126083,74.2000425611145,
60.0005305295167));
#220595=CARTESIAN_POINT('Ctrl Pts',(-36.6954200029145,75.5551736723792,
59.9776797136377));
#220596=CARTESIAN_POINT('Ctrl Pts',(-36.6785226409056,76.3291455552397,
60.0338452720972));
#220597=CARTESIAN_POINT('Ctrl Pts',(-36.6444393144889,77.8457582702571,
60.2813083747787));
#220598=CARTESIAN_POINT('Ctrl Pts',(-36.627304088817,78.5857589156217,60.4699725631839));
#220599=CARTESIAN_POINT('Ctrl Pts',(-36.5912629985634,80.1156502750462,
61.006890255804));
#220600=CARTESIAN_POINT('Ctrl Pts',(-36.5725265788013,80.8961498629526,
61.3710752105735));
#220601=CARTESIAN_POINT('Ctrl Pts',(-36.5440917128894,81.9941544883828,
62.02274903122));
#220602=CARTESIAN_POINT('Ctrl Pts',(-36.5347393239334,82.342829524566,62.2530948295483));
#220603=CARTESIAN_POINT('Ctrl Pts',(-36.5061627867831,83.3740467851531,
63.0081240833622));
#220604=CARTESIAN_POINT('Ctrl Pts',(-36.4873647837522,84.016106273638,63.5840945893444));
#220605=CARTESIAN_POINT('Ctrl Pts',(-36.4508287270845,85.1283164207911,
64.8011777565554));
#220606=CARTESIAN_POINT('Ctrl Pts',(-36.4331132215764,85.6060584898116,
65.4302567802297));
#220607=CARTESIAN_POINT('Ctrl Pts',(-36.3984301762445,86.4326940815265,
66.7528247587721));
#220608=CARTESIAN_POINT('Ctrl Pts',(-36.3815971455766,86.7824975342673,
67.4420206214496));
#220609=CARTESIAN_POINT('Ctrl Pts',(-36.3484649019024,87.3367234482972,
68.8267002318701));
#220610=CARTESIAN_POINT('Ctrl Pts',(-36.3322686753667,87.5483011039315,
69.5163260239332));
#220611=CARTESIAN_POINT('Ctrl Pts',(-36.3002569422523,87.8552943718372,
70.9245458454455));
#220612=CARTESIAN_POINT('Ctrl Pts',(-36.2845007615987,87.9500046304174,
71.6407444007544));
#220613=CARTESIAN_POINT('Ctrl Pts',(-36.2513677547274,88.0220816726077,
73.1315272035965));
#220614=CARTESIAN_POINT('Ctrl Pts',(-36.2340081542728,87.9906885105661,
73.9037468834361));
#220615=CARTESIAN_POINT('Ctrl Pts',(-36.1994040444401,87.7891197532016,
75.4506851129428));
#220616=CARTESIAN_POINT('Ctrl Pts',(-36.1821713308326,87.6162554705602,
76.2218644197147));
#220617=CARTESIAN_POINT('Ctrl Pts',(-36.1568663165708,87.2678008992854,
77.3042636933753));
#220618=CARTESIAN_POINT('Ctrl Pts',(-36.149081613326,87.1478054025579,77.6312952059185));
#220619=CARTESIAN_POINT('Ctrl Pts',(-36.1412950695185,87.0149197055719,
77.9529305295058));
#220620=CARTESIAN_POINT('',(-32.7070373297029,66.4977334966964,64.749780674319));
#220621=CARTESIAN_POINT('Ctrl Pts',(-26.5424658037409,86.773203990145,73.1405558201253));
#220622=CARTESIAN_POINT('Ctrl Pts',(-26.5750215991709,86.7903065205387,
71.812960950527));
#220623=CARTESIAN_POINT('Ctrl Pts',(-26.6401331900309,86.3710927791314,
69.1522693813868));
#220624=CARTESIAN_POINT('Ctrl Pts',(-26.7378005763209,84.4533116811586,
65.595862444819));
#220625=CARTESIAN_POINT('Ctrl Pts',(-26.8354679626109,81.4639547431525,
62.8775596699702));
#220626=CARTESIAN_POINT('Ctrl Pts',(-26.9331353489009,77.7418800381493,
61.3054018749864));
#220627=CARTESIAN_POINT('Ctrl Pts',(-27.0308027351909,73.7090009717682,
61.0576244908064));
#220628=CARTESIAN_POINT('Ctrl Pts',(-27.1284701214809,69.8224624038905,
62.1623076602057));
#220629=CARTESIAN_POINT('Ctrl Pts',(-27.2261375077709,66.5228207415521,
64.4942323820705));
#220630=CARTESIAN_POINT('Ctrl Pts',(-27.3238048940609,64.1841050462514,
67.789064150928));
#220631=CARTESIAN_POINT('Ctrl Pts',(-27.4214722803509,63.0714191403804,
71.6733192596676));
#220632=CARTESIAN_POINT('Ctrl Pts',(-27.5191396666409,63.3108909197464,
75.7067000853347));
#220633=CARTESIAN_POINT('Ctrl Pts',(-27.6168070529309,64.8753751931555,
79.4320049844844));
#220634=CARTESIAN_POINT('Ctrl Pts',(-27.7144744392209,67.5875307112038,
82.4269540784776));
#220635=CARTESIAN_POINT('Ctrl Pts',(-27.8121418255109,71.139922585341,84.3520565700369));
#220636=CARTESIAN_POINT('Ctrl Pts',(-27.9098092118009,75.129871399649,84.9890935309176));
#220637=CARTESIAN_POINT('Ctrl Pts',(-28.0074765980909,79.1050987132879,
84.2658539888279));
#220638=CARTESIAN_POINT('Ctrl Pts',(-28.1051439843809,82.6149948329797,
82.2643203620044));
#220639=CARTESIAN_POINT('Ctrl Pts',(-28.2028113706709,85.2616974255471,
79.211375387585));
#220640=CARTESIAN_POINT('Ctrl Pts',(-28.3004787569609,86.745190982611,75.4530839544341));
#220641=CARTESIAN_POINT('Ctrl Pts',(-28.3981461432509,86.8973149125801,
71.4154651090891));
#220642=CARTESIAN_POINT('Ctrl Pts',(-28.4958135295409,85.7008252915377,
67.5562009023972));
#220643=CARTESIAN_POINT('Ctrl Pts',(-28.5934809158309,83.2913495386348,
64.3127560937844));
#220644=CARTESIAN_POINT('Ctrl Pts',(-28.6911483021209,79.9420124450654,
62.0527895754545));
#220645=CARTESIAN_POINT('Ctrl Pts',(-28.7888156884109,76.0324762644166,
61.0324786020043));
#220646=CARTESIAN_POINT('Ctrl Pts',(-28.8864830747009,72.005904307922,61.367479959455));
#220647=CARTESIAN_POINT('Ctrl Pts',(-28.9841504609909,68.3187264124431,
63.0198197542422));
#220648=CARTESIAN_POINT('Ctrl Pts',(-29.0818178472809,65.3889005887908,
65.8021979228998));
#220649=CARTESIAN_POINT('Ctrl Pts',(-29.1794852335709,63.5485356226125,
69.399219527172));
#220650=CARTESIAN_POINT('Ctrl Pts',(-29.2771526198609,63.00624506665,73.403146172761));
#220651=CARTESIAN_POINT('Ctrl Pts',(-29.3748200061509,63.823499966919,77.3601149694953));
#220652=CARTESIAN_POINT('Ctrl Pts',(-29.4724873924409,65.9076608462574,
80.8215859081835));
#220653=CARTESIAN_POINT('Ctrl Pts',(-29.5701547787309,69.0224788010218,
83.3951858652539));
#220654=CARTESIAN_POINT('Ctrl Pts',(-29.6678221650209,72.8148753648847,
84.789185841132));
#220655=CARTESIAN_POINT('Ctrl Pts',(-29.7654895513109,76.8549655230795,
84.8455697396331));
#220656=CARTESIAN_POINT('Ctrl Pts',(-29.8631569376009,80.6847870904639,
83.5579461951268));
#220657=CARTESIAN_POINT('Ctrl Pts',(-29.9608243238909,83.8702127616981,
81.0722730622719));
#220658=CARTESIAN_POINT('Ctrl Pts',(-30.0584917101809,86.0501603718022,
77.6703124441068));
#220659=CARTESIAN_POINT('Ctrl Pts',(-30.1561590964709,86.9775231652655,
73.7376917047466));
#220660=CARTESIAN_POINT('Ctrl Pts',(-30.2538264827609,86.5471804455886,
69.720190892803));
#220661=CARTESIAN_POINT('Ctrl Pts',(-30.3514938690509,84.8079134737197,
66.0732115905698));
#220662=CARTESIAN_POINT('Ctrl Pts',(-30.4491612553409,81.956875895195,63.2101551195606));
#220663=CARTESIAN_POINT('Ctrl Pts',(-30.5468286416309,78.3172454977062,
61.4555616623674));
#220664=CARTESIAN_POINT('Ctrl Pts',(-30.6444960279209,74.3015905717297,
61.0083221897942));
#220665=CARTESIAN_POINT('Ctrl Pts',(-30.7421634142109,70.365103460175,61.9191332848712));
#220666=CARTESIAN_POINT('Ctrl Pts',(-30.8398308005009,66.9540024821432,
64.0847504597222));
#220667=CARTESIAN_POINT('Ctrl Pts',(-30.9374981867909,64.4549511021745,
67.2596913773823));
#220668=CARTESIAN_POINT('Ctrl Pts',(-31.0351655730809,63.1512279071195,
71.0840623663198));
#220669=CARTESIAN_POINT('Ctrl Pts',(-31.1328329593709,63.1906157186087,
75.1243539684998));
#220670=CARTESIAN_POINT('Ctrl Pts',(-31.2305003456609,64.5686497530634,
78.9225811642114));
#220671=CARTESIAN_POINT('Ctrl Pts',(-31.3281677319509,67.1291237247518,
82.0481980106354));
#220672=CARTESIAN_POINT('Ctrl Pts',(-31.4258351182409,70.5817965229168,
84.1469019390543));
#220673=CARTESIAN_POINT('Ctrl Pts',(-31.5235025045309,74.5352923323311,
84.980795526557));
#220674=CARTESIAN_POINT('Ctrl Pts',(-31.6211698908209,78.5414648223814,
84.4553532267351));
#220675=CARTESIAN_POINT('Ctrl Pts',(-31.7188372771109,82.1461965263699,
82.630136261015));
#220676=CARTESIAN_POINT('Ctrl Pts',(-31.8165046634009,84.9408750761412,
79.712041088333));
#220677=CARTESIAN_POINT('Ctrl Pts',(-31.9141720496909,86.6087112297139,
76.031846775141));
#220678=CARTESIAN_POINT('Ctrl Pts',(-32.0118394359809,86.9606483455424,
72.0067197036773));
#220679=CARTESIAN_POINT('Ctrl Pts',(-32.1095068222709,85.9567927749161,
68.0929259582382));
#220680=CARTESIAN_POINT('Ctrl Pts',(-32.2071742085609,83.7109360542007,
64.7341113461544));
#220681=CARTESIAN_POINT('Ctrl Pts',(-32.3048415948509,80.4776558675686,
62.3110128795057));
#220682=CARTESIAN_POINT('Ctrl Pts',(-32.4025089811409,76.6234595071886,
61.0982979039962));
#220683=CARTESIAN_POINT('Ctrl Pts',(-32.5001763674309,72.5852350114378,
61.233439177867));
#220684=CARTESIAN_POINT('Ctrl Pts',(-32.5978437537209,68.8207415117928,
62.7010949855073));
#220685=CARTESIAN_POINT('Ctrl Pts',(-32.6955111400109,65.7566696348843,
65.3349852966985));
#220686=CARTESIAN_POINT('Ctrl Pts',(-32.7606227308709,64.4125318335594,
67.6691475357373));
#220687=CARTESIAN_POINT('Ctrl Pts',(-32.7931785263009,63.9531251169506,
68.9148385500207));
#220688=CARTESIAN_POINT('Ctrl Pts',(-26.7665939140209,87.2037143630092,
73.1461018017395));
#220689=CARTESIAN_POINT('Ctrl Pts',(-26.7991497094509,87.2214422810865,
71.7699608131094));
#220690=CARTESIAN_POINT('Ctrl Pts',(-26.8642613003109,86.7868991642302,
69.0119758206587));
#220691=CARTESIAN_POINT('Ctrl Pts',(-26.9619286865909,84.7989906263339,
65.3255218656522));
#220692=CARTESIAN_POINT('Ctrl Pts',(-27.0595960728809,81.7003219690098,
62.5078190003946));
#220693=CARTESIAN_POINT('Ctrl Pts',(-27.1572634591709,77.8421422775993,
60.8781721617227));
#220694=CARTESIAN_POINT('Ctrl Pts',(-27.2549308454609,73.6617930516903,
60.6213343098834));
#220695=CARTESIAN_POINT('Ctrl Pts',(-27.3525982317509,69.6331355526051,
61.766412393317));
#220696=CARTESIAN_POINT('Ctrl Pts',(-27.4502656180409,66.212835999391,64.1836085317264));
#220697=CARTESIAN_POINT('Ctrl Pts',(-27.5479330043309,63.7886005622341,
67.5989223082414));
#220698=CARTESIAN_POINT('Ctrl Pts',(-27.6456003906209,62.6352271065125,
71.6252128490112));
#220699=CARTESIAN_POINT('Ctrl Pts',(-27.7432677769109,62.8834556427626,
75.8060821820242));
#220700=CARTESIAN_POINT('Ctrl Pts',(-27.8409351632009,64.5051483624386,
79.6676101859859));
#220701=CARTESIAN_POINT('Ctrl Pts',(-27.9386025494909,67.3164791843653,
82.7720754874778));
#220702=CARTESIAN_POINT('Ctrl Pts',(-28.0362699357809,70.9987712582735,
84.767573140128));
#220703=CARTESIAN_POINT('Ctrl Pts',(-28.1339373220709,75.1346204029575,
85.4279046111303));
#220704=CARTESIAN_POINT('Ctrl Pts',(-28.2316047083609,79.2552097263266,
84.678218391901));
#220705=CARTESIAN_POINT('Ctrl Pts',(-28.3292720946509,82.8934521049011,
82.6034947491146));
#220706=CARTESIAN_POINT('Ctrl Pts',(-28.4269394809409,85.6369365863143,
79.4389128336909));
#220707=CARTESIAN_POINT('Ctrl Pts',(-28.5246068672309,87.1746770047232,
75.5431920781981));
#220708=CARTESIAN_POINT('Ctrl Pts',(-28.6222742535209,87.3323636455694,
71.3579297539834));
#220709=CARTESIAN_POINT('Ctrl Pts',(-28.7199416398109,86.0921220269066,
67.3575439567694));
#220710=CARTESIAN_POINT('Ctrl Pts',(-28.8176090261009,83.5945390513956,
63.9954962058266));
#220711=CARTESIAN_POINT('Ctrl Pts',(-28.9152764123909,80.1227268557061,
61.6528895642724));
#220712=CARTESIAN_POINT('Ctrl Pts',(-29.0129437986809,76.0702307908808,
60.5952689121648));
#220713=CARTESIAN_POINT('Ctrl Pts',(-29.1106111849709,71.8964193067431,
60.9425202535142));
#220714=CARTESIAN_POINT('Ctrl Pts',(-29.2082785712609,68.0744124953734,
62.6552811046037));
#220715=CARTESIAN_POINT('Ctrl Pts',(-29.3059459575509,65.0374518247561,
65.5394024065494));
#220716=CARTESIAN_POINT('Ctrl Pts',(-29.4036133438509,63.1297902918518,
69.2679561845011));
#220717=CARTESIAN_POINT('Ctrl Pts',(-29.5012807301409,62.5676698145191,
73.4182942873752));
#220718=CARTESIAN_POINT('Ctrl Pts',(-29.5989481164309,63.4148092485251,
77.5199574352399));
#220719=CARTESIAN_POINT('Ctrl Pts',(-29.6966155027209,65.5751815719184,
81.1080038707725));
#220720=CARTESIAN_POINT('Ctrl Pts',(-29.7942828890109,68.8038989749744,
83.7757125749618));
#220721=CARTESIAN_POINT('Ctrl Pts',(-29.8919502753009,72.7349719824068,
85.2206869032595));
#220722=CARTESIAN_POINT('Ctrl Pts',(-29.9896176615909,76.9227959878881,
85.2791325899756));
#220723=CARTESIAN_POINT('Ctrl Pts',(-30.0872850478809,80.8926625177431,
83.9444245566036));
#220724=CARTESIAN_POINT('Ctrl Pts',(-30.1849524341709,84.1945695473749,
81.3678578939925));
#220725=CARTESIAN_POINT('Ctrl Pts',(-30.2826198204609,86.4542312318516,
77.8414978909713));
#220726=CARTESIAN_POINT('Ctrl Pts',(-30.3802872067509,87.4155048708503,
73.7650731351128));
#220727=CARTESIAN_POINT('Ctrl Pts',(-30.4779545930409,86.9694258227422,
69.6006644997807));
#220728=CARTESIAN_POINT('Ctrl Pts',(-30.5756219793309,85.1665591312736,
65.820326222327));
#220729=CARTESIAN_POINT('Ctrl Pts',(-30.6732893656209,82.2112677530227,
62.8525764571268));
#220730=CARTESIAN_POINT('Ctrl Pts',(-30.7709567519109,78.4385471074775,
61.0338228372305));
#220731=CARTESIAN_POINT('Ctrl Pts',(-30.8686241382009,74.2760518565624,
60.5702291732061));
#220732=CARTESIAN_POINT('Ctrl Pts',(-30.9662915244909,70.1956193470026,
61.5143458683933));
#220733=CARTESIAN_POINT('Ctrl Pts',(-31.0639589107809,66.6597847488641,
63.7591530970452));
#220734=CARTESIAN_POINT('Ctrl Pts',(-31.1616262970709,64.0693506371989,
67.0501919774508));
#220735=CARTESIAN_POINT('Ctrl Pts',(-31.2592936833609,62.7179542378677,
71.0144086177314));
#220736=CARTESIAN_POINT('Ctrl Pts',(-31.3569610696509,62.7587823422011,
75.2024414334005));
#220737=CARTESIAN_POINT('Ctrl Pts',(-31.4546284559409,64.1872069030099,
79.1395582812057));
#220738=CARTESIAN_POINT('Ctrl Pts',(-31.5522958422309,66.8413096443314,
82.3794694586463));
#220739=CARTESIAN_POINT('Ctrl Pts',(-31.6499632285209,70.4202362180114,
84.5549166263379));
#220740=CARTESIAN_POINT('Ctrl Pts',(-31.7476306148109,74.5182993819421,
85.4193031739153));
#220741=CARTESIAN_POINT('Ctrl Pts',(-31.8452980011009,78.670965452998,84.8746470423662));
#220742=CARTESIAN_POINT('Ctrl Pts',(-31.9429653873909,82.4075112656457,
82.9826874263801));
#220743=CARTESIAN_POINT('Ctrl Pts',(-32.0406327736809,85.304382736349,79.9578863610725));
#220744=CARTESIAN_POINT('Ctrl Pts',(-32.1383001599709,87.0332066010756,
76.1431185004146));
#220745=CARTESIAN_POINT('Ctrl Pts',(-32.2359675462609,87.3980129901441,
71.970804736377));
#220746=CARTESIAN_POINT('Ctrl Pts',(-32.3336349325509,86.357449465044,67.9138954205205));
#220747=CARTESIAN_POINT('Ctrl Pts',(-32.4313023188409,84.0294685736218,
64.4322591422073));
#220748=CARTESIAN_POINT('Ctrl Pts',(-32.5289697051309,80.6779571340673,
61.9205553116033));
#220749=CARTESIAN_POINT('Ctrl Pts',(-32.6266370914209,76.6828244989406,
60.6634950264663));
#220750=CARTESIAN_POINT('Ctrl Pts',(-32.7243044777109,72.4969343775197,
60.8035780069627));
#220751=CARTESIAN_POINT('Ctrl Pts',(-32.8219718640009,68.5947847647611,
62.3249015374696));
#220752=CARTESIAN_POINT('Ctrl Pts',(-32.9196392502909,65.4186690697612,
65.0551052312264));
#220753=CARTESIAN_POINT('Ctrl Pts',(-32.9847508411509,64.025380224545,67.4746207060263));
#220754=CARTESIAN_POINT('Ctrl Pts',(-33.0173066365809,63.5491743972569,
68.7658628636919));
#220755=CARTESIAN_POINT('Ctrl Pts',(-26.9907220242909,87.6342247358637,
73.1516477833508));
#220756=CARTESIAN_POINT('Ctrl Pts',(-27.0232778197209,87.6525780416251,
71.7269606756879));
#220757=CARTESIAN_POINT('Ctrl Pts',(-27.0883894105809,87.2027055493278,
68.8716822599311));
#220758=CARTESIAN_POINT('Ctrl Pts',(-27.1860567968709,85.1446695715054,
65.0551812864947));
#220759=CARTESIAN_POINT('Ctrl Pts',(-27.2837241831609,81.9366891948709,
62.1380783308097));
#220760=CARTESIAN_POINT('Ctrl Pts',(-27.3813915694509,77.9424045170492,
60.4509424484589));
#220761=CARTESIAN_POINT('Ctrl Pts',(-27.4790589557409,73.6145851316153,
60.1850441289509));
#220762=CARTESIAN_POINT('Ctrl Pts',(-27.5767263420309,69.4438087013183,
61.3705171264289));
#220763=CARTESIAN_POINT('Ctrl Pts',(-27.6743937283209,65.9028512572195,
63.8729846813812));
#220764=CARTESIAN_POINT('Ctrl Pts',(-27.7720611146109,63.3930960782151,
67.4087804655588));
#220765=CARTESIAN_POINT('Ctrl Pts',(-27.8697285009009,62.1990350726515,
71.5771064383641));
#220766=CARTESIAN_POINT('Ctrl Pts',(-27.9673958871909,62.4560203657777,
75.9054642787187));
#220767=CARTESIAN_POINT('Ctrl Pts',(-28.0650632734809,64.1349215317246,
79.9032153874961));
#220768=CARTESIAN_POINT('Ctrl Pts',(-28.1627306597709,67.0454276575313,
83.1171968964906));
#220769=CARTESIAN_POINT('Ctrl Pts',(-28.2603980460609,70.8576199312134,
85.1830897102328));
#220770=CARTESIAN_POINT('Ctrl Pts',(-28.3580654323509,75.139369406275,85.8667156913576));
#220771=CARTESIAN_POINT('Ctrl Pts',(-28.4557328186409,79.4053207393797,
85.0905827949681));
#220772=CARTESIAN_POINT('Ctrl Pts',(-28.5534002049309,83.1719093768379,
82.9426691362138));
#220773=CARTESIAN_POINT('Ctrl Pts',(-28.6510675912209,86.012175747098,79.666450279783));
#220774=CARTESIAN_POINT('Ctrl Pts',(-28.7487349775109,87.6041630268346,
75.6333002019379));
#220775=CARTESIAN_POINT('Ctrl Pts',(-28.8464023638009,87.7674123785483,
71.3003943988506));
#220776=CARTESIAN_POINT('Ctrl Pts',(-28.9440697500909,86.4834187622644,
67.1588870111186));
#220777=CARTESIAN_POINT('Ctrl Pts',(-29.0417371363809,83.8977285641353,
63.6782363178493));
#220778=CARTESIAN_POINT('Ctrl Pts',(-29.1394045226709,80.3034412663224,
61.2529895530694));
#220779=CARTESIAN_POINT('Ctrl Pts',(-29.2370719089609,76.1079853173108,
60.1580592223219));
#220780=CARTESIAN_POINT('Ctrl Pts',(-29.3347392952509,71.7869343055323,
60.5175605475774));
#220781=CARTESIAN_POINT('Ctrl Pts',(-29.4324066815409,67.8300985782672,
62.2907424549827));
#220782=CARTESIAN_POINT('Ctrl Pts',(-29.5300740678309,64.6860030606972,
65.2766068902312));
#220783=CARTESIAN_POINT('Ctrl Pts',(-29.6277414541209,62.7110449610938,
69.1366928418758));
#220784=CARTESIAN_POINT('Ctrl Pts',(-29.7254088404109,62.1290945623912,
73.433442402035));
#220785=CARTESIAN_POINT('Ctrl Pts',(-29.8230762267009,63.0061185301486,
77.6797999010284));
#220786=CARTESIAN_POINT('Ctrl Pts',(-29.9207436129909,65.2427022976115,
81.3944218333965));
#220787=CARTESIAN_POINT('Ctrl Pts',(-30.0184109992809,68.5853191489713,
84.1562392846882));
#220788=CARTESIAN_POINT('Ctrl Pts',(-30.1160783855709,72.6550685999751,
85.6521879654061));
#220789=CARTESIAN_POINT('Ctrl Pts',(-30.2137457718609,76.9906264527469,
85.7126954403172));
#220790=CARTESIAN_POINT('Ctrl Pts',(-30.3114131581509,81.1005379450693,
84.3309029180554));
#220791=CARTESIAN_POINT('Ctrl Pts',(-30.4090805444409,84.5189263330808,
81.6634427256689));
#220792=CARTESIAN_POINT('Ctrl Pts',(-30.5067479307309,86.8583020919226,
78.0126833377833));
#220793=CARTESIAN_POINT('Ctrl Pts',(-30.6044153170209,87.8534865764371,
73.7924545654215));
#220794=CARTESIAN_POINT('Ctrl Pts',(-30.7020827033109,87.3916711998821,
69.4811381067028));
#220795=CARTESIAN_POINT('Ctrl Pts',(-30.7997500896009,85.5252047887965,
65.5674408540281));
#220796=CARTESIAN_POINT('Ctrl Pts',(-30.8974174758909,82.4656596108035,
62.4949977946519));
#220797=CARTESIAN_POINT('Ctrl Pts',(-30.9950848621809,78.5598487171896,
60.61208401208));
#220798=CARTESIAN_POINT('Ctrl Pts',(-31.0927522484709,74.2505131413366,
60.1321361566155));
#220799=CARTESIAN_POINT('Ctrl Pts',(-31.1904196347609,70.026135233775,61.1095584519391));
#220800=CARTESIAN_POINT('Ctrl Pts',(-31.2880870210509,66.3655670155455,
63.4335557344115));
#220801=CARTESIAN_POINT('Ctrl Pts',(-31.3857544073409,63.6837501722009,
66.8406925775739));
#220802=CARTESIAN_POINT('Ctrl Pts',(-31.4834217936309,62.2846805686123,
70.9447548692043));
#220803=CARTESIAN_POINT('Ctrl Pts',(-31.5810891799209,62.3269489658028,
75.2805288983569));
#220804=CARTESIAN_POINT('Ctrl Pts',(-31.6787565662109,63.8057640529833,
79.3565353982501));
#220805=CARTESIAN_POINT('Ctrl Pts',(-31.7764239525009,66.5534955639515,
82.7107409066956));
#220806=CARTESIAN_POINT('Ctrl Pts',(-31.8740913387909,70.2586759131592,
84.9629313136325));
#220807=CARTESIAN_POINT('Ctrl Pts',(-31.9717587250809,74.5013064316051,
85.8578108212735));
#220808=CARTESIAN_POINT('Ctrl Pts',(-32.0694261113709,78.8004660836611,
85.2939408579818));
#220809=CARTESIAN_POINT('Ctrl Pts',(-32.1670934976609,82.668826004946,83.335238591712));
#220810=CARTESIAN_POINT('Ctrl Pts',(-32.2647608839509,85.6678903965729,
80.203731633773));
#220811=CARTESIAN_POINT('Ctrl Pts',(-32.3624282702409,87.4577019724425,
76.2543902256493));
#220812=CARTESIAN_POINT('Ctrl Pts',(-32.4600956565309,87.8353776347299,
71.9348897690367));
#220813=CARTESIAN_POINT('Ctrl Pts',(-32.5577630428209,86.7581061551578,
67.7348648827743));
#220814=CARTESIAN_POINT('Ctrl Pts',(-32.6554304291109,84.3480010930265,
64.1304069382318));
#220815=CARTESIAN_POINT('Ctrl Pts',(-32.7530978154009,80.8782584005449,
61.5300977436922));
#220816=CARTESIAN_POINT('Ctrl Pts',(-32.8507652016909,76.7421894906778,
60.2286921489303));
#220817=CARTESIAN_POINT('Ctrl Pts',(-32.9484325879809,72.4086337435891,
60.373716836065));
#220818=CARTESIAN_POINT('Ctrl Pts',(-33.0460999742709,68.3688280177291,
61.9487080894351));
#220819=CARTESIAN_POINT('Ctrl Pts',(-33.1437673605609,65.0806685046385,
64.7752251657534));
#220820=CARTESIAN_POINT('Ctrl Pts',(-33.2088789514209,63.6382286155421,
67.2800938763135));
#220821=CARTESIAN_POINT('Ctrl Pts',(-33.2414347468509,63.1452236775756,
68.616887177359));
#220822=CARTESIAN_POINT('Ctrl Pts',(-27.2148501345709,88.0647351087276,
73.1571937649659));
#220823=CARTESIAN_POINT('Ctrl Pts',(-27.2474059300009,88.0837138021636,
71.6839605382665));
#220824=CARTESIAN_POINT('Ctrl Pts',(-27.3125175208609,87.6185119344257,
68.7313886992027));
#220825=CARTESIAN_POINT('Ctrl Pts',(-27.4101849071509,85.4903485166769,
64.7848407073372));
#220826=CARTESIAN_POINT('Ctrl Pts',(-27.5078522934409,82.1730564207291,
61.7683376612345));
#220827=CARTESIAN_POINT('Ctrl Pts',(-27.6055196797309,78.0426667564991,
60.0237127351951));
#220828=CARTESIAN_POINT('Ctrl Pts',(-27.7031870660209,73.5673772115374,
59.7487539480279));
#220829=CARTESIAN_POINT('Ctrl Pts',(-27.8008544523109,69.2544818500329,
60.9746218595402));
#220830=CARTESIAN_POINT('Ctrl Pts',(-27.8985218386009,65.5928665150491,
63.5623608310333));
#220831=CARTESIAN_POINT('Ctrl Pts',(-27.9961892248909,62.9975915941978,
67.2186386228722));
#220832=CARTESIAN_POINT('Ctrl Pts',(-28.0938566111809,61.7628430387832,
71.5290000277085));
#220833=CARTESIAN_POINT('Ctrl Pts',(-28.1915239974709,62.0285850887952,
76.0048463754076));
#220834=CARTESIAN_POINT('Ctrl Pts',(-28.2891913837609,63.7646947010089,
80.1388205889948));
#220835=CARTESIAN_POINT('Ctrl Pts',(-28.3868587700509,66.774376130688,83.4623183054996));
#220836=CARTESIAN_POINT('Ctrl Pts',(-28.4845261563409,70.7164686041459,
85.5986062803239));
#220837=CARTESIAN_POINT('Ctrl Pts',(-28.5821935426309,75.1441184095806,
86.3055267715799));
#220838=CARTESIAN_POINT('Ctrl Pts',(-28.6798609289209,79.5554317524179,
85.5029471980399));
#220839=CARTESIAN_POINT('Ctrl Pts',(-28.7775283152109,83.4503666487593,
83.281843523324));
#220840=CARTESIAN_POINT('Ctrl Pts',(-28.8751957015009,86.3874149078648,
79.8939877258898));
#220841=CARTESIAN_POINT('Ctrl Pts',(-28.9728630877909,88.0336490489472,
75.7234083257009));
#220842=CARTESIAN_POINT('Ctrl Pts',(-29.0705304740809,88.2024611115288,
71.2428590437401));
#220843=CARTESIAN_POINT('Ctrl Pts',(-29.1681978603709,86.874715497634,66.960230065489));
#220844=CARTESIAN_POINT('Ctrl Pts',(-29.2658652466609,84.200918076899,63.3609764298819));
#220845=CARTESIAN_POINT('Ctrl Pts',(-29.3635326329509,80.4841556769628,
60.8530895418872));
#220846=CARTESIAN_POINT('Ctrl Pts',(-29.4612000192409,76.1457398437741,
59.720849532482));
#220847=CARTESIAN_POINT('Ctrl Pts',(-29.5588674055309,71.6774493043503,
60.0926008416417));
#220848=CARTESIAN_POINT('Ctrl Pts',(-29.6565347918209,67.5857846611909,
61.9262038053416));
#220849=CARTESIAN_POINT('Ctrl Pts',(-29.7542021781109,64.3345542966621,
65.0138113738816));
#220850=CARTESIAN_POINT('Ctrl Pts',(-29.8518695644009,62.2922996303327,
69.0054294992058));
#220851=CARTESIAN_POINT('Ctrl Pts',(-29.9495369506909,61.6905193102603,
73.4485905166492));
#220852=CARTESIAN_POINT('Ctrl Pts',(-30.0472043369809,62.5974278117552,
77.8396423667743));
#220853=CARTESIAN_POINT('Ctrl Pts',(-30.1448717232709,64.9102230232763,
81.6808397959763));
#220854=CARTESIAN_POINT('Ctrl Pts',(-30.2425391095609,68.3667393229248,
84.5367659943965));
#220855=CARTESIAN_POINT('Ctrl Pts',(-30.3402064958509,72.5751652174933,
86.0836890275428));
#220856=CARTESIAN_POINT('Ctrl Pts',(-30.4378738821409,77.0584569175565,
86.1462582906601));
#220857=CARTESIAN_POINT('Ctrl Pts',(-30.5355412684309,81.3084133723522,
84.7173812795337));
#220858=CARTESIAN_POINT('Ctrl Pts',(-30.6332086547209,84.8432831187579,
81.9590275573887));
#220859=CARTESIAN_POINT('Ctrl Pts',(-30.7308760410109,87.2623729519723,
78.183868784647));
#220860=CARTESIAN_POINT('Ctrl Pts',(-30.8285434273009,88.2914682820311,
73.8198359957915));
#220861=CARTESIAN_POINT('Ctrl Pts',(-30.9262108135909,87.8139165770324,
69.361611713678));
#220862=CARTESIAN_POINT('Ctrl Pts',(-31.0238781998809,85.8838504463503,
65.3145554857853));
#220863=CARTESIAN_POINT('Ctrl Pts',(-31.1215455861709,82.7200514686303,
62.1374191322177));
#220864=CARTESIAN_POINT('Ctrl Pts',(-31.2192129724609,78.6811503269562,
60.190345186952));
#220865=CARTESIAN_POINT('Ctrl Pts',(-31.3168803587509,74.2249744261684,
59.694043140027));
#220866=CARTESIAN_POINT('Ctrl Pts',(-31.4145477450409,69.8566511206013,
60.7047710354618));
#220867=CARTESIAN_POINT('Ctrl Pts',(-31.5122151313309,66.0713492822661,
63.1079583717355));
#220868=CARTESIAN_POINT('Ctrl Pts',(-31.6098825176209,63.2981497072342,
66.6311931776472));
#220869=CARTESIAN_POINT('Ctrl Pts',(-31.7075499039109,61.8514068993598,
70.8751011206178));
#220870=CARTESIAN_POINT('Ctrl Pts',(-31.8052172902009,61.8951155893856,
75.3586163632547));
#220871=CARTESIAN_POINT('Ctrl Pts',(-31.9028846764909,63.424321202929,79.5735125152463));
#220872=CARTESIAN_POINT('Ctrl Pts',(-32.0005520627809,66.2656814835311,
83.0420123547065));
#220873=CARTESIAN_POINT('Ctrl Pts',(-32.0982194490709,70.0971156082545,
85.3709460009164));
#220874=CARTESIAN_POINT('Ctrl Pts',(-32.1958868353609,74.4843134812133,
86.2963184686414));
#220875=CARTESIAN_POINT('Ctrl Pts',(-32.2935542216509,78.9299667142801,
85.7132346736073));
#220876=CARTESIAN_POINT('Ctrl Pts',(-32.3912216079409,82.9301407442222,
83.6877897570762));
#220877=CARTESIAN_POINT('Ctrl Pts',(-32.4888889942309,86.0313980567812,
80.4495769065115));
#220878=CARTESIAN_POINT('Ctrl Pts',(-32.5865563805209,87.8821973438042,
76.3656619509229));
#220879=CARTESIAN_POINT('Ctrl Pts',(-32.6842237668109,88.2727422793224,
71.8989748017326));
#220880=CARTESIAN_POINT('Ctrl Pts',(-32.7818911531009,87.1587628452857,
67.5558343450567));
#220881=CARTESIAN_POINT('Ctrl Pts',(-32.8795585393909,84.6665336124505,
63.8285547342752));
#220882=CARTESIAN_POINT('Ctrl Pts',(-32.9772259256809,81.0785596670429,
61.1396401757895));
#220883=CARTESIAN_POINT('Ctrl Pts',(-33.0748933119709,76.8015544824298,
59.7938892714004));
#220884=CARTESIAN_POINT('Ctrl Pts',(-33.1725606982609,72.3203331096696,
59.9438556651612));
#220885=CARTESIAN_POINT('Ctrl Pts',(-33.2702280845509,68.1428712706964,
61.572514641397));
#220886=CARTESIAN_POINT('Ctrl Pts',(-33.3678954708409,64.7426679395154,
64.4953451002813));
#220887=CARTESIAN_POINT('Ctrl Pts',(-33.4330070617009,63.2510770065369,
67.0855670466063));
#220888=CARTESIAN_POINT('Ctrl Pts',(-33.4655628571309,62.7412729578912,
68.4679114910339));
#220889=CARTESIAN_POINT('',(-26.6970235948769,85.8892179113949,68.3402936518988));
#220890=CARTESIAN_POINT('Ctrl Pts',(-22.3657263431209,71.0427934340047,
84.0781567697158));
#220891=CARTESIAN_POINT('Ctrl Pts',(-22.4113638359009,72.7957341079248,
84.7036938863735));
#220892=CARTESIAN_POINT('Ctrl Pts',(-22.5026388214709,76.6021092212285,
85.1071590883939));
#220893=CARTESIAN_POINT('Ctrl Pts',(-22.6395512998309,81.9594314524499,
83.0382494769743));
#220894=CARTESIAN_POINT('Ctrl Pts',(-22.7764637781809,85.7803921824825,
78.7512421293735));
#220895=CARTESIAN_POINT('Ctrl Pts',(-22.9133762565409,87.2221381590131,
73.1924757376221));
#220896=CARTESIAN_POINT('Ctrl Pts',(-23.0502887348909,85.9663418720247,
67.5887670194206));
#220897=CARTESIAN_POINT('Ctrl Pts',(-23.1872012132509,82.2901999352476,
63.1769076868418));
#220898=CARTESIAN_POINT('Ctrl Pts',(-23.3241136916009,77.0050551559994,
60.9306245140911));
#220899=CARTESIAN_POINT('Ctrl Pts',(-23.4610261699609,71.2773803974512,
61.3456896355517));
#220900=CARTESIAN_POINT('Ctrl Pts',(-23.5979386483109,66.3713151444493,
64.3304948862029));
#220901=CARTESIAN_POINT('Ctrl Pts',(-23.7348511266709,63.3696644032273,
69.226271763487));
#220902=CARTESIAN_POINT('Ctrl Pts',(-23.8717636050209,62.9349146157014,
74.9524861359762));
#220903=CARTESIAN_POINT('Ctrl Pts',(-24.0086760833809,65.16301828311,80.2453202044371));
#220904=CARTESIAN_POINT('Ctrl Pts',(-24.1455885617309,69.5622164668703,
83.9366063979647));
#220905=CARTESIAN_POINT('Ctrl Pts',(-24.2825010400909,75.1615736379323,
85.211650591567));
#220906=CARTESIAN_POINT('Ctrl Pts',(-24.4194135184409,80.7252703137354,
83.7890411146378));
#220907=CARTESIAN_POINT('Ctrl Pts',(-24.5563259967909,85.0253575466822,
79.9827583856074));
#220908=CARTESIAN_POINT('Ctrl Pts',(-24.6932384751509,87.1127743256804,
74.6328771144894));
#220909=CARTESIAN_POINT('Ctrl Pts',(-24.8301509535009,86.5268123507618,
68.9201556099781));
#220910=CARTESIAN_POINT('Ctrl Pts',(-24.9670634318609,83.3967977574361,
64.1054337000071));
#220911=CARTESIAN_POINT('Ctrl Pts',(-25.1039759102109,78.4135478836825,
61.251356069971));
#220912=CARTESIAN_POINT('Ctrl Pts',(-25.2408883885709,72.6769027803898,
60.9878387312059));
#220913=CARTESIAN_POINT('Ctrl Pts',(-25.3778008669209,67.4529823927194,
63.37304190929));
#220914=CARTESIAN_POINT('Ctrl Pts',(-25.5147133452809,63.8947445237484,
67.8805336366522));
#220915=CARTESIAN_POINT('Ctrl Pts',(-25.6516258236309,62.787518582008,73.5154772357479));
#220916=CARTESIAN_POINT('Ctrl Pts',(-25.7885383019909,64.3756773943421,
79.034198897657));
#220917=CARTESIAN_POINT('Ctrl Pts',(-25.9254507803409,68.3087030144427,
83.2186765115834));
#220918=CARTESIAN_POINT('Ctrl Pts',(-26.0623632587009,73.7185460237825,
85.1453630258059));
#220919=CARTESIAN_POINT('Ctrl Pts',(-26.1992757370509,79.4112201475916,
84.3890317273548));
#220920=CARTESIAN_POINT('Ctrl Pts',(-26.3361882154009,84.1302876496623,
81.116583535284));
#220921=CARTESIAN_POINT('Ctrl Pts',(-26.4731006937609,86.8342994995147,
76.0503726420501));
#220922=CARTESIAN_POINT('Ctrl Pts',(-26.6100131721109,86.9261467426327,
70.3081733636108));
#220923=CARTESIAN_POINT('Ctrl Pts',(-26.7012881576809,85.2332010925808,
66.8752138971438));
#220924=CARTESIAN_POINT('Ctrl Pts',(-26.7469256504709,84.0408674757396,
65.446074912737));
#220925=CARTESIAN_POINT('Ctrl Pts',(-22.5898544533909,70.8980903883704,
84.4836576545961));
#220926=CARTESIAN_POINT('Ctrl Pts',(-22.6354919461809,72.7151307877147,
85.1320687669442));
#220927=CARTESIAN_POINT('Ctrl Pts',(-22.7267669317509,76.660693497755,85.5502874680715));
#220928=CARTESIAN_POINT('Ctrl Pts',(-22.8636794101009,82.2139167592551,
83.405724105221));
#220929=CARTESIAN_POINT('Ctrl Pts',(-23.0005918884609,86.1745984378018,
78.9619538973823));
#220930=CARTESIAN_POINT('Ctrl Pts',(-23.1375043668109,87.6690646932333,
73.1999202731972));
#220931=CARTESIAN_POINT('Ctrl Pts',(-23.2744168451709,86.3673477436804,
67.3913009179511));
#220932=CARTESIAN_POINT('Ctrl Pts',(-23.4113293235209,82.5567804425581,
62.8181132666061));
#220933=CARTESIAN_POINT('Ctrl Pts',(-23.5482418018809,77.078373943613,60.4896903290828));
#220934=CARTESIAN_POINT('Ctrl Pts',(-23.6851542802309,71.1412554857959,
60.9199331235346));
#220935=CARTESIAN_POINT('Ctrl Pts',(-23.8220667585909,66.0557903019732,
64.0138836520906));
#220936=CARTESIAN_POINT('Ctrl Pts',(-23.9589792369409,62.9443782943297,
69.088684245488));
#220937=CARTESIAN_POINT('Ctrl Pts',(-24.0958917153009,62.493731025262,75.0242889153554));
#220938=CARTESIAN_POINT('Ctrl Pts',(-24.2328041936509,64.8033096880395,
80.5106658775062));
#220939=CARTESIAN_POINT('Ctrl Pts',(-24.3697166720109,69.3633732107457,
84.3369312149315));
#220940=CARTESIAN_POINT('Ctrl Pts',(-24.5066291503609,75.1674818959678,
85.6585999086832));
#220941=CARTESIAN_POINT('Ctrl Pts',(-24.6435416287209,80.9346260897404,
84.1839699166284));
#220942=CARTESIAN_POINT('Ctrl Pts',(-24.7804541070709,85.3919544746771,
80.2385029690767));
#220943=CARTESIAN_POINT('Ctrl Pts',(-24.9173665854309,87.5557017561136,
74.6929927610359));
#220944=CARTESIAN_POINT('Ctrl Pts',(-25.0542790637809,86.9483129284454,
68.7713743524177));
#220945=CARTESIAN_POINT('Ctrl Pts',(-25.1911915421409,83.7038431918362,
63.7805926607207));
#220946=CARTESIAN_POINT('Ctrl Pts',(-25.3281040204909,78.5383709797127,
60.8221500654867));
#220947=CARTESIAN_POINT('Ctrl Pts',(-25.4650164988409,72.591954158844,60.5489966966418));
#220948=CARTESIAN_POINT('Ctrl Pts',(-25.6019289772009,67.177010841838,63.021419522869));
#220949=CARTESIAN_POINT('Ctrl Pts',(-25.7388414555509,63.4886590027825,
67.6937365557131));
#220950=CARTESIAN_POINT('Ctrl Pts',(-25.8757539339109,62.3409451655286,
73.5347329567422));
#220951=CARTESIAN_POINT('Ctrl Pts',(-26.0126664122609,63.9871781302336,
79.2552575367331));
#220952=CARTESIAN_POINT('Ctrl Pts',(-26.1495788906209,68.0640225720935,
83.5927488094103));
#220953=CARTESIAN_POINT('Ctrl Pts',(-26.2864913689709,73.671687137312,85.5898884076403));
#220954=CARTESIAN_POINT('Ctrl Pts',(-26.4234038473309,79.5725250933031,
84.8059003668432));
#220955=CARTESIAN_POINT('Ctrl Pts',(-26.5603163256809,84.4641545854305,
81.4137886666481));
#220956=CARTESIAN_POINT('Ctrl Pts',(-26.6972288040409,87.26704394991,76.1623218021049));
#220957=CARTESIAN_POINT('Ctrl Pts',(-26.8341412823909,87.3622497682239,
70.2101477067447));
#220958=CARTESIAN_POINT('Ctrl Pts',(-26.9254162679609,85.6073982288574,
66.6516553215257));
#220959=CARTESIAN_POINT('Ctrl Pts',(-26.9710537607409,84.3714645868736,
65.1702570576971));
#220960=CARTESIAN_POINT('Ctrl Pts',(-22.8139825636709,70.7533873427582,
84.8891585394854));
#220961=CARTESIAN_POINT('Ctrl Pts',(-22.8596200564509,72.6345274675306,
85.5604436475148));
#220962=CARTESIAN_POINT('Ctrl Pts',(-22.9508950420209,76.7192777743104,
85.9934158477393));
#220963=CARTESIAN_POINT('Ctrl Pts',(-23.0878075203809,82.4684020660794,
83.7731987334476));
#220964=CARTESIAN_POINT('Ctrl Pts',(-23.2247199987309,86.5688046931341,
79.1726656653597));
#220965=CARTESIAN_POINT('Ctrl Pts',(-23.3616324770909,88.1159912274573,
73.207364808737));
#220966=CARTESIAN_POINT('Ctrl Pts',(-23.4985449554409,86.7683536153187,
67.1938348164451));
#220967=CARTESIAN_POINT('Ctrl Pts',(-23.6354574338009,82.8233609498366,
62.4593188463356));
#220968=CARTESIAN_POINT('Ctrl Pts',(-23.7723699121509,77.1516927311802,
60.0487561440661));
#220969=CARTESIAN_POINT('Ctrl Pts',(-23.9092823905109,71.0051305740928,
60.4941766115334));
#220970=CARTESIAN_POINT('Ctrl Pts',(-24.0461948688609,65.7402654594603,
63.697272418015));
#220971=CARTESIAN_POINT('Ctrl Pts',(-24.1831073472209,62.5190921854207,
68.9510967275429));
#220972=CARTESIAN_POINT('Ctrl Pts',(-24.3200198255709,62.0525474348232,
75.0960916947856));
#220973=CARTESIAN_POINT('Ctrl Pts',(-24.4569323039309,64.4436010930036,
80.776011550622));
#220974=CARTESIAN_POINT('Ctrl Pts',(-24.5938447822809,69.164529954672,84.7372560319302));
#220975=CARTESIAN_POINT('Ctrl Pts',(-24.7307572606409,75.1733901540581,
86.1055492258112));
#220976=CARTESIAN_POINT('Ctrl Pts',(-24.8676697389909,81.1439818658025,
84.5788987185907));
#220977=CARTESIAN_POINT('Ctrl Pts',(-25.0045822173509,85.7585514027134,
80.4942475524982));
#220978=CARTESIAN_POINT('Ctrl Pts',(-25.1414946957009,87.9986291865511,
74.7531084075193));
#220979=CARTESIAN_POINT('Ctrl Pts',(-25.2784071740609,87.3698135061078,
68.6225930947988));
#220980=CARTESIAN_POINT('Ctrl Pts',(-25.4153196524109,84.0108886261921,
63.4557516213944));
#220981=CARTESIAN_POINT('Ctrl Pts',(-25.5522321307709,78.6631940756854,
60.3929440609894));
#220982=CARTESIAN_POINT('Ctrl Pts',(-25.6891446091209,72.5070055372434,
60.1101546620874));
#220983=CARTESIAN_POINT('Ctrl Pts',(-25.8260570874809,66.9010392909102,
62.6697971364818));
#220984=CARTESIAN_POINT('Ctrl Pts',(-25.9629695658309,63.0825734817967,
67.5069394748224));
#220985=CARTESIAN_POINT('Ctrl Pts',(-26.0998820441809,61.8943717490509,
73.5539886777849));
#220986=CARTESIAN_POINT('Ctrl Pts',(-26.2367945225409,63.5986788661504,
79.4763161758423));
#220987=CARTESIAN_POINT('Ctrl Pts',(-26.3737070008909,67.8193421297727,
83.9668211072706));
#220988=CARTESIAN_POINT('Ctrl Pts',(-26.5106194792509,73.6248282508795,
86.0344137894687));
#220989=CARTESIAN_POINT('Ctrl Pts',(-26.6475319576009,79.7338300390394,
85.2227690063213));
#220990=CARTESIAN_POINT('Ctrl Pts',(-26.7844444359609,84.7980215212156,
81.7109937979974));
#220991=CARTESIAN_POINT('Ctrl Pts',(-26.9213569143109,87.6997884003007,
76.2742709621448));
#220992=CARTESIAN_POINT('Ctrl Pts',(-27.0582693926709,87.7983527938067,
70.1121220498729));
#220993=CARTESIAN_POINT('Ctrl Pts',(-27.1495443782409,85.9815953651354,
66.4280967459094));
#220994=CARTESIAN_POINT('Ctrl Pts',(-27.1951818710209,84.7020616980161,
64.8944392026497));
#220995=CARTESIAN_POINT('Ctrl Pts',(-23.0381106739509,70.608684297128,85.2946594243566));
#220996=CARTESIAN_POINT('Ctrl Pts',(-23.0837481667309,72.5539241473244,
85.9888185280762));
#220997=CARTESIAN_POINT('Ctrl Pts',(-23.1750231523009,76.7778620508368,
86.4365442274169));
#220998=CARTESIAN_POINT('Ctrl Pts',(-23.3119356306609,82.7228873728753,
84.1406733616905));
#220999=CARTESIAN_POINT('Ctrl Pts',(-23.4488481090109,86.9630109484534,
79.3833774333685));
#221000=CARTESIAN_POINT('Ctrl Pts',(-23.5857605873609,88.5629177616779,
73.2148093443111));
#221001=CARTESIAN_POINT('Ctrl Pts',(-23.7226730657209,87.169359486974,66.9963687149764));
#221002=CARTESIAN_POINT('Ctrl Pts',(-23.8595855440709,83.0899414571462,
62.1005244260996));
#221003=CARTESIAN_POINT('Ctrl Pts',(-23.9964980224309,77.225011518789,59.6078219590666));
#221004=CARTESIAN_POINT('Ctrl Pts',(-24.1334105007809,70.8690056624368,
60.0684200995182));
#221005=CARTESIAN_POINT('Ctrl Pts',(-24.2703229791409,65.4247406169838,
63.3806611839035));
#221006=CARTESIAN_POINT('Ctrl Pts',(-24.4072354574909,62.0938060765228,
68.8135092095446));
#221007=CARTESIAN_POINT('Ctrl Pts',(-24.5441479358509,61.6113638443835,
75.1678944741657));
#221008=CARTESIAN_POINT('Ctrl Pts',(-24.6810604142009,64.0838924979292,
81.0413572237003));
#221009=CARTESIAN_POINT('Ctrl Pts',(-24.8179728925609,68.9656866985482,
85.1375808488973));
#221010=CARTESIAN_POINT('Ctrl Pts',(-24.9548853709109,75.1792984120937,
86.5524985429274));
#221011=CARTESIAN_POINT('Ctrl Pts',(-25.0917978492709,81.3533376418032,
84.9738275205784));
#221012=CARTESIAN_POINT('Ctrl Pts',(-25.2287103276209,86.1251483307086,
80.7499921359666));
#221013=CARTESIAN_POINT('Ctrl Pts',(-25.3656228059809,88.4415566169843,
74.8132240540658));
#221014=CARTESIAN_POINT('Ctrl Pts',(-25.5025352843309,87.7913140837909,
68.4738118372372));
#221015=CARTESIAN_POINT('Ctrl Pts',(-25.6394477626909,84.3179340605874,
63.1309105821169));
#221016=CARTESIAN_POINT('Ctrl Pts',(-25.7763602410409,78.7880171717146,
59.9637380565047));
#221017=CARTESIAN_POINT('Ctrl Pts',(-25.9132727194009,72.4220569156967,
59.6713126275229));
#221018=CARTESIAN_POINT('Ctrl Pts',(-26.0501851977509,66.6250677400192,
62.3181747500578));
#221019=CARTESIAN_POINT('Ctrl Pts',(-26.1870976761109,62.6764879608306,
67.320142393884));
#221020=CARTESIAN_POINT('Ctrl Pts',(-26.3240101544609,61.4477983325716,
73.5732443987792));
#221021=CARTESIAN_POINT('Ctrl Pts',(-26.4609226328209,63.2101796020395,
79.6973748149271));
#221022=CARTESIAN_POINT('Ctrl Pts',(-26.5978351111709,67.5746616874234,
84.3408934050975));
#221023=CARTESIAN_POINT('Ctrl Pts',(-26.7347475895209,73.5779693644099,
86.4789391713035));
#221024=CARTESIAN_POINT('Ctrl Pts',(-26.8716600678809,79.8951349847512,
85.6396376458088));
#221025=CARTESIAN_POINT('Ctrl Pts',(-27.0085725462309,85.1318884569838,
82.0081989293615));
#221026=CARTESIAN_POINT('Ctrl Pts',(-27.1454850245909,88.1325328506964,
76.3862201221988));
#221027=CARTESIAN_POINT('Ctrl Pts',(-27.2823975029409,88.2344558193887,
70.0140963930029));
#221028=CARTESIAN_POINT('Ctrl Pts',(-27.3736724885109,86.3557925014101,
66.2045381702959));
#221029=CARTESIAN_POINT('Ctrl Pts',(-27.4193099813009,85.032658809151,64.6186213476101));
#221030=CARTESIAN_POINT('',(-22.5674166601918,77.7863349909178,84.4952548267707));
#221031=CARTESIAN_POINT('Ctrl Pts',(-22.5675364832709,77.7863942292111,
84.4954770366417));
#221032=CARTESIAN_POINT('Ctrl Pts',(-22.5675364832709,77.2378487361899,
84.6563729599099));
#221033=CARTESIAN_POINT('Ctrl Pts',(-22.5675364832727,76.6778394979494,
84.7774848925877));
#221034=CARTESIAN_POINT('Ctrl Pts',(-22.5675364832727,75.5395172400914,
84.936908357079));
#221035=CARTESIAN_POINT('Ctrl Pts',(-22.5675364832709,74.9641682946092,
84.9749462493134));
#221036=CARTESIAN_POINT('Ctrl Pts',(-22.5675364832709,74.3890417160681,
84.9719151100471));
#221037=CARTESIAN_POINT('Ctrl Pts',(-22.5674166601918,77.7862809883271,
84.4950313516973));
#221038=CARTESIAN_POINT('Ctrl Pts',(-22.5674566012175,77.7893705430951,
84.4942847630104));
#221039=CARTESIAN_POINT('Ctrl Pts',(-22.5674965422431,77.7924597972905,
84.4935369402494));
#221040=CARTESIAN_POINT('Ctrl Pts',(-22.5675364832687,77.7955487498965,
84.4927878836051));
#221041=CARTESIAN_POINT('Origin',(-21.6548258024609,75.,72.9888893865801));
#221042=CARTESIAN_POINT('Ctrl Pts',(-25.6386080251009,88.0647351087276,
73.1571937649659));
#221043=CARTESIAN_POINT('Ctrl Pts',(-25.6711638205309,88.0837138021636,
71.6839605382665));
#221044=CARTESIAN_POINT('Ctrl Pts',(-25.7362754113909,87.6185119344257,
68.7313886992027));
#221045=CARTESIAN_POINT('Ctrl Pts',(-25.8339427976809,85.4903485166769,
64.7848407073372));
#221046=CARTESIAN_POINT('Ctrl Pts',(-25.9316101839709,82.1730564207291,
61.7683376612345));
#221047=CARTESIAN_POINT('Ctrl Pts',(-26.0292775702609,78.0426667564991,
60.0237127351951));
#221048=CARTESIAN_POINT('Ctrl Pts',(-26.1269449565509,73.5673772115374,
59.7487539480279));
#221049=CARTESIAN_POINT('Ctrl Pts',(-26.2246123428409,69.2544818500329,
60.9746218595402));
#221050=CARTESIAN_POINT('Ctrl Pts',(-26.3222797291309,65.5928665150491,
63.5623608310333));
#221051=CARTESIAN_POINT('Ctrl Pts',(-26.4199471154209,62.9975915941978,
67.2186386228722));
#221052=CARTESIAN_POINT('Ctrl Pts',(-26.5176145017109,61.7628430387832,
71.5290000277085));
#221053=CARTESIAN_POINT('Ctrl Pts',(-26.6152818880009,62.0285850887952,
76.0048463754076));
#221054=CARTESIAN_POINT('Ctrl Pts',(-26.7129492742909,63.7646947010089,
80.1388205889948));
#221055=CARTESIAN_POINT('Ctrl Pts',(-26.8106166605809,66.774376130688,83.4623183054996));
#221056=CARTESIAN_POINT('Ctrl Pts',(-26.9082840468709,70.7164686041459,
85.5986062803239));
#221057=CARTESIAN_POINT('Ctrl Pts',(-27.0059514331609,75.1441184095806,
86.3055267715799));
#221058=CARTESIAN_POINT('Ctrl Pts',(-27.1036188194509,79.5554317524179,
85.5029471980399));
#221059=CARTESIAN_POINT('Ctrl Pts',(-27.2012862057409,83.4503666487593,
83.281843523324));
#221060=CARTESIAN_POINT('Ctrl Pts',(-27.2989535920309,86.3874149078648,
79.8939877258898));
#221061=CARTESIAN_POINT('Ctrl Pts',(-27.3966209783209,88.0336490489472,
75.7234083257009));
#221062=CARTESIAN_POINT('Ctrl Pts',(-27.4942883646109,88.2024611115288,
71.2428590437401));
#221063=CARTESIAN_POINT('Ctrl Pts',(-27.5919557509009,86.874715497634,66.960230065489));
#221064=CARTESIAN_POINT('Ctrl Pts',(-27.6896231371909,84.200918076899,63.3609764298819));
#221065=CARTESIAN_POINT('Ctrl Pts',(-27.7872905234809,80.4841556769628,
60.8530895418872));
#221066=CARTESIAN_POINT('Ctrl Pts',(-27.8849579097709,76.1457398437741,
59.720849532482));
#221067=CARTESIAN_POINT('Ctrl Pts',(-27.9826252960609,71.6774493043503,
60.0926008416417));
#221068=CARTESIAN_POINT('Ctrl Pts',(-28.0802926823509,67.5857846611909,
61.9262038053416));
#221069=CARTESIAN_POINT('Ctrl Pts',(-28.1779600686409,64.3345542966621,
65.0138113738816));
#221070=CARTESIAN_POINT('Ctrl Pts',(-28.2756274549309,62.2922996303327,
69.0054294992058));
#221071=CARTESIAN_POINT('Ctrl Pts',(-28.3732948412209,61.6905193102603,
73.4485905166492));
#221072=CARTESIAN_POINT('Ctrl Pts',(-28.4709622275109,62.5974278117552,
77.8396423667743));
#221073=CARTESIAN_POINT('Ctrl Pts',(-28.5686296138009,64.9102230232763,
81.6808397959763));
#221074=CARTESIAN_POINT('Ctrl Pts',(-28.6662970000909,68.3667393229248,
84.5367659943965));
#221075=CARTESIAN_POINT('Ctrl Pts',(-28.7639643863809,72.5751652174933,
86.0836890275428));
#221076=CARTESIAN_POINT('Ctrl Pts',(-28.8616317726709,77.0584569175565,
86.1462582906601));
#221077=CARTESIAN_POINT('Ctrl Pts',(-28.9592991589609,81.3084133723522,
84.7173812795337));
#221078=CARTESIAN_POINT('Ctrl Pts',(-29.0569665452509,84.8432831187579,
81.9590275573887));
#221079=CARTESIAN_POINT('Ctrl Pts',(-29.1546339315409,87.2623729519723,
78.183868784647));
#221080=CARTESIAN_POINT('Ctrl Pts',(-29.2523013178309,88.2914682820311,
73.8198359957915));
#221081=CARTESIAN_POINT('Ctrl Pts',(-29.3499687041209,87.8139165770324,
69.361611713678));
#221082=CARTESIAN_POINT('Ctrl Pts',(-29.4476360904109,85.8838504463503,
65.3145554857853));
#221083=CARTESIAN_POINT('Ctrl Pts',(-29.5453034767009,82.7200514686303,
62.1374191322177));
#221084=CARTESIAN_POINT('Ctrl Pts',(-29.6429708629909,78.6811503269562,
60.190345186952));
#221085=CARTESIAN_POINT('Ctrl Pts',(-29.7406382492809,74.2249744261684,
59.694043140027));
#221086=CARTESIAN_POINT('Ctrl Pts',(-29.8383056355709,69.8566511206013,
60.7047710354618));
#221087=CARTESIAN_POINT('Ctrl Pts',(-29.9359730218609,66.0713492822661,
63.1079583717355));
#221088=CARTESIAN_POINT('Ctrl Pts',(-30.0336404081509,63.2981497072342,
66.6311931776472));
#221089=CARTESIAN_POINT('Ctrl Pts',(-30.1313077944409,61.8514068993598,
70.8751011206178));
#221090=CARTESIAN_POINT('Ctrl Pts',(-30.2289751807309,61.8951155893856,
75.3586163632547));
#221091=CARTESIAN_POINT('Ctrl Pts',(-30.3266425670209,63.424321202929,79.5735125152463));
#221092=CARTESIAN_POINT('Ctrl Pts',(-30.4243099533109,66.2656814835311,
83.0420123547065));
#221093=CARTESIAN_POINT('Ctrl Pts',(-30.5219773396009,70.0971156082545,
85.3709460009164));
#221094=CARTESIAN_POINT('Ctrl Pts',(-30.6196447258909,74.4843134812133,
86.2963184686414));
#221095=CARTESIAN_POINT('Ctrl Pts',(-30.7173121121809,78.9299667142801,
85.7132346736073));
#221096=CARTESIAN_POINT('Ctrl Pts',(-30.8149794984709,82.9301407442222,
83.6877897570762));
#221097=CARTESIAN_POINT('Ctrl Pts',(-30.9126468847609,86.0313980567812,
80.4495769065115));
#221098=CARTESIAN_POINT('Ctrl Pts',(-31.0103142710509,87.8821973438046,
76.3656619509219));
#221099=CARTESIAN_POINT('Ctrl Pts',(-31.1079816573409,88.2727422793224,
71.8989748017326));
#221100=CARTESIAN_POINT('Ctrl Pts',(-31.2056490436309,87.1587628452857,
67.5558343450567));
#221101=CARTESIAN_POINT('Ctrl Pts',(-31.3033164299209,84.6665336124505,
63.8285547342752));
#221102=CARTESIAN_POINT('Ctrl Pts',(-31.4009838162109,81.0785596670429,
61.1396401757895));
#221103=CARTESIAN_POINT('Ctrl Pts',(-31.4986512025009,76.8015544824298,
59.7938892714004));
#221104=CARTESIAN_POINT('Ctrl Pts',(-31.5963185887909,72.3203331096696,
59.9438556651612));
#221105=CARTESIAN_POINT('Ctrl Pts',(-31.6939859750809,68.1428712706964,
61.572514641397));
#221106=CARTESIAN_POINT('Ctrl Pts',(-31.7916533613709,64.7426679395154,
64.4953451002813));
#221107=CARTESIAN_POINT('Ctrl Pts',(-31.8567649522309,63.2510770065369,
67.0855670466063));
#221108=CARTESIAN_POINT('Ctrl Pts',(-31.8893207476609,62.7412729578912,
68.4679114910339));
#221109=CARTESIAN_POINT('Ctrl Pts',(-25.8627361353809,87.6342247358637,
73.1516477833508));
#221110=CARTESIAN_POINT('Ctrl Pts',(-25.8952919308109,87.6525780416251,
71.7269606756879));
#221111=CARTESIAN_POINT('Ctrl Pts',(-25.9604035216709,87.2027055493278,
68.8716822599311));
#221112=CARTESIAN_POINT('Ctrl Pts',(-26.0580709079509,85.1446695715054,
65.0551812864947));
#221113=CARTESIAN_POINT('Ctrl Pts',(-26.1557382942409,81.9366891948709,
62.1380783308097));
#221114=CARTESIAN_POINT('Ctrl Pts',(-26.2534056805309,77.9424045170492,
60.4509424484589));
#221115=CARTESIAN_POINT('Ctrl Pts',(-26.3510730668209,73.6145851316153,
60.1850441289509));
#221116=CARTESIAN_POINT('Ctrl Pts',(-26.4487404531109,69.4438087013183,
61.3705171264289));
#221117=CARTESIAN_POINT('Ctrl Pts',(-26.5464078394009,65.9028512572195,
63.8729846813812));
#221118=CARTESIAN_POINT('Ctrl Pts',(-26.6440752256909,63.3930960782151,
67.4087804655588));
#221119=CARTESIAN_POINT('Ctrl Pts',(-26.7417426119809,62.1990350726515,
71.5771064383641));
#221120=CARTESIAN_POINT('Ctrl Pts',(-26.8394099982709,62.4560203657777,
75.9054642787187));
#221121=CARTESIAN_POINT('Ctrl Pts',(-26.9370773845609,64.1349215317246,
79.9032153874961));
#221122=CARTESIAN_POINT('Ctrl Pts',(-27.0347447708509,67.0454276575313,
83.1171968964906));
#221123=CARTESIAN_POINT('Ctrl Pts',(-27.1324121571409,70.8576199312134,
85.1830897102328));
#221124=CARTESIAN_POINT('Ctrl Pts',(-27.2300795434309,75.139369406275,85.8667156913576));
#221125=CARTESIAN_POINT('Ctrl Pts',(-27.3277469297209,79.4053207393797,
85.0905827949681));
#221126=CARTESIAN_POINT('Ctrl Pts',(-27.4254143160109,83.1719093768379,
82.9426691362138));
#221127=CARTESIAN_POINT('Ctrl Pts',(-27.5230817023009,86.0121757470976,
79.666450279784));
#221128=CARTESIAN_POINT('Ctrl Pts',(-27.6207490885909,87.6041630268346,
75.6333002019379));
#221129=CARTESIAN_POINT('Ctrl Pts',(-27.7184164748809,87.7674123785483,
71.3003943988506));
#221130=CARTESIAN_POINT('Ctrl Pts',(-27.8160838611709,86.4834187622644,
67.1588870111186));
#221131=CARTESIAN_POINT('Ctrl Pts',(-27.9137512474609,83.8977285641353,
63.6782363178493));
#221132=CARTESIAN_POINT('Ctrl Pts',(-28.0114186337509,80.3034412663224,
61.2529895530694));
#221133=CARTESIAN_POINT('Ctrl Pts',(-28.1090860200409,76.1079853173108,
60.1580592223219));
#221134=CARTESIAN_POINT('Ctrl Pts',(-28.2067534063309,71.7869343055323,
60.5175605475774));
#221135=CARTESIAN_POINT('Ctrl Pts',(-28.3044207926209,67.8300985782672,
62.2907424549827));
#221136=CARTESIAN_POINT('Ctrl Pts',(-28.4020881789109,64.6860030606972,
65.2766068902312));
#221137=CARTESIAN_POINT('Ctrl Pts',(-28.4997555652109,62.7110449610938,
69.1366928418758));
#221138=CARTESIAN_POINT('Ctrl Pts',(-28.5974229515009,62.1290945623912,
73.433442402035));
#221139=CARTESIAN_POINT('Ctrl Pts',(-28.6950903377909,63.0061185301486,
77.6797999010284));
#221140=CARTESIAN_POINT('Ctrl Pts',(-28.7927577240809,65.2427022976115,
81.3944218333965));
#221141=CARTESIAN_POINT('Ctrl Pts',(-28.8904251103709,68.5853191489713,
84.1562392846882));
#221142=CARTESIAN_POINT('Ctrl Pts',(-28.9880924966609,72.6550685999751,
85.6521879654061));
#221143=CARTESIAN_POINT('Ctrl Pts',(-29.0857598829509,76.9906264527469,
85.7126954403172));
#221144=CARTESIAN_POINT('Ctrl Pts',(-29.1834272692409,81.1005379450693,
84.3309029180554));
#221145=CARTESIAN_POINT('Ctrl Pts',(-29.2810946555309,84.5189263330808,
81.6634427256689));
#221146=CARTESIAN_POINT('Ctrl Pts',(-29.3787620418209,86.8583020919226,
78.0126833377833));
#221147=CARTESIAN_POINT('Ctrl Pts',(-29.4764294281109,87.8534865764371,
73.7924545654215));
#221148=CARTESIAN_POINT('Ctrl Pts',(-29.5740968144009,87.3916711998821,
69.4811381067028));
#221149=CARTESIAN_POINT('Ctrl Pts',(-29.6717642006909,85.5252047887965,
65.5674408540281));
#221150=CARTESIAN_POINT('Ctrl Pts',(-29.7694315869809,82.4656596108035,
62.4949977946519));
#221151=CARTESIAN_POINT('Ctrl Pts',(-29.8670989732709,78.5598487171896,
60.61208401208));
#221152=CARTESIAN_POINT('Ctrl Pts',(-29.9647663595609,74.2505131413366,
60.1321361566155));
#221153=CARTESIAN_POINT('Ctrl Pts',(-30.0624337458509,70.026135233775,61.1095584519391));
#221154=CARTESIAN_POINT('Ctrl Pts',(-30.1601011321409,66.3655670155455,
63.4335557344115));
#221155=CARTESIAN_POINT('Ctrl Pts',(-30.2577685184309,63.6837501722009,
66.8406925775739));
#221156=CARTESIAN_POINT('Ctrl Pts',(-30.3554359047209,62.2846805686123,
70.9447548692043));
#221157=CARTESIAN_POINT('Ctrl Pts',(-30.4531032910109,62.3269489658028,
75.2805288983569));
#221158=CARTESIAN_POINT('Ctrl Pts',(-30.5507706773009,63.8057640529833,
79.3565353982501));
#221159=CARTESIAN_POINT('Ctrl Pts',(-30.6484380635909,66.5534955639515,
82.7107409066956));
#221160=CARTESIAN_POINT('Ctrl Pts',(-30.7461054498809,70.2586759131591,
84.9629313136325));
#221161=CARTESIAN_POINT('Ctrl Pts',(-30.8437728361709,74.5013064316051,
85.8578108212735));
#221162=CARTESIAN_POINT('Ctrl Pts',(-30.9414402224609,78.8004660836611,
85.2939408579818));
#221163=CARTESIAN_POINT('Ctrl Pts',(-31.0391076087509,82.668826004946,83.335238591712));
#221164=CARTESIAN_POINT('Ctrl Pts',(-31.1367749950409,85.6678903965733,
80.2037316337721));
#221165=CARTESIAN_POINT('Ctrl Pts',(-31.2344423813309,87.4577019724425,
76.2543902256493));
#221166=CARTESIAN_POINT('Ctrl Pts',(-31.3321097676209,87.8353776347299,
71.9348897690367));
#221167=CARTESIAN_POINT('Ctrl Pts',(-31.4297771539109,86.7581061551578,
67.7348648827743));
#221168=CARTESIAN_POINT('Ctrl Pts',(-31.5274445402009,84.3480010930265,
64.1304069382318));
#221169=CARTESIAN_POINT('Ctrl Pts',(-31.6251119264909,80.8782584005449,
61.5300977436922));
#221170=CARTESIAN_POINT('Ctrl Pts',(-31.7227793127809,76.7421894906778,
60.2286921489303));
#221171=CARTESIAN_POINT('Ctrl Pts',(-31.8204466990709,72.4086337435891,
60.373716836065));
#221172=CARTESIAN_POINT('Ctrl Pts',(-31.9181140853609,68.3688280177291,
61.9487080894351));
#221173=CARTESIAN_POINT('Ctrl Pts',(-32.0157814716509,65.0806685046385,
64.7752251657534));
#221174=CARTESIAN_POINT('Ctrl Pts',(-32.0808930625109,63.6382286155421,
67.2800938763135));
#221175=CARTESIAN_POINT('Ctrl Pts',(-32.1134488579409,63.1452236775756,
68.616887177359));
#221176=CARTESIAN_POINT('Ctrl Pts',(-26.0868642456509,87.2037143630092,
73.1461018017395));
#221177=CARTESIAN_POINT('Ctrl Pts',(-26.1194200410809,87.2214422810865,
71.7699608131094));
#221178=CARTESIAN_POINT('Ctrl Pts',(-26.1845316319409,86.7868991642302,
69.0119758206587));
#221179=CARTESIAN_POINT('Ctrl Pts',(-26.2821990182309,84.7989906263339,
65.3255218656522));
#221180=CARTESIAN_POINT('Ctrl Pts',(-26.3798664045209,81.7003219690098,
62.5078190003946));
#221181=CARTESIAN_POINT('Ctrl Pts',(-26.4775337908109,77.8421422775993,
60.8781721617227));
#221182=CARTESIAN_POINT('Ctrl Pts',(-26.5752011771009,73.6617930516903,
60.6213343098834));
#221183=CARTESIAN_POINT('Ctrl Pts',(-26.6728685633909,69.6331355526051,
61.766412393317));
#221184=CARTESIAN_POINT('Ctrl Pts',(-26.7705359496809,66.212835999391,64.1836085317264));
#221185=CARTESIAN_POINT('Ctrl Pts',(-26.8682033359709,63.7886005622341,
67.5989223082414));
#221186=CARTESIAN_POINT('Ctrl Pts',(-26.9658707222609,62.6352271065125,
71.6252128490112));
#221187=CARTESIAN_POINT('Ctrl Pts',(-27.0635381085509,62.8834556427626,
75.8060821820242));
#221188=CARTESIAN_POINT('Ctrl Pts',(-27.1612054948409,64.5051483624386,
79.6676101859859));
#221189=CARTESIAN_POINT('Ctrl Pts',(-27.2588728811309,67.3164791843653,
82.7720754874778));
#221190=CARTESIAN_POINT('Ctrl Pts',(-27.3565402674209,70.9987712582735,
84.767573140128));
#221191=CARTESIAN_POINT('Ctrl Pts',(-27.4542076537109,75.1346204029575,
85.4279046111303));
#221192=CARTESIAN_POINT('Ctrl Pts',(-27.5518750400009,79.2552097263266,
84.678218391901));
#221193=CARTESIAN_POINT('Ctrl Pts',(-27.6495424262909,82.8934521049011,
82.6034947491146));
#221194=CARTESIAN_POINT('Ctrl Pts',(-27.7472098125809,85.6369365863143,
79.4389128336909));
#221195=CARTESIAN_POINT('Ctrl Pts',(-27.8448771988709,87.1746770047232,
75.5431920781981));
#221196=CARTESIAN_POINT('Ctrl Pts',(-27.9425445851609,87.3323636455694,
71.3579297539834));
#221197=CARTESIAN_POINT('Ctrl Pts',(-28.0402119714509,86.0921220269066,
67.3575439567694));
#221198=CARTESIAN_POINT('Ctrl Pts',(-28.1378793577409,83.5945390513956,
63.9954962058266));
#221199=CARTESIAN_POINT('Ctrl Pts',(-28.2355467440309,80.1227268557061,
61.6528895642724));
#221200=CARTESIAN_POINT('Ctrl Pts',(-28.3332141303209,76.0702307908808,
60.5952689121648));
#221201=CARTESIAN_POINT('Ctrl Pts',(-28.4308815166109,71.8964193067431,
60.9425202535142));
#221202=CARTESIAN_POINT('Ctrl Pts',(-28.5285489029009,68.0744124953734,
62.6552811046037));
#221203=CARTESIAN_POINT('Ctrl Pts',(-28.6262162891909,65.0374518247561,
65.5394024065494));
#221204=CARTESIAN_POINT('Ctrl Pts',(-28.7238836754809,63.1297902918518,
69.2679561845011));
#221205=CARTESIAN_POINT('Ctrl Pts',(-28.8215510617709,62.5676698145191,
73.4182942873752));
#221206=CARTESIAN_POINT('Ctrl Pts',(-28.9192184480609,63.4148092485251,
77.5199574352399));
#221207=CARTESIAN_POINT('Ctrl Pts',(-29.0168858343509,65.5751815719184,
81.1080038707725));
#221208=CARTESIAN_POINT('Ctrl Pts',(-29.1145532206409,68.8038989749744,
83.7757125749618));
#221209=CARTESIAN_POINT('Ctrl Pts',(-29.2122206069309,72.7349719824068,
85.2206869032595));
#221210=CARTESIAN_POINT('Ctrl Pts',(-29.3098879932209,76.9227959878881,
85.2791325899756));
#221211=CARTESIAN_POINT('Ctrl Pts',(-29.4075553795109,80.8926625177431,
83.9444245566036));
#221212=CARTESIAN_POINT('Ctrl Pts',(-29.5052227658009,84.1945695473749,
81.3678578939925));
#221213=CARTESIAN_POINT('Ctrl Pts',(-29.6028901520909,86.4542312318516,
77.8414978909713));
#221214=CARTESIAN_POINT('Ctrl Pts',(-29.7005575383809,87.4155048708503,
73.7650731351128));
#221215=CARTESIAN_POINT('Ctrl Pts',(-29.7982249246709,86.9694258227422,
69.6006644997807));
#221216=CARTESIAN_POINT('Ctrl Pts',(-29.8958923109609,85.1665591312736,
65.820326222327));
#221217=CARTESIAN_POINT('Ctrl Pts',(-29.9935596972509,82.2112677530227,
62.8525764571268));
#221218=CARTESIAN_POINT('Ctrl Pts',(-30.0912270835409,78.4385471074775,
61.0338228372305));
#221219=CARTESIAN_POINT('Ctrl Pts',(-30.1888944698309,74.2760518565624,
60.5702291732061));
#221220=CARTESIAN_POINT('Ctrl Pts',(-30.2865618561209,70.1956193470026,
61.5143458683933));
#221221=CARTESIAN_POINT('Ctrl Pts',(-30.3842292424109,66.6597847488641,
63.7591530970452));
#221222=CARTESIAN_POINT('Ctrl Pts',(-30.4818966287009,64.0693506371989,
67.0501919774508));
#221223=CARTESIAN_POINT('Ctrl Pts',(-30.5795640149909,62.7179542378677,
71.0144086177314));
#221224=CARTESIAN_POINT('Ctrl Pts',(-30.6772314012809,62.7587823422011,
75.2024414334005));
#221225=CARTESIAN_POINT('Ctrl Pts',(-30.7748987875709,64.1872069030099,
79.1395582812057));
#221226=CARTESIAN_POINT('Ctrl Pts',(-30.8725661738609,66.8413096443314,
82.3794694586463));
#221227=CARTESIAN_POINT('Ctrl Pts',(-30.9702335601509,70.4202362180114,
84.5549166263379));
#221228=CARTESIAN_POINT('Ctrl Pts',(-31.0679009464409,74.5182993819421,
85.4193031739153));
#221229=CARTESIAN_POINT('Ctrl Pts',(-31.1655683327309,78.670965452998,84.8746470423662));
#221230=CARTESIAN_POINT('Ctrl Pts',(-31.2632357190209,82.4075112656457,
82.9826874263801));
#221231=CARTESIAN_POINT('Ctrl Pts',(-31.3609031053109,85.304382736349,79.9578863610725));
#221232=CARTESIAN_POINT('Ctrl Pts',(-31.4585704916009,87.0332066010756,
76.1431185004146));
#221233=CARTESIAN_POINT('Ctrl Pts',(-31.5562378778909,87.3980129901441,
71.970804736377));
#221234=CARTESIAN_POINT('Ctrl Pts',(-31.6539052641809,86.357449465044,67.9138954205205));
#221235=CARTESIAN_POINT('Ctrl Pts',(-31.7515726504709,84.0294685736218,
64.4322591422073));
#221236=CARTESIAN_POINT('Ctrl Pts',(-31.8492400367609,80.6779571340673,
61.9205553116033));
#221237=CARTESIAN_POINT('Ctrl Pts',(-31.9469074230509,76.6828244989406,
60.6634950264663));
#221238=CARTESIAN_POINT('Ctrl Pts',(-32.0445748093409,72.4969343775197,
60.8035780069627));
#221239=CARTESIAN_POINT('Ctrl Pts',(-32.1422421956309,68.5947847647611,
62.3249015374696));
#221240=CARTESIAN_POINT('Ctrl Pts',(-32.2399095819209,65.4186690697612,
65.0551052312264));
#221241=CARTESIAN_POINT('Ctrl Pts',(-32.3050211727809,64.025380224545,67.4746207060263));
#221242=CARTESIAN_POINT('Ctrl Pts',(-32.3375769682109,63.5491743972569,
68.7658628636919));
#221243=CARTESIAN_POINT('Ctrl Pts',(-26.3109923559309,86.773203990145,73.1405558201253));
#221244=CARTESIAN_POINT('Ctrl Pts',(-26.3435481513609,86.7903065205387,
71.812960950527));
#221245=CARTESIAN_POINT('Ctrl Pts',(-26.4086597422209,86.3710927791314,
69.1522693813868));
#221246=CARTESIAN_POINT('Ctrl Pts',(-26.5063271285109,84.4533116811586,
65.595862444819));
#221247=CARTESIAN_POINT('Ctrl Pts',(-26.6039945148009,81.4639547431525,
62.8775596699702));
#221248=CARTESIAN_POINT('Ctrl Pts',(-26.7016619010909,77.7418800381493,
61.3054018749864));
#221249=CARTESIAN_POINT('Ctrl Pts',(-26.7993292873809,73.7090009717682,
61.0576244908064));
#221250=CARTESIAN_POINT('Ctrl Pts',(-26.8969966736709,69.8224624038905,
62.1623076602057));
#221251=CARTESIAN_POINT('Ctrl Pts',(-26.9946640599609,66.5228207415521,
64.4942323820705));
#221252=CARTESIAN_POINT('Ctrl Pts',(-27.0923314462509,64.1841050462514,
67.789064150928));
#221253=CARTESIAN_POINT('Ctrl Pts',(-27.1899988325409,63.0714191403804,
71.6733192596676));
#221254=CARTESIAN_POINT('Ctrl Pts',(-27.2876662188309,63.3108909197464,
75.7067000853347));
#221255=CARTESIAN_POINT('Ctrl Pts',(-27.3853336051209,64.8753751931555,
79.4320049844844));
#221256=CARTESIAN_POINT('Ctrl Pts',(-27.4830009914109,67.5875307112038,
82.4269540784776));
#221257=CARTESIAN_POINT('Ctrl Pts',(-27.5806683777009,71.139922585341,84.3520565700369));
#221258=CARTESIAN_POINT('Ctrl Pts',(-27.6783357639909,75.129871399649,84.9890935309176));
#221259=CARTESIAN_POINT('Ctrl Pts',(-27.7760031502809,79.1050987132879,
84.2658539888279));
#221260=CARTESIAN_POINT('Ctrl Pts',(-27.8736705365709,82.6149948329797,
82.2643203620044));
#221261=CARTESIAN_POINT('Ctrl Pts',(-27.9713379228609,85.2616974255471,
79.211375387585));
#221262=CARTESIAN_POINT('Ctrl Pts',(-28.0690053091509,86.745190982611,75.4530839544341));
#221263=CARTESIAN_POINT('Ctrl Pts',(-28.1666726954409,86.8973149125801,
71.4154651090891));
#221264=CARTESIAN_POINT('Ctrl Pts',(-28.2643400817309,85.7008252915377,
67.5562009023972));
#221265=CARTESIAN_POINT('Ctrl Pts',(-28.3620074680209,83.2913495386348,
64.3127560937844));
#221266=CARTESIAN_POINT('Ctrl Pts',(-28.4596748543109,79.9420124450654,
62.0527895754545));
#221267=CARTESIAN_POINT('Ctrl Pts',(-28.5573422406009,76.0324762644166,
61.0324786020043));
#221268=CARTESIAN_POINT('Ctrl Pts',(-28.6550096268909,72.005904307922,61.367479959455));
#221269=CARTESIAN_POINT('Ctrl Pts',(-28.7526770131809,68.3187264124431,
63.0198197542422));
#221270=CARTESIAN_POINT('Ctrl Pts',(-28.8503443994709,65.3889005887908,
65.8021979228998));
#221271=CARTESIAN_POINT('Ctrl Pts',(-28.9480117857609,63.5485356226125,
69.399219527172));
#221272=CARTESIAN_POINT('Ctrl Pts',(-29.0456791720509,63.00624506665,73.403146172761));
#221273=CARTESIAN_POINT('Ctrl Pts',(-29.1433465583409,63.823499966919,77.3601149694953));
#221274=CARTESIAN_POINT('Ctrl Pts',(-29.2410139446309,65.9076608462574,
80.8215859081835));
#221275=CARTESIAN_POINT('Ctrl Pts',(-29.3386813309209,69.0224788010218,
83.3951858652539));
#221276=CARTESIAN_POINT('Ctrl Pts',(-29.4363487172109,72.8148753648847,
84.789185841132));
#221277=CARTESIAN_POINT('Ctrl Pts',(-29.5340161035009,76.8549655230795,
84.8455697396331));
#221278=CARTESIAN_POINT('Ctrl Pts',(-29.6316834897909,80.6847870904639,
83.5579461951268));
#221279=CARTESIAN_POINT('Ctrl Pts',(-29.7293508760809,83.8702127616981,
81.0722730622719));
#221280=CARTESIAN_POINT('Ctrl Pts',(-29.8270182623709,86.0501603718022,
77.6703124441068));
#221281=CARTESIAN_POINT('Ctrl Pts',(-29.9246856486609,86.9775231652655,
73.7376917047466));
#221282=CARTESIAN_POINT('Ctrl Pts',(-30.0223530349509,86.5471804455886,
69.720190892803));
#221283=CARTESIAN_POINT('Ctrl Pts',(-30.1200204212409,84.8079134737197,
66.0732115905698));
#221284=CARTESIAN_POINT('Ctrl Pts',(-30.2176878075309,81.956875895195,63.2101551195606));
#221285=CARTESIAN_POINT('Ctrl Pts',(-30.3153551938209,78.3172454977062,
61.4555616623674));
#221286=CARTESIAN_POINT('Ctrl Pts',(-30.4130225801109,74.3015905717297,
61.0083221897942));
#221287=CARTESIAN_POINT('Ctrl Pts',(-30.5106899664009,70.365103460175,61.9191332848712));
#221288=CARTESIAN_POINT('Ctrl Pts',(-30.6083573526909,66.9540024821432,
64.0847504597222));
#221289=CARTESIAN_POINT('Ctrl Pts',(-30.7060247389809,64.4549511021745,
67.2596913773823));
#221290=CARTESIAN_POINT('Ctrl Pts',(-30.8036921252709,63.1512279071195,
71.0840623663198));
#221291=CARTESIAN_POINT('Ctrl Pts',(-30.9013595115609,63.1906157186087,
75.1243539684998));
#221292=CARTESIAN_POINT('Ctrl Pts',(-30.9990268978509,64.5686497530634,
78.9225811642114));
#221293=CARTESIAN_POINT('Ctrl Pts',(-31.0966942841409,67.1291237247518,
82.0481980106354));
#221294=CARTESIAN_POINT('Ctrl Pts',(-31.1943616704309,70.5817965229168,
84.1469019390543));
#221295=CARTESIAN_POINT('Ctrl Pts',(-31.2920290567209,74.5352923323311,
84.980795526557));
#221296=CARTESIAN_POINT('Ctrl Pts',(-31.3896964430109,78.5414648223814,
84.4553532267351));
#221297=CARTESIAN_POINT('Ctrl Pts',(-31.4873638293009,82.1461965263699,
82.630136261015));
#221298=CARTESIAN_POINT('Ctrl Pts',(-31.5850312155909,84.9408750761412,
79.712041088333));
#221299=CARTESIAN_POINT('Ctrl Pts',(-31.6826986018809,86.6087112297139,
76.031846775141));
#221300=CARTESIAN_POINT('Ctrl Pts',(-31.7803659881709,86.9606483455424,
72.0067197036773));
#221301=CARTESIAN_POINT('Ctrl Pts',(-31.8780333744609,85.9567927749164,
68.0929259582372));
#221302=CARTESIAN_POINT('Ctrl Pts',(-31.9757007607509,83.7109360542007,
64.7341113461544));
#221303=CARTESIAN_POINT('Ctrl Pts',(-32.0733681470409,80.4776558675686,
62.3110128795057));
#221304=CARTESIAN_POINT('Ctrl Pts',(-32.1710355333309,76.6234595071886,
61.0982979039962));
#221305=CARTESIAN_POINT('Ctrl Pts',(-32.2687029196209,72.5852350114378,
61.233439177867));
#221306=CARTESIAN_POINT('Ctrl Pts',(-32.3663703059109,68.8207415117928,
62.7010949855073));
#221307=CARTESIAN_POINT('Ctrl Pts',(-32.4640376922009,65.7566696348843,
65.3349852966985));
#221308=CARTESIAN_POINT('Ctrl Pts',(-32.5291492830609,64.4125318335594,
67.6691475357373));
#221309=CARTESIAN_POINT('Ctrl Pts',(-32.5617050784909,63.9531251169506,
68.9148385500207));
#221310=CARTESIAN_POINT('',(-25.7929823067402,86.9560662404983,67.8848523453355));
#221311=CARTESIAN_POINT('Ctrl Pts',(-21.8528274563309,86.0743198651036,
79.922508163981));
#221312=CARTESIAN_POINT('Ctrl Pts',(-21.8943126079409,87.0706315571954,
78.331207182819));
#221313=CARTESIAN_POINT('Ctrl Pts',(-21.9772829111709,88.365914761124,74.7135063587071));
#221314=CARTESIAN_POINT('Ctrl Pts',(-22.1017383660109,87.8638206689949,
68.9705612798485));
#221315=CARTESIAN_POINT('Ctrl Pts',(-22.2261938208509,85.007906359249,63.9630709697879));
#221316=CARTESIAN_POINT('Ctrl Pts',(-22.3506492756909,80.3208945091187,
60.6069640495696));
#221317=CARTESIAN_POINT('Ctrl Pts',(-22.4751047305309,74.660314401302,59.516380349804));
#221318=CARTESIAN_POINT('Ctrl Pts',(-22.5995601853709,69.0618889064457,
60.8908421950948));
#221319=CARTESIAN_POINT('Ctrl Pts',(-22.7240156402109,64.5499522186845,
64.4788713483501));
#221320=CARTESIAN_POINT('Ctrl Pts',(-22.8484710950509,61.950049264097,69.6239686585277));
#221321=CARTESIAN_POINT('Ctrl Pts',(-22.9729265498909,61.737881126671,75.3847418289771));
#221322=CARTESIAN_POINT('Ctrl Pts',(-23.0973820047309,63.9522680392151,
80.7071485391446));
#221323=CARTESIAN_POINT('Ctrl Pts',(-23.2218374595709,68.1880460907971,
84.6173540230353));
#221324=CARTESIAN_POINT('Ctrl Pts',(-23.3462929144109,73.6701997203885,
86.3999123553094));
#221325=CARTESIAN_POINT('Ctrl Pts',(-23.4707483692509,79.3956654174182,
85.7286708365147));
#221326=CARTESIAN_POINT('Ctrl Pts',(-23.5952038240909,84.3168611364881,
82.726445774969));
#221327=CARTESIAN_POINT('Ctrl Pts',(-23.7196592789309,87.5333612087902,
77.9425509276693));
#221328=CARTESIAN_POINT('Ctrl Pts',(-23.8441147337709,88.4566462187817,
72.2522901765632));
#221329=CARTESIAN_POINT('Ctrl Pts',(-23.9685701886109,86.9177837423074,
66.6968041578818));
#221330=CARTESIAN_POINT('Ctrl Pts',(-24.0930256434509,83.1983377230885,
62.292573926019));
#221331=CARTESIAN_POINT('Ctrl Pts',(-24.2174810982909,77.9788510332431,
59.8454365534837));
#221332=CARTESIAN_POINT('Ctrl Pts',(-24.3419365531309,72.2143273064089,
59.8031420245331));
#221333=CARTESIAN_POINT('Ctrl Pts',(-24.4663920079709,66.959494991902,62.1734289212542));
#221334=CARTESIAN_POINT('Ctrl Pts',(-24.5908474628109,63.175824874085,66.522608506883));
#221335=CARTESIAN_POINT('Ctrl Pts',(-24.7153029176509,61.5556108309429,
72.0549162569263));
#221336=CARTESIAN_POINT('Ctrl Pts',(-24.8397583724909,62.3953016319811,
77.7581120451256));
#221337=CARTESIAN_POINT('Ctrl Pts',(-24.9642138273309,65.5412599143316,
82.5886884279321));
#221338=CARTESIAN_POINT('Ctrl Pts',(-25.0886692821709,70.417873503959,85.6628006211224));
#221339=CARTESIAN_POINT('Ctrl Pts',(-25.2131247370109,76.1328727949813,
86.4179803938818));
#221340=CARTESIAN_POINT('Ctrl Pts',(-25.3375801918409,81.6405947968609,
84.7160584470278));
#221341=CARTESIAN_POINT('Ctrl Pts',(-25.4620356466809,85.9332827488514,
80.8684145069104));
#221342=CARTESIAN_POINT('Ctrl Pts',(-25.5864911015209,88.2255644558482,
75.5791186817848));
#221343=CARTESIAN_POINT('Ctrl Pts',(-25.7109465563609,88.0978142907784,
69.8156825060805));
#221344=CARTESIAN_POINT('Ctrl Pts',(-25.7939168595909,86.4153968231172,
66.3609771213052));
#221345=CARTESIAN_POINT('Ctrl Pts',(-25.8354020112009,85.2513468075614,
64.8879315138231));
#221346=CARTESIAN_POINT('Ctrl Pts',(-22.0769555666009,85.7093978414631,
79.694030909732));
#221347=CARTESIAN_POINT('Ctrl Pts',(-22.1184407182209,86.672878977512,78.1551666272841));
#221348=CARTESIAN_POINT('Ctrl Pts',(-22.2014110214409,87.9254798881987,
74.6566766189857));
#221349=CARTESIAN_POINT('Ctrl Pts',(-22.3258664762809,87.4399308475407,
69.1029736033339));
#221350=CARTESIAN_POINT('Ctrl Pts',(-22.4503219311209,84.6781248931543,
64.2604905821707));
#221351=CARTESIAN_POINT('Ctrl Pts',(-22.5747773859609,80.1455598957456,
61.014974410985));
#221352=CARTESIAN_POINT('Ctrl Pts',(-22.6992328408009,74.6715077529058,
59.9603277272688));
#221353=CARTESIAN_POINT('Ctrl Pts',(-22.8236882956409,69.2575620984069,
61.2894981773207));
#221354=CARTESIAN_POINT('Ctrl Pts',(-22.9481437504809,64.8943031702593,
64.7592942584412));
#221355=CARTESIAN_POINT('Ctrl Pts',(-23.0725992053209,62.3800724609222,
69.7348498409865));
#221356=CARTESIAN_POINT('Ctrl Pts',(-23.1970546601609,62.1748957078033,
75.3057934752902));
#221357=CARTESIAN_POINT('Ctrl Pts',(-23.3215101150009,64.3163139357595,
80.4528157418881));
#221358=CARTESIAN_POINT('Ctrl Pts',(-23.4459655698409,68.4125142329405,
84.2341717690691));
#221359=CARTESIAN_POINT('Ctrl Pts',(-23.5704210246809,73.7140194235437,
85.9579910725118));
#221360=CARTESIAN_POINT('Ctrl Pts',(-23.6948764795209,79.2508190395935,
85.3088683670014));
#221361=CARTESIAN_POINT('Ctrl Pts',(-23.8193319343609,84.0098510571879,
82.4055729063877));
#221362=CARTESIAN_POINT('Ctrl Pts',(-23.9437873892009,87.1203607183689,
77.7793174093934));
#221363=CARTESIAN_POINT('Ctrl Pts',(-24.0682428440409,88.0132215543806,
72.2765626625984));
#221364=CARTESIAN_POINT('Ctrl Pts',(-24.1926982988809,86.5250678181105,
66.9041415386484));
#221365=CARTESIAN_POINT('Ctrl Pts',(-24.3171537537209,82.9281853318851,
62.6450399131802));
#221366=CARTESIAN_POINT('Ctrl Pts',(-24.4416092085609,77.8806916554658,
60.2785408401571));
#221367=CARTESIAN_POINT('Ctrl Pts',(-24.5660646634009,72.3061210534633,
60.2376400044814));
#221368=CARTESIAN_POINT('Ctrl Pts',(-24.6905201182409,67.2244464647128,
62.5298209857595));
#221369=CARTESIAN_POINT('Ctrl Pts',(-24.8149755730809,63.565456198401,66.7356859990377));
#221370=CARTESIAN_POINT('Ctrl Pts',(-24.9394310279209,61.9986315998985,
72.0856926268274));
#221371=CARTESIAN_POINT('Ctrl Pts',(-25.0638864827609,62.8106528311494,
77.6009561741625));
#221372=CARTESIAN_POINT('Ctrl Pts',(-25.1883419376009,65.8529452020323,
82.2723549523412));
#221373=CARTESIAN_POINT('Ctrl Pts',(-25.3127973924409,70.5688641646879,
85.2451687131141));
#221374=CARTESIAN_POINT('Ctrl Pts',(-25.4372528472809,76.0955422647207,
85.9754637313838));
#221375=CARTESIAN_POINT('Ctrl Pts',(-25.5617083021209,81.4217732962185,
84.3296236756516));
#221376=CARTESIAN_POINT('Ctrl Pts',(-25.6861637569609,85.5730081934492,
80.6087676584069));
#221377=CARTESIAN_POINT('Ctrl Pts',(-25.8106192118009,87.7897544193025,
75.4937652038599));
#221378=CARTESIAN_POINT('Ctrl Pts',(-25.9350746666409,87.6662138896252,
69.9202463159047));
#221379=CARTESIAN_POINT('Ctrl Pts',(-26.0180449698709,86.0392355996607,
66.5793807059785));
#221380=CARTESIAN_POINT('Ctrl Pts',(-26.0595301214809,84.9135434690527,
65.1548750350943));
#221381=CARTESIAN_POINT('Ctrl Pts',(-22.3010836768809,85.3444758178016,
79.4655536555077));
#221382=CARTESIAN_POINT('Ctrl Pts',(-22.3425688284909,86.2751263978158,
77.9791260717799));
#221383=CARTESIAN_POINT('Ctrl Pts',(-22.4255391317209,87.4850450152697,
74.5998468792995));
#221384=CARTESIAN_POINT('Ctrl Pts',(-22.5499945865609,87.0160410260944,
69.235385926855));
#221385=CARTESIAN_POINT('Ctrl Pts',(-22.6744500414009,84.3483434270861,
64.5579101945861));
#221386=CARTESIAN_POINT('Ctrl Pts',(-22.7989054962409,79.9702252824092,
61.4229847724263));
#221387=CARTESIAN_POINT('Ctrl Pts',(-22.9233609510809,74.6827011045569,
60.4042751047315));
#221388=CARTESIAN_POINT('Ctrl Pts',(-23.0478164059209,69.4532352904164,
61.6881541595265));
#221389=CARTESIAN_POINT('Ctrl Pts',(-23.1722718607609,65.238654121862,65.0397171684909));
#221390=CARTESIAN_POINT('Ctrl Pts',(-23.2967273156009,62.8100956577584,
69.8457310233925));
#221391=CARTESIAN_POINT('Ctrl Pts',(-23.4211827704409,62.6119102889162,
75.2268451215454));
#221392=CARTESIAN_POINT('Ctrl Pts',(-23.5456382252809,64.6803598322671,
80.1984829445947));
#221393=CARTESIAN_POINT('Ctrl Pts',(-23.6700936801209,68.6369823750294,
83.8509895150804));
#221394=CARTESIAN_POINT('Ctrl Pts',(-23.7945491349609,73.7578391266432,
85.516069789702));
#221395=CARTESIAN_POINT('Ctrl Pts',(-23.9190045898009,79.1059726617113,
84.8890658975066));
#221396=CARTESIAN_POINT('Ctrl Pts',(-24.0434600446409,83.7028409778482,
82.0847000378495));
#221397=CARTESIAN_POINT('Ctrl Pts',(-24.1679154994809,86.7073602279152,
77.6160838911697));
#221398=CARTESIAN_POINT('Ctrl Pts',(-24.2923709543209,87.5697968899769,
72.3008351486921));
#221399=CARTESIAN_POINT('Ctrl Pts',(-24.4168264091609,86.1323518939429,
67.1114789194617));
#221400=CARTESIAN_POINT('Ctrl Pts',(-24.5412818640009,82.6580329407277,
62.997505900382));
#221401=CARTESIAN_POINT('Ctrl Pts',(-24.6657373188409,77.7825322777459,
60.7116451268434));
#221402=CARTESIAN_POINT('Ctrl Pts',(-24.7901927736809,72.3979148005717,
60.6721379844194));
#221403=CARTESIAN_POINT('Ctrl Pts',(-24.9146482285209,67.4893979375692,
62.8862130502327));
#221404=CARTESIAN_POINT('Ctrl Pts',(-25.0391036833609,63.955087522728,66.9487634911397));
#221405=CARTESIAN_POINT('Ctrl Pts',(-25.1635591382009,62.4416523688531,
72.1164689966783));
#221406=CARTESIAN_POINT('Ctrl Pts',(-25.2880145930409,63.2260040303007,
77.4438003031568));
#221407=CARTESIAN_POINT('Ctrl Pts',(-25.4124700478809,66.1646304897018,
81.9560214767266));
#221408=CARTESIAN_POINT('Ctrl Pts',(-25.5369255027209,70.7198548253873,
84.8275368050829));
#221409=CARTESIAN_POINT('Ctrl Pts',(-25.6613809575609,76.0582117344314,
85.5329470688848));
#221410=CARTESIAN_POINT('Ctrl Pts',(-25.7858364124009,81.2029517955551,
83.9431889042895));
#221411=CARTESIAN_POINT('Ctrl Pts',(-25.9102918672409,85.2127336380402,
80.34912080992));
#221412=CARTESIAN_POINT('Ctrl Pts',(-26.0347473220809,87.3539443827526,
75.4084117259452));
#221413=CARTESIAN_POINT('Ctrl Pts',(-26.1592027769209,87.2346134884619,
70.024810125727));
#221414=CARTESIAN_POINT('Ctrl Pts',(-26.2421730801409,85.6630743761998,
66.7977842906575));
#221415=CARTESIAN_POINT('Ctrl Pts',(-26.2836582317609,84.5757401305432,
65.4218185563542));
#221416=CARTESIAN_POINT('Ctrl Pts',(-22.5252117871509,84.9795537941519,
79.2370764012549));
#221417=CARTESIAN_POINT('Ctrl Pts',(-22.5666969387709,85.8773738181418,
77.8030855162483));
#221418=CARTESIAN_POINT('Ctrl Pts',(-22.6496672419909,87.0446101423444,
74.5430171395781));
#221419=CARTESIAN_POINT('Ctrl Pts',(-22.7741226968309,86.5921512046365,
69.3677982503388));
#221420=CARTESIAN_POINT('Ctrl Pts',(-22.8985781516709,84.0185619609905,
64.8553298069685));
#221421=CARTESIAN_POINT('Ctrl Pts',(-23.0230336065109,79.7948906690355,
61.8309951338414));
#221422=CARTESIAN_POINT('Ctrl Pts',(-23.1474890613509,74.6938944561598,
60.8482224821959));
#221423=CARTESIAN_POINT('Ctrl Pts',(-23.2719445161909,69.6489084823822,
62.0868101417543));
#221424=CARTESIAN_POINT('Ctrl Pts',(-23.3963999710309,65.5830050734272,
65.3201400785792));
#221425=CARTESIAN_POINT('Ctrl Pts',(-23.5208554258709,63.2401188545836,
69.9566122058514));
#221426=CARTESIAN_POINT('Ctrl Pts',(-23.6453108807209,63.0489248700484,
75.1478967678585));
#221427=CARTESIAN_POINT('Ctrl Pts',(-23.7697663355609,65.0444057288086,
79.9441501473479));
#221428=CARTESIAN_POINT('Ctrl Pts',(-23.8942217904009,68.8614505171728,
83.4678072611142));
#221429=CARTESIAN_POINT('Ctrl Pts',(-24.0186772452409,73.8016588297993,
85.0741485069047));
#221430=CARTESIAN_POINT('Ctrl Pts',(-24.1431327000809,78.9611262838869,
84.4692634279924));
#221431=CARTESIAN_POINT('Ctrl Pts',(-24.2675881549209,83.3958308985575,
81.7638271692711));
#221432=CARTESIAN_POINT('Ctrl Pts',(-24.3920436097609,86.2943597374942,
77.4528503728929));
#221433=CARTESIAN_POINT('Ctrl Pts',(-24.5164990646009,87.1263722255761,
72.3251076347264));
#221434=CARTESIAN_POINT('Ctrl Pts',(-24.6409545194409,85.7396359697469,
67.3188163002233));
#221435=CARTESIAN_POINT('Ctrl Pts',(-24.7654099742709,82.3878805495234,
63.3499718875428));
#221436=CARTESIAN_POINT('Ctrl Pts',(-24.8898654291109,77.6843728999677,
61.1447494135163));
#221437=CARTESIAN_POINT('Ctrl Pts',(-25.0143208839509,72.489708547626,61.1066359643677));
#221438=CARTESIAN_POINT('Ctrl Pts',(-25.1387763387909,67.7543494103795,
63.2426051147388));
#221439=CARTESIAN_POINT('Ctrl Pts',(-25.2632317936309,64.344718847044,67.1618409832945));
#221440=CARTESIAN_POINT('Ctrl Pts',(-25.3876872484709,62.8846731378082,
72.1472453665802));
#221441=CARTESIAN_POINT('Ctrl Pts',(-25.5121427033109,63.6413552294693,
77.2866444321928));
#221442=CARTESIAN_POINT('Ctrl Pts',(-25.6365981581509,66.4763157774064,
81.6396880011265));
#221443=CARTESIAN_POINT('Ctrl Pts',(-25.7610536129909,70.8708454861167,
84.4099048970748));
#221444=CARTESIAN_POINT('Ctrl Pts',(-25.8855090678309,76.0208812041709,
85.0904304063868));
#221445=CARTESIAN_POINT('Ctrl Pts',(-26.0099645226709,80.9841302949145,
83.5567541329141));
#221446=CARTESIAN_POINT('Ctrl Pts',(-26.1344199775109,84.8524590826292,
80.0894739614117));
#221447=CARTESIAN_POINT('Ctrl Pts',(-26.2588754323509,86.9181343462161,
75.3230582480241));
#221448=CARTESIAN_POINT('Ctrl Pts',(-26.3833308871909,86.8030130873046,
70.1293739355507));
#221449=CARTESIAN_POINT('Ctrl Pts',(-26.4663011904209,85.2869131527418,
67.0161878753345));
#221450=CARTESIAN_POINT('Ctrl Pts',(-26.5077863420309,84.2379367920383,
65.6887620776161));
#221451=CARTESIAN_POINT('',(-22.5675364832709,86.9994393436682,73.0560055650937));
#221452=CARTESIAN_POINT('Ctrl Pts',(-22.5675364832709,86.9990620203006,
73.0559939530084));
#221453=CARTESIAN_POINT('Ctrl Pts',(-22.5675364832709,86.969760595878,73.6283224514649));
#221454=CARTESIAN_POINT('Ctrl Pts',(-22.5675364832698,86.8995247109982,
74.1992222599948));
#221455=CARTESIAN_POINT('Ctrl Pts',(-22.5675364832698,86.6763715914487,
75.321931358547));
#221456=CARTESIAN_POINT('Ctrl Pts',(-22.5675364832709,86.5248895569673,
75.8722213989229));
#221457=CARTESIAN_POINT('Ctrl Pts',(-22.5675364832709,86.3349224103826,
76.4088722773807));
#221458=CARTESIAN_POINT('Ctrl Pts',(-22.5673477912806,86.9996280326377,
73.0560066204832));
#221459=CARTESIAN_POINT('Ctrl Pts',(-22.5674106883502,86.999721811328,73.0504855961939));
#221460=CARTESIAN_POINT('Ctrl Pts',(-22.5674735854198,86.9998117796859,
73.0449644637686));
#221461=CARTESIAN_POINT('Ctrl Pts',(-22.5675364824894,86.9998979375059,
73.039443228467));
#221462=CARTESIAN_POINT('Origin',(-21.7675364832709,75.,72.9888893865801));
#221463=CARTESIAN_POINT('',(-23.0675424572509,84.7043582237312,76.9983072327893));
#221464=CARTESIAN_POINT('',(-23.0675424572509,65.2956417762688,68.9794715403709));
#221465=CARTESIAN_POINT('Origin',(-23.0675424572509,75.,72.9888893865801));
#221466=CARTESIAN_POINT('',(-38.5675364832709,84.7043582237312,76.9983072327893));
#221467=CARTESIAN_POINT('',(-21.7675364832709,84.7043582237312,76.9983072327893));
#221468=CARTESIAN_POINT('Origin',(-38.5675364832709,75.,72.9888893865801));
#221469=CARTESIAN_POINT('Origin',(-23.0675424572509,75.,72.9888893865801));
#221470=CARTESIAN_POINT('Origin',(-22.8175393993109,75.,72.9888893865801));
#221471=CARTESIAN_POINT('',(-22.5675364832709,64.8335236965284,68.7885444915902));
#221472=CARTESIAN_POINT('',(-22.8175393993109,65.0645826708248,68.8840079888883));
#221473=CARTESIAN_POINT('Origin',(-22.5675364832709,75.,72.9888893865801));
#221474=CARTESIAN_POINT('Origin',(-22.5675364832709,75.,72.9888893865801));
#221475=CARTESIAN_POINT('Origin',(-38.5675364832709,75.,72.9888893865801));
#221476=CARTESIAN_POINT('Origin',(-48.5675364832709,66.6819786653733,69.5522455184007));
#221477=CARTESIAN_POINT('',(-48.5675364832709,73.8447192590797,72.5115777382218));
#221478=CARTESIAN_POINT('Origin',(-48.5675364832709,66.6819786653733,69.5522455184007));
#221479=CARTESIAN_POINT('Origin',(-47.7675364832709,66.6819786653733,69.5522455184007));
#221480=CARTESIAN_POINT('',(-64.0675410045048,73.8447192590797,72.5115777382218));
#221481=CARTESIAN_POINT('',(-47.7675364832709,73.8447192590797,72.5115777382218));
#221482=CARTESIAN_POINT('Origin',(-64.0675410045048,66.6819786653733,69.5522455184007));
#221483=CARTESIAN_POINT('Origin',(-64.3175392245649,66.6819786653733,69.5522455184007));
#221484=CARTESIAN_POINT('',(-64.5675367041793,74.3068269192978,72.70250048211));
#221485=CARTESIAN_POINT('',(-64.3175392245649,74.075773247593,72.6070391756116));
#221486=CARTESIAN_POINT('Origin',(-64.5675367039552,66.6819786653733,69.5522455184007));
#221487=CARTESIAN_POINT('Origin',(-64.5675364832709,66.6819786653733,69.5522455184007));
#221488=CARTESIAN_POINT('Ctrl Pts',(-64.5675364832709,57.6609583680643,
70.6705889999386));
#221489=CARTESIAN_POINT('Ctrl Pts',(-64.5675364832709,57.6884511920649,
71.1096763190363));
#221490=CARTESIAN_POINT('Ctrl Pts',(-64.5675364832708,57.7483094871617,
71.5466701563318));
#221491=CARTESIAN_POINT('Ctrl Pts',(-64.5675364832708,57.9303798077129,
72.41066731052));
#221492=CARTESIAN_POINT('Ctrl Pts',(-64.5675364832709,58.0530241033855,
72.8375946044308));
#221493=CARTESIAN_POINT('Ctrl Pts',(-64.5675364832709,58.2054611415104,
73.2535681280901));
#221494=CARTESIAN_POINT('Origin',(-45.8894114130409,66.6819786653733,69.5522455184007));
#221495=CARTESIAN_POINT('',(-63.5674079539854,63.4392572871834,59.8285649416409));
#221496=CARTESIAN_POINT('Ctrl Pts',(-63.567539947994,63.4350769493012,59.8300991896842));
#221497=CARTESIAN_POINT('Ctrl Pts',(-63.5674959499171,63.4364702751625,
59.8295874742253));
#221498=CARTESIAN_POINT('Ctrl Pts',(-63.5674519518401,63.4378637211896,
59.8290760582624));
#221499=CARTESIAN_POINT('Ctrl Pts',(-63.5674079537632,63.4392572872537,
59.8285649418516));
#221500=CARTESIAN_POINT('',(-62.9075072593131,76.1552860519195,73.46618818022));
#221501=CARTESIAN_POINT('Ctrl Pts',(-63.5674123768639,63.4393239295404,
59.8286818576752));
#221502=CARTESIAN_POINT('Ctrl Pts',(-63.5537244696136,63.8950358571431,
59.6767091353507));
#221503=CARTESIAN_POINT('Ctrl Pts',(-63.5400136073417,64.3608717030263,
59.5569597714857));
#221504=CARTESIAN_POINT('Ctrl Pts',(-63.5129296748257,65.3050981973121,
59.3838289856031));
#221505=CARTESIAN_POINT('Ctrl Pts',(-63.4995889539748,65.7823014895405,
59.330549021255));
#221506=CARTESIAN_POINT('Ctrl Pts',(-63.4597780386861,67.2123915236249,
59.2718310830067));
#221507=CARTESIAN_POINT('Ctrl Pts',(-63.4325802602361,68.1641190178407,
59.3654163782555));
#221508=CARTESIAN_POINT('Ctrl Pts',(-63.3869424607676,69.7331885825598,
59.744516418622));
#221509=CARTESIAN_POINT('Ctrl Pts',(-63.3686283032081,70.3605758197365,
59.9621800299818));
#221510=CARTESIAN_POINT('Ctrl Pts',(-63.3128692356676,72.1773044290275,
60.7971770385974));
#221511=CARTESIAN_POINT('Ctrl Pts',(-63.2745815754463,73.2711609789934,
61.587793568521));
#221512=CARTESIAN_POINT('Ctrl Pts',(-63.2002097006855,75.093653850845,63.5444294238347));
#221513=CARTESIAN_POINT('Ctrl Pts',(-63.1618824850836,75.8047677283667,
64.6917037744082));
#221514=CARTESIAN_POINT('Ctrl Pts',(-63.1061663303517,76.5088612625986,
66.563278327776));
#221515=CARTESIAN_POINT('Ctrl Pts',(-63.0878060649445,76.6814853170575,
67.2046067609666));
#221516=CARTESIAN_POINT('Ctrl Pts',(-63.0553782680594,76.8696372913774,
68.3273127282598));
#221517=CARTESIAN_POINT('Ctrl Pts',(-63.0417928519769,76.9155090722919,
68.8014397964858));
#221518=CARTESIAN_POINT('Ctrl Pts',(-63.0081560309446,76.9474973885907,
69.9923893239148));
#221519=CARTESIAN_POINT('Ctrl Pts',(-62.9884692522367,76.8917445355874,
70.7077860596408));
#221520=CARTESIAN_POINT('Ctrl Pts',(-62.9483777816462,76.6320462074141,
72.1157259528595));
#221521=CARTESIAN_POINT('Ctrl Pts',(-62.9277656193976,76.4287171030932,
72.8043756242868));
#221522=CARTESIAN_POINT('Ctrl Pts',(-62.9075072593131,76.1552860519195,
73.46618818022));
#221523=CARTESIAN_POINT('Ctrl Pts',(-62.9075072593131,76.1552860519195,
73.46618818022));
#221524=CARTESIAN_POINT('Ctrl Pts',(-62.9075071281503,76.1552842815894,
73.4661924651273));
#221525=CARTESIAN_POINT('Ctrl Pts',(-62.9075069969875,76.1552825112564,
73.4661967500333));
#221526=CARTESIAN_POINT('Ctrl Pts',(-62.9075068658247,76.1552807409205,
73.4662010349381));
#221527=CARTESIAN_POINT('Ctrl Pts',(-64.7235137149846,58.9641128133577,
74.2288240611484));
#221528=CARTESIAN_POINT('Ctrl Pts',(-64.6818903153503,58.2898823562254,
73.1161259264028));
#221529=CARTESIAN_POINT('Ctrl Pts',(-64.5986435160818,57.4306928818431,
70.5953071644979));
#221530=CARTESIAN_POINT('Ctrl Pts',(-64.4737733171789,57.8453681147118,
66.6213799744606));
#221531=CARTESIAN_POINT('Ctrl Pts',(-64.3489031182761,59.8875902288061,
63.1873940424807));
#221532=CARTESIAN_POINT('Ctrl Pts',(-64.2240329193733,63.1811176368601,
60.9255881378499));
#221533=CARTESIAN_POINT('Ctrl Pts',(-64.0991627204705,67.1194100886389,
60.2525763176752));
#221534=CARTESIAN_POINT('Ctrl Pts',(-63.9742925215677,70.9771383669053,
61.2922934738364));
#221535=CARTESIAN_POINT('Ctrl Pts',(-63.8494223226649,74.0438220518638,
63.8532574547353));
#221536=CARTESIAN_POINT('Ctrl Pts',(-63.7245521237622,75.7546654243016,
67.4638112038693));
#221537=CARTESIAN_POINT('Ctrl Pts',(-63.5996819248594,75.7945804349819,
71.4589945804267));
#221538=CARTESIAN_POINT('Ctrl Pts',(-63.4748117259569,74.1562158093098,
75.103009768157));
#221539=CARTESIAN_POINT('Ctrl Pts',(-63.3499415270539,71.1413113950972,
77.7247325999806));
#221540=CARTESIAN_POINT('Ctrl Pts',(-63.2250713281509,67.305125597119,78.8413215436999));
#221541=CARTESIAN_POINT('Ctrl Pts',(-63.1002011292489,63.3541752639937,
78.2471160211359));
#221542=CARTESIAN_POINT('Ctrl Pts',(-62.9753309303459,60.0161061500815,
76.0516149086199));
#221543=CARTESIAN_POINT('Ctrl Pts',(-62.8504607314429,57.9057165985323,
72.6589303077136));
#221544=CARTESIAN_POINT('Ctrl Pts',(-62.7672139321749,57.5763043356606,
70.0161625645473));
#221545=CARTESIAN_POINT('Ctrl Pts',(-62.7255905325409,57.6961945356714,
68.7206664478601));
#221546=CARTESIAN_POINT('Ctrl Pts',(-64.4993856047086,58.5958913594194,
74.4519448802346));
#221547=CARTESIAN_POINT('Ctrl Pts',(-64.4577622050742,57.8894931859754,
73.2861596184455));
#221548=CARTESIAN_POINT('Ctrl Pts',(-64.3745154058057,56.9893115508722,
70.6450719159537));
#221549=CARTESIAN_POINT('Ctrl Pts',(-64.2496452069029,57.4237710505392,
66.4815475917032));
#221550=CARTESIAN_POINT('Ctrl Pts',(-64.1247750080001,59.5634281305272,
62.8837252680371));
#221551=CARTESIAN_POINT('Ctrl Pts',(-63.9999048090973,63.0140906163541,
60.5140079958519));
#221552=CARTESIAN_POINT('Ctrl Pts',(-63.8750346101945,67.1402800594054,
59.8088866008654));
#221553=CARTESIAN_POINT('Ctrl Pts',(-63.7501644112917,71.1820615905698,
60.8982089419637));
#221554=CARTESIAN_POINT('Ctrl Pts',(-63.6252942123889,74.395057578295,63.58135720264));
#221555=CARTESIAN_POINT('Ctrl Pts',(-63.5004240134859,76.1875257478145,
67.3641714414642));
#221556=CARTESIAN_POINT('Ctrl Pts',(-63.3755538145829,76.2293451143814,
71.5499660906056));
#221557=CARTESIAN_POINT('Ctrl Pts',(-63.2506836156809,74.5128136721155,
75.3678382222558));
#221558=CARTESIAN_POINT('Ctrl Pts',(-63.1258134167779,71.3540673580585,
78.1146441549625));
#221559=CARTESIAN_POINT('Ctrl Pts',(-63.0009432178749,67.3348561047015,
79.2845058572659));
#221560=CARTESIAN_POINT('Ctrl Pts',(-62.8760730189729,63.1954048693821,
78.6619506295289));
#221561=CARTESIAN_POINT('Ctrl Pts',(-62.7512028200699,59.6980755809505,
76.3617015689027));
#221562=CARTESIAN_POINT('Ctrl Pts',(-62.6263326211669,57.4869987767368,
72.8071510739182));
#221563=CARTESIAN_POINT('Ctrl Pts',(-62.5430858218989,57.1418701662744,
70.0382961714914));
#221564=CARTESIAN_POINT('Ctrl Pts',(-62.5014624222649,57.2674803599551,
68.6809915869218));
#221565=CARTESIAN_POINT('Ctrl Pts',(-64.2752574944325,58.2276699054746,
74.6750656993105));
#221566=CARTESIAN_POINT('Ctrl Pts',(-64.2336340947982,57.4891040157201,
73.4561933104751));
#221567=CARTESIAN_POINT('Ctrl Pts',(-64.1503872955297,56.5479302198967,
70.6948366673945));
#221568=CARTESIAN_POINT('Ctrl Pts',(-64.0255170966268,57.0021739863718,
66.341715208933));
#221569=CARTESIAN_POINT('Ctrl Pts',(-63.900646897724,59.2392660322718,62.5800564935892));
#221570=CARTESIAN_POINT('Ctrl Pts',(-63.7757766988212,62.8470635958519,
60.1024278538446));
#221571=CARTESIAN_POINT('Ctrl Pts',(-63.6509064999184,67.161150030173,59.3651968840528));
#221572=CARTESIAN_POINT('Ctrl Pts',(-63.5260363010159,71.3869848142425,
60.5041244100999));
#221573=CARTESIAN_POINT('Ctrl Pts',(-63.4011661021129,74.7462931047338,
63.3094569505521));
#221574=CARTESIAN_POINT('Ctrl Pts',(-63.2762959032099,76.6203860713289,
67.2645316790695));
#221575=CARTESIAN_POINT('Ctrl Pts',(-63.1514257043069,76.6641097937791,
71.6409376007935));
#221576=CARTESIAN_POINT('Ctrl Pts',(-63.0265555054049,74.8694115349166,
75.6326666763602));
#221577=CARTESIAN_POINT('Ctrl Pts',(-62.9016853065019,71.5668233210142,
78.5045557099475));
#221578=CARTESIAN_POINT('Ctrl Pts',(-62.7768151075989,67.3645866122776,
79.7276901708313));
#221579=CARTESIAN_POINT('Ctrl Pts',(-62.6519449086969,63.0366344747639,
79.0767852379246));
#221580=CARTESIAN_POINT('Ctrl Pts',(-62.5270747097939,59.3800450118199,
76.6717882291846));
#221581=CARTESIAN_POINT('Ctrl Pts',(-62.4022045108909,57.0682809549513,
72.9553718401247));
#221582=CARTESIAN_POINT('Ctrl Pts',(-62.3189577116229,56.707435996897,70.0604297784402));
#221583=CARTESIAN_POINT('Ctrl Pts',(-62.2773343119879,56.8387661842384,
68.6413167259844));
#221584=CARTESIAN_POINT('Ctrl Pts',(-64.0511293841564,57.8594484515271,
74.8981865183928));
#221585=CARTESIAN_POINT('Ctrl Pts',(-64.0095059845222,57.088714845479,73.6262270025225));
#221586=CARTESIAN_POINT('Ctrl Pts',(-63.9262591852536,56.1065488889258,
70.7446014188502));
#221587=CARTESIAN_POINT('Ctrl Pts',(-63.8013889863508,56.5805769221993,
66.2018828261753));
#221588=CARTESIAN_POINT('Ctrl Pts',(-63.676518787448,58.9151039339933,62.2763877191448));
#221589=CARTESIAN_POINT('Ctrl Pts',(-63.5516485885449,62.680036575337,59.6908477118419));
#221590=CARTESIAN_POINT('Ctrl Pts',(-63.4267783896419,67.182020000941,58.9215071672393));
#221591=CARTESIAN_POINT('Ctrl Pts',(-63.3019081907399,71.5919080379106,
60.1100398782212));
#221592=CARTESIAN_POINT('Ctrl Pts',(-63.1770379918369,75.0975286311649,
63.0375566984567));
#221593=CARTESIAN_POINT('Ctrl Pts',(-63.0521677929339,77.0532463948415,
67.1648919166655));
#221594=CARTESIAN_POINT('Ctrl Pts',(-62.9272975940309,77.0988744731788,
71.7319091109725));
#221595=CARTESIAN_POINT('Ctrl Pts',(-62.8024273951289,75.2260093977218,
75.8974951304588));
#221596=CARTESIAN_POINT('Ctrl Pts',(-62.6775571962259,71.7795792839757,
78.8944672649294));
#221597=CARTESIAN_POINT('Ctrl Pts',(-62.5526869973229,67.3943171198596,
80.170874484396));
#221598=CARTESIAN_POINT('Ctrl Pts',(-62.4278167984199,62.8778640801542,
79.491619846313));
#221599=CARTESIAN_POINT('Ctrl Pts',(-62.3029465995179,59.0620144426885,
76.9818748894683));
#221600=CARTESIAN_POINT('Ctrl Pts',(-62.1780764006149,56.6495631331558,
73.1035926063292));
#221601=CARTESIAN_POINT('Ctrl Pts',(-62.0948296013469,56.2730018275201,
70.0825633853882));
#221602=CARTESIAN_POINT('Ctrl Pts',(-62.0532062017119,56.410052008522,68.6016418650461));
#221603=CARTESIAN_POINT('Origin',(-113.778845940191,66.6819786653733,69.5522455184007));
#221604=CARTESIAN_POINT('',(-47.1840596451118,61.3985627647214,74.6727879441187));
#221605=CARTESIAN_POINT('Ctrl Pts',(-47.1840596451125,61.3985627647224,
74.6727879441184));
#221606=CARTESIAN_POINT('Ctrl Pts',(-47.1330608433754,61.0554912975567,
73.6555434581613));
#221607=CARTESIAN_POINT('Ctrl Pts',(-47.0897582262311,60.8615439161923,
72.5407972914318));
#221608=CARTESIAN_POINT('Ctrl Pts',(-47.0209270037,60.8476294176321,70.0468757692862));
#221609=CARTESIAN_POINT('Ctrl Pts',(-47.002286125824,61.1325740255311,68.6660964641816));
#221610=CARTESIAN_POINT('Ctrl Pts',(-47.002286125824,62.1277464170818,66.2573903246842));
#221611=CARTESIAN_POINT('Ctrl Pts',(-47.021100980925,62.9050951362454,65.0734714286778));
#221612=CARTESIAN_POINT('Ctrl Pts',(-47.0902140976192,64.6780140493426,
63.3201249465718));
#221613=CARTESIAN_POINT('Ctrl Pts',(-47.1333057957547,65.5971180331206,
62.671905978486));
#221614=CARTESIAN_POINT('Ctrl Pts',(-47.1840596451125,66.5535285669908,
62.1957559421795));
#221615=CARTESIAN_POINT('Origin',(-113.778845940191,64.1044957642388,75.7907615193708));
#221616=CARTESIAN_POINT('Origin',(-113.778845940191,66.6819786653733,69.5522455184007));
#221617=CARTESIAN_POINT('Origin',(-51.8559251551109,68.8530468966737,77.752655878079));
#221618=CARTESIAN_POINT('',(-47.1840596451109,61.3985627647217,74.6727879441188));
#221619=CARTESIAN_POINT('Origin',(-51.5615184913109,70.415046688923,71.0945865171214));
#221646=UNCERTAINTY_MEASURE_WITH_UNIT(LENGTH_MEASURE(0.01),#221663,
'DISTANCE_ACCURACY_VALUE',
'Maximum model space distance between geometric entities at asserted c
onnectivities');
#221647=UNCERTAINTY_MEASURE_WITH_UNIT(LENGTH_MEASURE(0.01),#221663,
'DISTANCE_ACCURACY_VALUE',
'Maximum model space distance between geometric entities at asserted c
onnectivities');
#221661=(
GEOMETRIC_REPRESENTATION_CONTEXT(3)
GLOBAL_UNCERTAINTY_ASSIGNED_CONTEXT((#221646))
GLOBAL_UNIT_ASSIGNED_CONTEXT((#221663,#221665,#221666))
REPRESENTATION_CONTEXT('','3D')
);
#221662=(
GEOMETRIC_REPRESENTATION_CONTEXT(3)
GLOBAL_UNCERTAINTY_ASSIGNED_CONTEXT((#221647))
GLOBAL_UNIT_ASSIGNED_CONTEXT((#221663,#221665,#221666))
REPRESENTATION_CONTEXT('','3D')
);
#221663=(
LENGTH_UNIT()
NAMED_UNIT(*)
SI_UNIT(.MILLI.,.METRE.)
);
#221665=(
NAMED_UNIT(*)
PLANE_ANGLE_UNIT()
SI_UNIT($,.RADIAN.)
);
#221666=(
NAMED_UNIT(*)
SI_UNIT($,.STERADIAN.)
SOLID_ANGLE_UNIT()
);
#221680=SHAPE_DEFINITION_REPRESENTATION(#221694,#221721);
#221694=PRODUCT_DEFINITION_SHAPE('',$,#221736);
#221721=SHAPE_REPRESENTATION('',(#86059),#221661);
#221722=PRODUCT_DEFINITION_CONTEXT('part definition',#221766,'design');
#221736=PRODUCT_DEFINITION('2026-10-05-23-03-42-219',
'Eccentric Connector',#221750,#221722);
#221750=PRODUCT_DEFINITION_FORMATION('',$,#221781);
#221766=APPLICATION_CONTEXT(
'Core Data for Automotive Mechanical Design Process');
#221767=PRODUCT_CONTEXT('part definition',#221766,'mechanical');
#221781=PRODUCT('2026-10-05-23-03-42-219','Eccentric Connector',$,(#221767));
#221783=PRESENTATION_STYLE_ASSIGNMENT((#221785));
#221785=SURFACE_STYLE_USAGE(.BOTH.,#221787);
#221787=SURFACE_SIDE_STYLE('',(#221789));
#221789=SURFACE_STYLE_FILL_AREA(#221791);
#221791=FILL_AREA_STYLE('Opaque(202,209,238)',(#221793));
#221793=FILL_AREA_STYLE_COLOUR('Opaque(202,209,238)',#221795);
#221795=COLOUR_RGB('Opaque(202,209,238)', 0.09019608, 0.27058824, 0.51372549);
ENDSEC;
END-ISO-10303-21;
